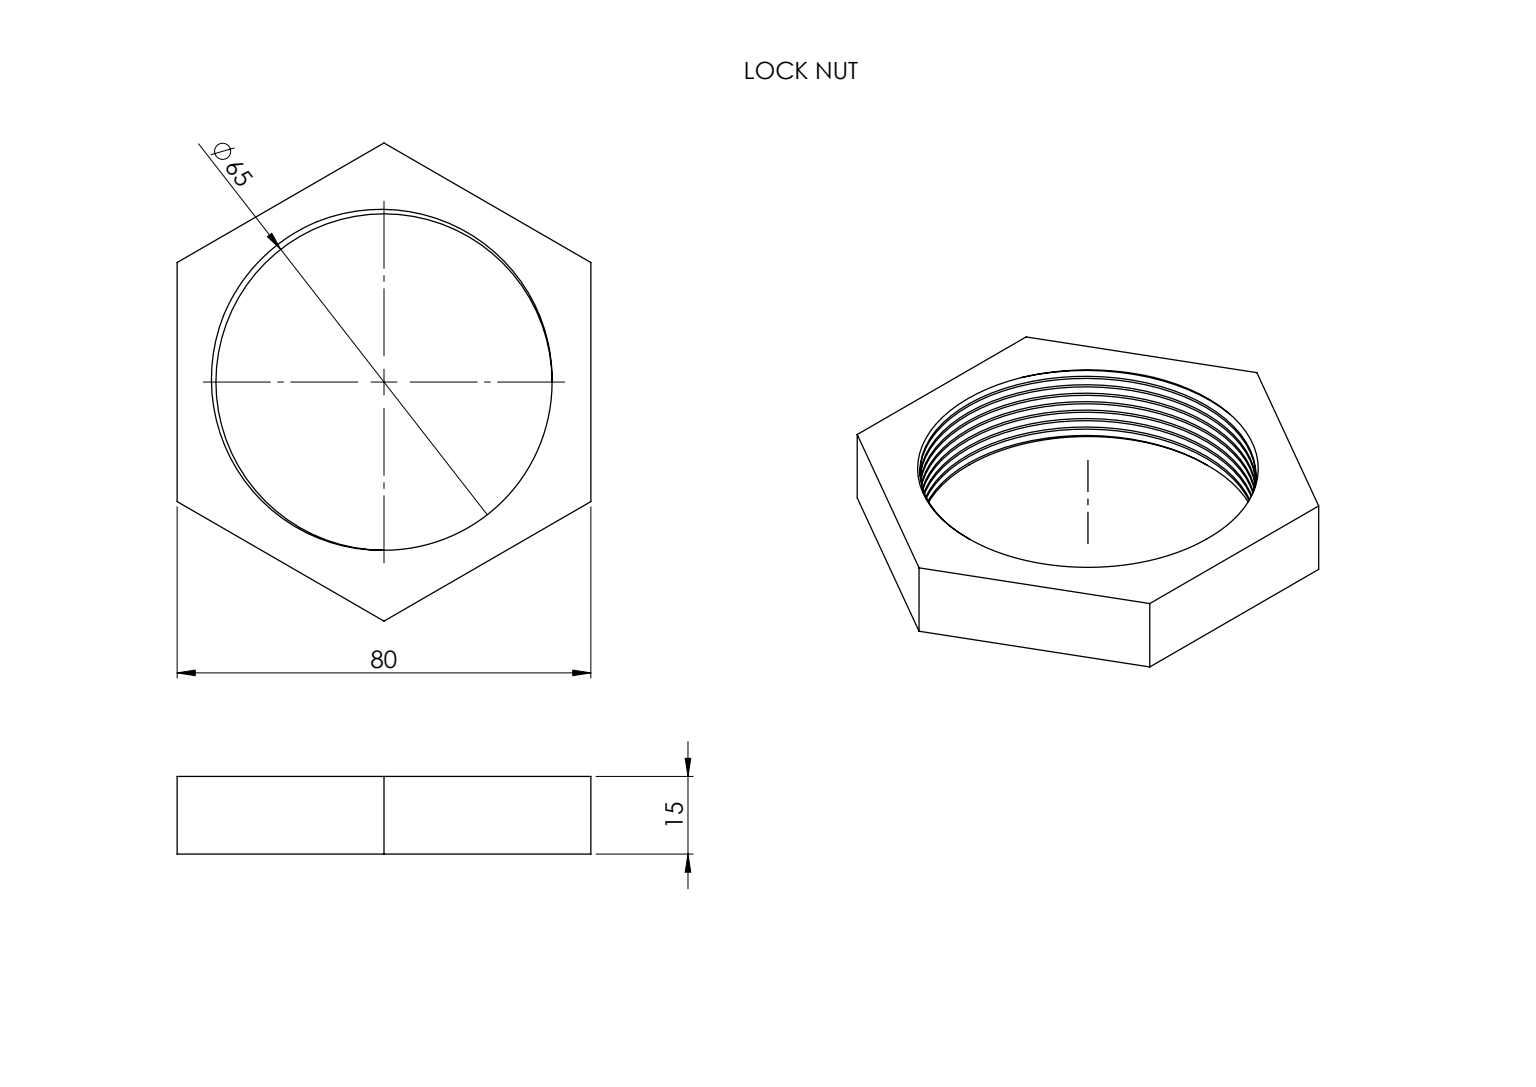
ISO-10303-21;
HEADER;
FILE_DESCRIPTION (('STEP AP214'),
    '1' );
FILE_NAME ('lock nut.step',
    '2026-10-02T18:08:48',
    ( '' ),
    ( '' ),
    'SwSTEP 2.0',
    'SolidWorks 2026',
    '' );
FILE_SCHEMA (( 'AUTOMOTIVE_DESIGN' ));
ENDSEC;

DATA;
#2=CARTESIAN_POINT ( 'NONE',  ( 20.75514604977249178, 32.07500000273117990, 28.56700777964553950 ) ) ;
#7=CARTESIAN_POINT ( 'NONE',  ( -32.50000000000000000, 22.50000000546238610, 0.000000000000000000 ) ) ;
#19=CARTESIAN_POINT ( 'NONE',  ( 10.37757302488624767, 61.72500000273119269, 31.93888565452638417 ) ) ;
#24=CARTESIAN_POINT ( 'NONE',  ( -10.04305231718579172, 66.10000000546239107, -30.90933677959248982 ) ) ;
#26=LINE ( 'NONE', #5703, #33612 ) ;
#29=CARTESIAN_POINT ( 'NONE',  ( 20.75514604977249178, 76.07500000273118701, 28.56700777964553950 ) ) ;
#34=CARTESIAN_POINT ( 'NONE',  ( 20.75514604977248467, 54.42500000273117422, -28.56700777964554305 ) ) ;
#35=CARTESIAN_POINT ( 'NONE',  ( 33.58253175000000113, 14.37500000273118950, -4.112674001490185761E-15 ) ) ;
#36=CARTESIAN_POINT ( 'NONE',  ( 10.37757302488624056, 4.775000002731191628, -31.93888565452638417 ) ) ;
#40=CARTESIAN_POINT ( 'NONE',  ( -26.29305231718578995, 76.70000000546238539, 19.10302069950538595 ) ) ;
#42=CARTESIAN_POINT ( 'NONE',  ( 1.353501352685244852, 52.00000000000004263, -32.52334280248234677 ) ) ;
#47=ORIENTED_EDGE ( 'NONE', *, *, #4310, .T. ) ;
#48=CARTESIAN_POINT ( 'NONE',  ( -33.58253175000000113, 53.27500000273117564, -10.91162601494193218 ) ) ;
#52=VERTEX_POINT ( 'NONE', #19751 ) ;
#53=CARTESIAN_POINT ( 'NONE',  ( -10.37757302488624411, 22.72500000273118559, -31.93888565452638417 ) ) ;
#64=B_SPLINE_CURVE_WITH_KNOTS ( 'NONE', 3,
 ( #12577, #7079, #6739, #22702, #12751, #9302, #25452, #17563, #30235, #33154 ),
 .UNSPECIFIED., .F., .F.,
 ( 4, 2, 2, 2, 4 ),
 ( 0.000000000000000000, 0.006590582801587737370, 0.01318116560317547474, 0.01977174840476321124, 0.02636233120635094948 ),
 .UNSPECIFIED. ) ;
#66=CARTESIAN_POINT ( 'NONE',  ( 1.093617666956751375E-13, 66.00000000546238255, -32.50000000000000711 ) ) ;
#68=CARTESIAN_POINT ( 'NONE',  ( -10.04305231718579172, 13.59999999999998721, -30.90933677959248982 ) ) ;
#74=CARTESIAN_POINT ( 'NONE',  ( -27.16883889988624290, 70.92500000273120975, -19.73931689729374028 ) ) ;
#76=CARTESIAN_POINT ( 'NONE',  ( -33.58253175000000113, 33.37500000273117706, 0.000000000000000000 ) ) ;
#83=CARTESIAN_POINT ( 'NONE',  ( -20.08610463437157989, 55.69999999999998863, -27.64615127144129758 ) ) ;
#88=CARTESIAN_POINT ( 'NONE',  ( 10.37757302488624767, 71.97500000273120691, 31.93888565452638417 ) ) ;
#93=CARTESIAN_POINT ( 'NONE',  ( 6.486482029760649416E-15, 43.62500000273116285, 35.31076352940723240 ) ) ;
#97=CARTESIAN_POINT ( 'NONE',  ( -20.08610463437157989, 4.200000005462371178, -27.64615127144129758 ) ) ;
#113=CARTESIAN_POINT ( 'NONE',  ( 27.16883889988623935, 52.57500000273117280, -19.73931689729374384 ) ) ;
#120=CARTESIAN_POINT ( 'NONE',  ( 6.486482029760649416E-15, 15.62500000273117884, 35.31076352940723240 ) ) ;
#126=CARTESIAN_POINT ( 'NONE',  ( 20.08610463437157279, 33.80000000546235839, -27.64615127144129758 ) ) ;
#131=CARTESIAN_POINT ( 'NONE',  ( -33.58253175000000113, 63.02500000273118985, -10.91162601494193218 ) ) ;
#133=ORIENTED_EDGE ( 'NONE', *, *, #14029, .F. ) ;
#137=CARTESIAN_POINT ( 'NONE',  ( -20.75514604977248112, 3.425000002731186655, 28.56700777964554661 ) ) ;
#147=CARTESIAN_POINT ( 'NONE',  ( 6.277390505771533514E-15, 20.49999999999999289, 34.17252228774368916 ) ) ;
#157=CARTESIAN_POINT ( 'NONE',  ( -6.410174973103736740, 66.99999999999995737, -32.88179426022560392 ) ) ;
#160=CARTESIAN_POINT ( 'NONE',  ( -33.58253175000000113, 33.02500000273118275, -10.91162601494193218 ) ) ;
#162=CARTESIAN_POINT ( 'NONE',  ( 12.90513655866702081, 52.00000000000000711, 31.00393344628893288 ) ) ;
#165=CARTESIAN_POINT ( 'NONE',  ( 20.08610463437158344, 53.20000000546237118, 27.64615127144129403 ) ) ;
#172=CARTESIAN_POINT ( 'NONE',  ( 10.37757302488624767, 25.97500000273118914, 31.93888565452638417 ) ) ;
#176=CARTESIAN_POINT ( 'NONE',  ( -20.08610463437156923, 14.80000000546238503, 27.64615127144130113 ) ) ;
#188=CARTESIAN_POINT ( 'NONE',  ( 10.37757302488624056, 60.52500000273118275, -31.93888565452638417 ) ) ;
#198=CARTESIAN_POINT ( 'NONE',  ( -33.58253175000000113, 73.27500000273118985, -10.91162601494193218 ) ) ;
#202=CARTESIAN_POINT ( 'NONE',  ( 27.16883889988623935, 52.32500000273120122, -19.73931689729374384 ) ) ;
#203=CARTESIAN_POINT ( 'NONE',  ( 33.58253175000000113, 16.37500000273119127, -4.112674001490185761E-15 ) ) ;
#204=CARTESIAN_POINT ( 'NONE',  ( 33.58253175000000113, 6.475000002731178483, -10.91162601494193751 ) ) ;
#208=CARTESIAN_POINT ( 'NONE',  ( -26.29305231718579350, 76.30000000546237970, -19.10302069950537884 ) ) ;
#209=CARTESIAN_POINT ( 'NONE',  ( 33.29860495311163504, 51.99999999999997868, -1.751800823569056309 ) ) ;
#217=CARTESIAN_POINT ( 'NONE',  ( 27.16883889988623935, 46.57500000273119412, -19.73931689729374384 ) ) ;
#221=CARTESIAN_POINT ( 'NONE',  ( -33.58253175000000113, 25.22500000273119625, 10.91162601494193929 ) ) ;
#225=FACE_OUTER_BOUND ( 'NONE', #13152, .T. ) ;
#240=CARTESIAN_POINT ( 'NONE',  ( 32.50000000000000000, 19.00000000000000355, -3.980102097228898626E-15 ) ) ;
#247=CARTESIAN_POINT ( 'NONE',  ( 33.58253175000000113, 76.12500000273118417, -4.112674001490185761E-15 ) ) ;
#248=CARTESIAN_POINT ( 'NONE',  ( 27.16883889988623935, 38.57500000273118701, -19.73931689729374384 ) ) ;
#254=CARTESIAN_POINT ( 'NONE',  ( -10.04305231718578462, 56.39999999999999147, 30.90933677959249337 ) ) ;
#258=ORIENTED_EDGE ( 'NONE', *, *, #24258, .F. ) ;
#259=CARTESIAN_POINT ( 'NONE',  ( 10.37757302488624056, 70.77500000273118985, -31.93888565452638417 ) ) ;
#264=CARTESIAN_POINT ( 'NONE',  ( 10.37757302488624767, 45.72500000273120691, 31.93888565452638417 ) ) ;
#269=CARTESIAN_POINT ( 'NONE',  ( 10.04305231718578817, 5.900000005462382902, -30.90933677959249337 ) ) ;
#288=CARTESIAN_POINT ( 'NONE',  ( 27.16883889988623935, 56.57500000273117990, -19.73931689729374384 ) ) ;
#295=CARTESIAN_POINT ( 'NONE',  ( -26.29305231718578995, 76.20000000000000284, 19.10302069950538595 ) ) ;
#296=CARTESIAN_POINT ( 'NONE',  ( -33.58253175000000113, 15.22500000273119447, 10.91162601494193929 ) ) ;
#300=CARTESIAN_POINT ( 'NONE',  ( -2.092463501923844636E-15, 36.00000000546238255, -34.17252228774368916 ) ) ;
#305=CARTESIAN_POINT ( 'NONE',  ( 27.16883889988623935, 62.32500000273120833, -19.73931689729374384 ) ) ;
#309=CARTESIAN_POINT ( 'NONE',  ( 10.37757302488624767, 3.725000002731182480, 31.93888565452638417 ) ) ;
#320=CARTESIAN_POINT ( 'NONE',  ( -32.50000000000000000, 19.90000000000001279, -10.55989012756945478 ) ) ;
#324=CARTESIAN_POINT ( 'NONE',  ( -20.18813247507404185, 67.00000000000005684, 25.94218825114890237 ) ) ;
#332=CARTESIAN_POINT ( 'NONE',  ( 2.357955684373970406, 67.00000000000001421, -33.24972188832315823 ) ) ;
#334=CARTESIAN_POINT ( 'NONE',  ( -33.58253175000000113, 37.12500000273118417, 0.000000000000000000 ) ) ;
#340=CARTESIAN_POINT ( 'NONE',  ( 32.50000000000000000, 51.60000000546239107, -10.55989012756945833 ) ) ;
#342=SURFACE_STYLE_FILL_AREA ( #7570 ) ;
#347=CARTESIAN_POINT ( 'NONE',  ( -20.75514604977248112, 27.67500000273118133, 28.56700777964554661 ) ) ;
#352=CARTESIAN_POINT ( 'NONE',  ( -20.08610463437157989, 16.20000000546237118, -27.64615127144129758 ) ) ;
#362=CARTESIAN_POINT ( 'NONE',  ( -2.162160676586882350E-15, 52.62500000273117706, -35.31076352940722529 ) ) ;
#372=CARTESIAN_POINT ( 'NONE',  ( 27.16883889988623935, 68.57500000273118701, -19.73931689729374384 ) ) ;
#377=CARTESIAN_POINT ( 'NONE',  ( -33.58253175000000113, 55.22500000273117848, 10.91162601494193929 ) ) ;
#378=CARTESIAN_POINT ( 'NONE',  ( -20.75514604977248823, 15.07500000273116747, -28.56700777964554305 ) ) ;
#379=CARTESIAN_POINT ( 'NONE',  ( 33.58253175000000113, 4.475000002731183812, -10.91162601494193751 ) ) ;
#384=CARTESIAN_POINT ( 'NONE',  ( -2.092463501923844636E-15, 74.00000000546236834, -34.17252228774368916 ) ) ;
#391=CARTESIAN_POINT ( 'NONE',  ( 6.486482029760649416E-15, 47.87500000273117706, 35.31076352940723240 ) ) ;
#396=CARTESIAN_POINT ( 'NONE',  ( -33.58253175000000113, 19.22500000273118204, 10.91162601494193929 ) ) ;
#406=CARTESIAN_POINT ( 'NONE',  ( -1.053607264507113999E-13, 64.50000000000000000, 32.50000000000000711 ) ) ;
#408=CARTESIAN_POINT ( 'NONE',  ( -1.137977401836464321E-14, 52.00000000000000711, 46.18802153517007270 ) ) ;
#411=CARTESIAN_POINT ( 'NONE',  ( -10.04305231718578462, 16.40000000000001279, 30.90933677959249337 ) ) ;
#417=CARTESIAN_POINT ( 'NONE',  ( -20.75514604977248112, 71.42500000273119554, 28.56700777964554661 ) ) ;
#418=CARTESIAN_POINT ( 'NONE',  ( 33.58253175000000113, 36.37500000273118417, -4.112674001490185761E-15 ) ) ;
#424=CARTESIAN_POINT ( 'NONE',  ( 20.08610463437157279, 51.29999999999997584, -27.64615127144129758 ) ) ;
#431=CARTESIAN_POINT ( 'NONE',  ( -33.58253175000000113, 67.37500000273121259, 0.000000000000000000 ) ) ;
#436=CARTESIAN_POINT ( 'NONE',  ( -20.75514604977248823, 38.82500000273120122, -28.56700777964554305 ) ) ;
#456=CARTESIAN_POINT ( 'NONE',  ( -5.147494310547430452, 54.05125428700921475, -32.49999999999999289 ) ) ;
#460=CARTESIAN_POINT ( 'NONE',  ( -2.162160676586881955E-15, 56.87500000273117706, -35.31076352940723240 ) ) ;
#466=CARTESIAN_POINT ( 'NONE',  ( 26.29305231718579350, 74.80000000000002558, 19.10302069950537529 ) ) ;
#467=CARTESIAN_POINT ( 'NONE',  ( 20.75514604977248467, 6.425000002731192872, -28.56700777964554305 ) ) ;
#475=CARTESIAN_POINT ( 'NONE',  ( -10.37757302488624411, 60.72500000273119269, -31.93888565452638417 ) ) ;
#479=CARTESIAN_POINT ( 'NONE',  ( 27.16883889988623935, 2.325000002731183901, -19.73931689729374384 ) ) ;
#490=CARTESIAN_POINT ( 'NONE',  ( 32.50000000000000000, 25.09999999999999432, -10.55989012756945833 ) ) ;
#494=CARTESIAN_POINT ( 'NONE',  ( -31.53731130704430541, 66.99999999999997158, -11.55439184653567253 ) ) ;
#501=DIRECTION ( 'NONE',  ( -0.8660254037844385966, 0.000000000000000000, 0.5000000000000000000 ) ) ;
#502=CARTESIAN_POINT ( 'NONE',  ( -4.374313548017133790, 52.00000000000000000, 33.03144926559792083 ) ) ;
#503=CARTESIAN_POINT ( 'NONE',  ( -33.58253175000000113, 27.02500000273119696, -10.91162601494193218 ) ) ;
#504=CARTESIAN_POINT ( 'NONE',  ( 10.04305231718578817, 65.40000000000000568, -30.90933677959249337 ) ) ;
#509=CARTESIAN_POINT ( 'NONE',  ( 32.50000000000000000, 55.60000000546238397, -10.55989012756945833 ) ) ;
#518=CARTESIAN_POINT ( 'NONE',  ( -20.08610463437157989, 18.20000000546239605, -27.64615127144129758 ) ) ;
#528=CARTESIAN_POINT ( 'NONE',  ( -10.37757302488623701, 57.52500000273118275, 31.93888565452638417 ) ) ;
#537=CARTESIAN_POINT ( 'NONE',  ( -33.58253175000000113, 67.47500000273117848, 10.91162601494193929 ) ) ;
#541=CARTESIAN_POINT ( 'NONE',  ( 10.37757302488624056, 52.52500000273117564, -31.93888565452638417 ) ) ;
#542=CARTESIAN_POINT ( 'NONE',  ( -20.75514604977248112, 11.67500000273118843, 28.56700777964554661 ) ) ;
#543=CARTESIAN_POINT ( 'NONE',  ( 6.486482029760649416E-15, 5.875000002731183280, 35.31076352940723240 ) ) ;
#548=CARTESIAN_POINT ( 'NONE',  ( -20.08610463437156923, 72.80000000546239391, 27.64615127144130113 ) ) ;
#551=( BOUNDED_CURVE ( )  B_SPLINE_CURVE ( 2, ( #8336, #3034, #11096, #13507, #32180, #11259, #29937, #3529, #27205, #21735, #3205, #16579, #13673 ),
 .UNSPECIFIED., .F., .T. ) 
 B_SPLINE_CURVE_WITH_KNOTS ( ( 3, 2, 2, 2, 2, 2, 3 ),
 ( 0.2628205128205128305, 0.2641025641025641080, 0.2666666666666666630, 0.2692307692307692180, 0.2717948717948717730, 0.2743589743589743835, 0.2756410256410256610 ),
 .UNSPECIFIED. ) 
 CURVE ( )  GEOMETRIC_REPRESENTATION_ITEM ( )  RATIONAL_B_SPLINE_CURVE ( ( 0.9755282581475768211, 0.9755282581475768211, 1.000000000000000000, 0.9510565162951535312, 1.000000000000000000, 0.9510565162951535312, 1.000000000000000000, 0.9510565162951535312, 1.000000000000000000, 0.9510565162951535312, 1.000000000000000000, 0.9755282581475768211, 0.9755282581475768211 ) ) 
 REPRESENTATION_ITEM ( '' )  );
#557=CARTESIAN_POINT ( 'NONE',  ( 10.37757302488624056, 44.77500000273119696, -31.93888565452638417 ) ) ;
#562=CARTESIAN_POINT ( 'NONE',  ( 27.16883889988623935, 16.32500000273116925, -19.73931689729374384 ) ) ;
#576=CARTESIAN_POINT ( 'NONE',  ( 32.50000000000000000, 7.099999999999993427, -10.55989012756945833 ) ) ;
#582=CARTESIAN_POINT ( 'NONE',  ( 33.58253175000000823, 76.02500000273118985, 10.91162601494192863 ) ) ;
#583=CARTESIAN_POINT ( 'NONE',  ( 10.37757302488624056, 30.77500000273118630, -31.93888565452638417 ) ) ;
#588=CARTESIAN_POINT ( 'NONE',  ( 32.50000000000000711, 52.89999999999999147, 10.55989012756945122 ) ) ;
#593=CARTESIAN_POINT ( 'NONE',  ( 6.486482029760649416E-15, 69.87500000273121259, 35.31076352940723240 ) ) ;
#598=CARTESIAN_POINT ( 'NONE',  ( -10.37757302488623701, 39.52500000273119696, 31.93888565452638417 ) ) ;
#620=CARTESIAN_POINT ( 'NONE',  ( -10.04305231718578462, 54.90000000546239534, 30.90933677959249337 ) ) ;
#624=CARTESIAN_POINT ( 'NONE',  ( -20.75514604977248112, 53.67500000273119554, 28.56700777964554661 ) ) ;
#630=CARTESIAN_POINT ( 'NONE',  ( 20.08610463437157279, 75.30000000000001137, -27.64615127144129758 ) ) ;
#631=CARTESIAN_POINT ( 'NONE',  ( -20.75514604977248112, 9.425000002731184878, 28.56700777964554661 ) ) ;
#633=B_SPLINE_CURVE_WITH_KNOTS ( 'NONE', 3,
 ( #5996, #16472, #16149, #29654, #14063, #13570, #10819, #16643, #26602, #24033, #24364, #502, #10987, #21459, #995, #834, #21793, #24526, #31739, #11480, #2925, #19384, #5497, #26926, #5834, #29160, #15976, #26433, #13395, #5667, #31902, #8397, #29333, #26769, #3260, #4261, #16811, #4092, #27601, #14735, #27267, #32571, #20059, #6666 ),
 .UNSPECIFIED., .F., .F.,
 ( 4, 2, 2, 2, 2, 2, 2, 2, 2, 2, 2, 2, 2, 2, 2, 2, 2, 2, 2, 2, 2, 4 ),
 ( 0.000000000000000000, 0.004064997385822698324, 0.008129994771645396648, 0.01219499215746809584, 0.01422749085037944457, 0.01625998954329079330, 0.02032498692911348381, 0.02235748562202483428, 0.02438998431493618127, 0.02845498170075888567, 0.03251997908658158659, 0.03455247777949293359, 0.03658497647240428752, 0.04064997385822698150, 0.04471497124404968243, 0.04877996862987238336, 0.05081246732278373035, 0.05284496601569507734, 0.05690996340151777827, 0.05894246209442912526, 0.06097496078734047226, 0.06503995817316317318 ),
 .UNSPECIFIED. ) ;
#635=CARTESIAN_POINT ( 'NONE',  ( -32.50000000000000000, 66.10000000000000853, 10.55989012756946366 ) ) ;
#640=CARTESIAN_POINT ( 'NONE',  ( -10.37757302488624411, 56.72500000273118559, -31.93888565452638417 ) ) ;
#656=CARTESIAN_POINT ( 'NONE',  ( 32.50000000000000711, 24.90000000000000213, 10.55989012756945122 ) ) ;
#668=CARTESIAN_POINT ( 'NONE',  ( -10.37757302488623701, 25.52500000273118275, 31.93888565452638417 ) ) ;
#669=CARTESIAN_POINT ( 'NONE',  ( 32.50000000000000711, 56.90000000000000568, 10.55989012756945122 ) ) ;
#670=CARTESIAN_POINT ( 'NONE',  ( 32.50000000000000711, 61.40000000546236691, 10.55989012756945122 ) ) ;
#673=CARTESIAN_POINT ( 'NONE',  ( 6.277390505771533514E-15, 49.00000000546238965, 34.17252228774368916 ) ) ;
#679=VERTEX_POINT ( 'NONE', #27771 ) ;
#681=CARTESIAN_POINT ( 'NONE',  ( 27.16883889988623935, 74.32500000273118701, -19.73931689729374384 ) ) ;
#686=CARTESIAN_POINT ( 'NONE',  ( -26.29305231718579350, 16.30000000546237615, -19.10302069950537884 ) ) ;
#704=CARTESIAN_POINT ( 'NONE',  ( 33.58253175000000113, 70.37500000273121259, -4.112674001490185761E-15 ) ) ;
#709=CARTESIAN_POINT ( 'NONE',  ( 27.16883889988624290, 47.92500000273118843, 19.73931689729373673 ) ) ;
#710=CARTESIAN_POINT ( 'NONE',  ( 33.58253175000000113, 12.37500000273118772, -4.112674001490185761E-15 ) ) ;
#711=CARTESIAN_POINT ( 'NONE',  ( 10.37757302488624767, 59.97500000273119269, 31.93888565452638417 ) ) ;
#715=CARTESIAN_POINT ( 'NONE',  ( -10.04305231718578462, 76.90000000546235981, 30.90933677959249337 ) ) ;
#722=CARTESIAN_POINT ( 'NONE',  ( 27.16883889988624290, 46.17500000273118133, 19.73931689729373673 ) ) ;
#727=CARTESIAN_POINT ( 'NONE',  ( 27.16883889988623935, 18.32500000273119767, -19.73931689729374384 ) ) ;
#742=CARTESIAN_POINT ( 'NONE',  ( 6.277390505771533514E-15, 12.49999999999999645, 34.17252228774368916 ) ) ;
#748=CARTESIAN_POINT ( 'NONE',  ( 20.75514604977248467, 64.42500000273116711, -28.56700777964554305 ) ) ;
#749=CARTESIAN_POINT ( 'NONE',  ( -20.75514604977248823, 27.07500000273119412, -28.56700777964554305 ) ) ;
#751=CARTESIAN_POINT ( 'NONE',  ( 33.58253175000000113, 18.47500000273117848, -10.91162601494193751 ) ) ;
#761=CARTESIAN_POINT ( 'NONE',  ( -26.29305231718579350, 53.79999999999999716, -19.10302069950537884 ) ) ;
#765=EDGE_CURVE ( 'NONE', #2905, #6717, #4427, .T. ) ;
#767=CARTESIAN_POINT ( 'NONE',  ( -27.16883889988623935, 69.57500000273118701, 19.73931689729374739 ) ) ;
#772=CARTESIAN_POINT ( 'NONE',  ( 33.58253175000000113, 38.12500000273118417, -4.112674001490185761E-15 ) ) ;
#776=CARTESIAN_POINT ( 'NONE',  ( 27.16883889988623935, 66.57500000273118701, -19.73931689729374384 ) ) ;
#788=CARTESIAN_POINT ( 'NONE',  ( 26.29305231718578995, 53.70000000546236407, -19.10302069950538240 ) ) ;
#789=CARTESIAN_POINT ( 'NONE',  ( -10.04305231718579172, 54.10000000546237686, -30.90933677959248982 ) ) ;
#793=CARTESIAN_POINT ( 'NONE',  ( 27.16883889988624290, 50.17500000273118843, 19.73931689729373673 ) ) ;
#800=CARTESIAN_POINT ( 'NONE',  ( -20.08610463437156923, 74.30000000000001137, 27.64615127144130113 ) ) ;
#801=CARTESIAN_POINT ( 'NONE',  ( -33.58253175000000113, 11.22500000273118559, 10.91162601494193929 ) ) ;
#810=EDGE_LOOP ( 'NONE', ( #13911, #21012, #6429, #7622 ) ) ;
#811=CARTESIAN_POINT ( 'NONE',  ( -27.16883889988624290, 58.92500000273119554, -19.73931689729374028 ) ) ;
#812=EDGE_LOOP ( 'NONE', ( #32829, #8494, #29549, #33668 ) ) ;
#824=CARTESIAN_POINT ( 'NONE',  ( 10.04305231718578817, 25.39999999999999147, -30.90933677959249337 ) ) ;
#833=DIRECTION ( 'NONE',  ( 0.000000000000000000, 1.000000000000000000, 0.000000000000000000 ) ) ;
#834=CARTESIAN_POINT ( 'NONE',  ( -9.638965394428050004, 52.00000000000000000, 31.78062433674932308 ) ) ;
#835=CARTESIAN_POINT ( 'NONE',  ( -27.16883889988624290, 26.92500000273119554, -19.73931689729374028 ) ) ;
#836=CARTESIAN_POINT ( 'NONE',  ( -20.08610463437156923, 56.80000000546240102, 27.64615127144130113 ) ) ;
#840=CARTESIAN_POINT ( 'NONE',  ( 10.04305231718579705, 49.10000000546236976, 30.90933677959248982 ) ) ;
#843=( BOUNDED_CURVE ( )  B_SPLINE_CURVE ( 2, ( #8736, #29835, #998, #836, #5669, #11157, #16474, #18887, #11482, #8902, #19386, #16151, #24366 ),
 .UNSPECIFIED., .F., .T. ) 
 B_SPLINE_CURVE_WITH_KNOTS ( ( 3, 2, 2, 2, 2, 2, 3 ),
 ( 0.2756410256410256610, 0.2769230769230769384, 0.2794871794871794934, 0.2820512820512820484, 0.2846153846153846034, 0.2871794871794871584, 0.2884615384615384914 ),
 .UNSPECIFIED. ) 
 CURVE ( )  GEOMETRIC_REPRESENTATION_ITEM ( )  RATIONAL_B_SPLINE_CURVE ( ( 0.9755282581475768211, 0.9755282581475768211, 1.000000000000000000, 0.9510565162951535312, 1.000000000000000000, 0.9510565162951535312, 1.000000000000000000, 0.9510565162951535312, 1.000000000000000000, 0.9510565162951535312, 1.000000000000000000, 0.9755282581475762660, 0.9755282581475768211 ) ) 
 REPRESENTATION_ITEM ( '' )  );
#847=CARTESIAN_POINT ( 'NONE',  ( -10.37757302488624411, 74.72500000273117848, -31.93888565452638417 ) ) ;
#853=CARTESIAN_POINT ( 'NONE',  ( -26.29305231718578995, 14.70000000546238539, 19.10302069950538595 ) ) ;
#870=CARTESIAN_POINT ( 'NONE',  ( -33.58253175000000113, 71.47500000273119269, 10.91162601494193929 ) ) ;
#876=CARTESIAN_POINT ( 'NONE',  ( 33.58253175000000113, 50.22500000273118559, -10.91162601494193751 ) ) ;
#877=CARTESIAN_POINT ( 'NONE',  ( 27.16883889988624290, 10.17500000273117955, 19.73931689729373673 ) ) ;
#878=CARTESIAN_POINT ( 'NONE',  ( 33.58253175000000823, 62.27500000273118985, 10.91162601494192685 ) ) ;
#882=CARTESIAN_POINT ( 'NONE',  ( -32.50000000000000000, 66.60000000546236265, 10.55989012756946366 ) ) ;
#889=CARTESIAN_POINT ( 'NONE',  ( -27.16883889988623935, 49.57500000273120122, 19.73931689729374739 ) ) ;
#894=CARTESIAN_POINT ( 'NONE',  ( -10.37757302488623701, 19.52500000273120406, 31.93888565452638417 ) ) ;
#906=CARTESIAN_POINT ( 'NONE',  ( 32.50000000000000000, 65.50000000546239676, -3.980102097228898626E-15 ) ) ;
#909=CARTESIAN_POINT ( 'NONE',  ( 20.08610463437157279, 13.29999999999998650, -27.64615127144129758 ) ) ;
#915=CARTESIAN_POINT ( 'NONE',  ( -33.58253175000000113, 69.22500000273117848, 10.91162601494193929 ) ) ;
#916=CARTESIAN_POINT ( 'NONE',  ( 10.37757302488624767, 31.97500000273119269, 31.93888565452638417 ) ) ;
#917=CARTESIAN_POINT ( 'NONE',  ( -27.16883889988623935, 19.57500000273119767, 19.73931689729374739 ) ) ;
#923=CARTESIAN_POINT ( 'NONE',  ( 26.29305231718579350, 50.79999999999999716, 19.10302069950537529 ) ) ;
#927=VERTEX_POINT ( 'NONE', #25192 ) ;
#928=CARTESIAN_POINT ( 'NONE',  ( 20.75514604977249178, 68.07500000273118701, 28.56700777964553950 ) ) ;
#934=CARTESIAN_POINT ( 'NONE',  ( 20.75514604977248467, 34.42500000273117422, -28.56700777964554305 ) ) ;
#949=EDGE_CURVE ( 'NONE', #9615, #21053, #27598, .T. ) ;
#950=CARTESIAN_POINT ( 'NONE',  ( -26.29305231718579350, 54.30000000546237970, -19.10302069950537884 ) ) ;
#954=CARTESIAN_POINT ( 'NONE',  ( 27.16883889988624290, 46.17500000273118133, 19.73931689729373673 ) ) ;
#960=CARTESIAN_POINT ( 'NONE',  ( 32.50000000000000000, 68.99999999999998579, -3.980102097228898626E-15 ) ) ;
#961=CARTESIAN_POINT ( 'NONE',  ( -33.58253175000000113, 11.12500000273118594, 0.000000000000000000 ) ) ;
#970=CARTESIAN_POINT ( 'NONE',  ( 10.37757302488624056, 58.52500000273118275, -31.93888565452638417 ) ) ;
#971=CARTESIAN_POINT ( 'NONE',  ( -33.58253175000000113, 29.27500000273118630, -10.91162601494193218 ) ) ;
#995=CARTESIAN_POINT ( 'NONE',  ( -8.342407680043393725, 52.00000000000000711, 32.16802901964487660 ) ) ;
#997=CARTESIAN_POINT ( 'NONE',  ( -33.58253175000000113, 29.22500000273118914, 10.91162601494193929 ) ) ;
#998=CARTESIAN_POINT ( 'NONE',  ( -10.04305231718578462, 56.90000000546240244, 30.90933677959249337 ) ) ;
#999=CARTESIAN_POINT ( 'NONE',  ( 5.147494310547426899, 61.94874572391552192, -32.50000000000000000 ) ) ;
#1002=CARTESIAN_POINT ( 'NONE',  ( 32.50000000000000000, 49.50000000546238255, -3.980102097228898626E-15 ) ) ;
#1006=CARTESIAN_POINT ( 'NONE',  ( 27.16883889988623935, 76.32500000273120122, -19.73931689729374384 ) ) ;
#1011=CARTESIAN_POINT ( 'NONE',  ( -32.50000000000000000, 10.40000000546237935, -10.55989012756945478 ) ) ;
#1018=CARTESIAN_POINT ( 'NONE',  ( -10.04305231718579172, 62.10000000546238397, -30.90933677959248982 ) ) ;
#1020=SURFACE_STYLE_USAGE ( .BOTH. , #4120 ) ;
#1021=CARTESIAN_POINT ( 'NONE',  ( 26.29305231718578995, 37.19999999999999574, -19.10302069950538240 ) ) ;
#1031=CARTESIAN_POINT ( 'NONE',  ( 20.75514604977249178, 66.07500000273118701, 28.56700777964553950 ) ) ;
#1036=CARTESIAN_POINT ( 'NONE',  ( 33.58253175000000823, 50.02500000273118985, 10.91162601494192863 ) ) ;
#1037=CARTESIAN_POINT ( 'NONE',  ( 20.75514604977249178, 14.07500000273119944, 28.56700777964553950 ) ) ;
#1038=CARTESIAN_POINT ( 'NONE',  ( 33.58253175000000113, 60.47500000273118559, -10.91162601494193574 ) ) ;
#1042=CARTESIAN_POINT ( 'NONE',  ( 26.29305231718579350, 67.30000000546236549, 19.10302069950537529 ) ) ;
#1048=CARTESIAN_POINT ( 'NONE',  ( 10.37757302488624767, 41.97500000273117138, 31.93888565452638417 ) ) ;
#1050=CARTESIAN_POINT ( 'NONE',  ( 6.277390505771533514E-15, 33.00000000546238255, 34.17252228774368916 ) ) ;
#1051=ORIENTED_EDGE ( 'NONE', *, *, #15985, .F. ) ;
#1052=CARTESIAN_POINT ( 'NONE',  ( 10.37757302488624767, 17.72500000273118204, 31.93888565452638417 ) ) ;
#1070=CARTESIAN_POINT ( 'NONE',  ( -20.08610463437157989, 11.70000000000000995, -27.64615127144129758 ) ) ;
#1076=CARTESIAN_POINT ( 'NONE',  ( -27.16883889988624290, 66.92500000273119554, -19.73931689729374028 ) ) ;
#1077=CARTESIAN_POINT ( 'NONE',  ( 27.16883889988624290, 32.17500000273120264, 19.73931689729373673 ) ) ;
#1078=CARTESIAN_POINT ( 'NONE',  ( -10.37757302488624411, 14.97500000273120691, -31.93888565452638417 ) ) ;
#1084=CARTESIAN_POINT ( 'NONE',  ( 10.04305231718578817, 49.39999999999998437, -30.90933677959249337 ) ) ;
#1089=CARTESIAN_POINT ( 'NONE',  ( -33.58253175000000113, 69.27500000273116143, -10.91162601494193218 ) ) ;
#1094=CARTESIAN_POINT ( 'NONE',  ( -20.75514604977248112, 39.42500000273118843, 28.56700777964554661 ) ) ;
#1114=CARTESIAN_POINT ( 'NONE',  ( -2.162160676586881955E-15, 50.87500000273119838, -35.31076352940723240 ) ) ;
#1118=CARTESIAN_POINT ( 'NONE',  ( 0.000000000000000000, 52.00000000000000711, 0.000000000000000000 ) ) ;
#1120=CARTESIAN_POINT ( 'NONE',  ( 32.50000000000000711, 68.90000000000001990, 10.55989012756945122 ) ) ;
#1121=CARTESIAN_POINT ( 'NONE',  ( -10.37757302488623701, 7.525000002731194293, 31.93888565452638417 ) ) ;
#1131=CARTESIAN_POINT ( 'NONE',  ( 27.16883889988624290, 53.92500000273118843, 19.73931689729373673 ) ) ;
#1132=CARTESIAN_POINT ( 'NONE',  ( -27.16883889988624290, 27.17500000273119554, -19.73931689729374028 ) ) ;
#1148=CARTESIAN_POINT ( 'NONE',  ( -33.58253175000000113, 57.02500000273118275, -10.91162601494193041 ) ) ;
#1162=CARTESIAN_POINT ( 'NONE',  ( 30.93003301939247152, 66.99999999999998579, -10.64619209630829211 ) ) ;
#1164=CARTESIAN_POINT ( 'NONE',  ( 33.58253175000000113, 26.22500000273119625, -10.91162601494193751 ) ) ;
#1172=CARTESIAN_POINT ( 'NONE',  ( 10.04305231718579705, 51.10000000546236976, 30.90933677959248982 ) ) ;
#1173=CARTESIAN_POINT ( 'NONE',  ( -1.778240108872766143E-15, 58.00000000546237544, -32.49999999999999289 ) ) ;
#1175=ORIENTED_EDGE ( 'NONE', *, *, #13369, .F. ) ;
#1176=CARTESIAN_POINT ( 'NONE',  ( 33.58253175000000113, 72.22500000273119269, -10.91162601494193751 ) ) ;
#1181=CARTESIAN_POINT ( 'NONE',  ( -10.04305231718579172, 10.10000000546239285, -30.90933677959248982 ) ) ;
#1191=CARTESIAN_POINT ( 'NONE',  ( -20.08610463437156923, 34.29999999999998295, 27.64615127144130113 ) ) ;
#1203=CARTESIAN_POINT ( 'NONE',  ( 10.37757302488624767, 49.72500000273117848, 31.93888565452638417 ) ) ;
#1204=CARTESIAN_POINT ( 'NONE',  ( -27.16883889988623935, 13.57500000273119412, 19.73931689729374739 ) ) ;
#1205=CARTESIAN_POINT ( 'NONE',  ( -27.16883889988624290, 61.17500000273119554, -19.73931689729374028 ) ) ;
#1209=CARTESIAN_POINT ( 'NONE',  ( -32.50000000000000000, 68.50000000546239676, 0.000000000000000000 ) ) ;
#1214=ORIENTED_EDGE ( 'NONE', *, *, #29173, .F. ) ;
#1216=CARTESIAN_POINT ( 'NONE',  ( 33.58253175000000113, 44.47500000273119269, -10.91162601494193751 ) ) ;
#1218=CARTESIAN_POINT ( 'NONE',  ( -10.04305231718579172, 32.10000000546238397, -30.90933677959248982 ) ) ;
#1221=VERTEX_POINT ( 'NONE', #6926 ) ;
#1222=ORIENTED_EDGE ( 'NONE', *, *, #18466, .F. ) ;
#1234=CARTESIAN_POINT ( 'NONE',  ( 0.000000000000000000, 52.00000000000000711, 32.50000000000000000 ) ) ;
#1237=CARTESIAN_POINT ( 'NONE',  ( -26.29305231718578995, 56.20000000000001705, 19.10302069950538595 ) ) ;
#1239=CARTESIAN_POINT ( 'NONE',  ( 20.08610463437157279, 3.299999999999997602, -27.64615127144129758 ) ) ;
#1244=CARTESIAN_POINT ( 'NONE',  ( -33.58253175000000113, 67.22500000273117848, 10.91162601494193929 ) ) ;
#1245=CARTESIAN_POINT ( 'NONE',  ( 33.58253175000000823, 30.27500000273118630, 10.91162601494192863 ) ) ;
#1246=CARTESIAN_POINT ( 'NONE',  ( -33.58253175000000113, 15.37500000273118950, 0.000000000000000000 ) ) ;
#1252=CARTESIAN_POINT ( 'NONE',  ( 6.277390505771533514E-15, 46.50000000000001421, 34.17252228774368916 ) ) ;
#1258=CARTESIAN_POINT ( 'NONE',  ( 10.37757302488624767, 61.97500000273119269, 31.93888565452638417 ) ) ;
#1264=CARTESIAN_POINT ( 'NONE',  ( 6.486482029760649416E-15, 33.62500000273119127, 35.31076352940723240 ) ) ;
#1286=CARTESIAN_POINT ( 'NONE',  ( -20.75514604977248823, 51.07500000273116569, -28.56700777964554305 ) ) ;
#1291=CARTESIAN_POINT ( 'NONE',  ( -31.04172217648553556, 66.99999999999998579, -12.81397374188210136 ) ) ;
#1292=CARTESIAN_POINT ( 'NONE',  ( -20.08610463437157989, 65.69999999999998863, -27.64615127144129758 ) ) ;
#1297=CARTESIAN_POINT ( 'NONE',  ( -2.162160676586881955E-15, 78.87500000273118417, -35.31076352940723240 ) ) ;
#1303=CARTESIAN_POINT ( 'NONE',  ( -33.58253175000000113, 53.02500000273118985, -10.91162601494193218 ) ) ;
#1304=CARTESIAN_POINT ( 'NONE',  ( -20.75514604977248112, 25.67500000273118488, 28.56700777964554661 ) ) ;
#1318=CARTESIAN_POINT ( 'NONE',  ( -20.75514604977248823, 54.82500000273118701, -28.56700777964554305 ) ) ;
#1331=DIRECTION ( 'NONE',  ( 0.000000000000000000, 0.000000000000000000, 1.000000000000000000 ) ) ;
#1336=CARTESIAN_POINT ( 'NONE',  ( -33.58253175000000113, 21.02500000273117919, -10.91162601494193218 ) ) ;
#1341=CARTESIAN_POINT ( 'NONE',  ( 32.50000000000000000, 45.60000000546236265, -10.55989012756945833 ) ) ;
#1345=VERTEX_POINT ( 'NONE', #20504 ) ;
#1346=CARTESIAN_POINT ( 'NONE',  ( 33.58253175000000113, 76.22500000273119269, -10.91162601494193751 ) ) ;
#1352=CARTESIAN_POINT ( 'NONE',  ( 6.277390505771533514E-15, 13.00000000546238255, 34.17252228774368916 ) ) ;
#1364=CARTESIAN_POINT ( 'NONE',  ( -32.50000000000000000, 34.10000000000000142, 10.55989012756946366 ) ) ;
#1376=AXIS2_PLACEMENT_3D ( 'NONE', #6186, #27460, #21818 ) ;
#1379=CARTESIAN_POINT ( 'NONE',  ( -20.75514604977248112, 49.42500000273118133, 28.56700777964554661 ) ) ;
#1380=CARTESIAN_POINT ( 'NONE',  ( -33.58253175000000113, 1.375000002731191495, 0.000000000000000000 ) ) ;
#1381=CARTESIAN_POINT ( 'NONE',  ( 27.16883889988623935, 56.57500000273117990, -19.73931689729374384 ) ) ;
#1386=CARTESIAN_POINT ( 'NONE',  ( 20.08610463437157279, 69.80000000546240813, -27.64615127144129758 ) ) ;
#1394=CARTESIAN_POINT ( 'NONE',  ( -10.37757302488623701, 43.77500000273119696, 31.93888565452638417 ) ) ;
#1396=CARTESIAN_POINT ( 'NONE',  ( -32.50000000000000000, 32.60000000546237686, 10.55989012756946366 ) ) ;
#1399=ORIENTED_EDGE ( 'NONE', *, *, #21754, .T. ) ;
#1404=CARTESIAN_POINT ( 'NONE',  ( 20.75514604977248467, 66.42500000273119554, -28.56700777964554305 ) ) ;
#1412=CARTESIAN_POINT ( 'NONE',  ( -20.08610463437156923, 56.29999999999999716, 27.64615127144130113 ) ) ;
#1414=CARTESIAN_POINT ( 'NONE',  ( 32.50000000000000000, 5.099999999999998757, -10.55989012756945833 ) ) ;
#1415=ORIENTED_EDGE ( 'NONE', *, *, #27172, .T. ) ;
#1419=CARTESIAN_POINT ( 'NONE',  ( -20.75514604977248112, 69.42500000273116711, 28.56700777964554661 ) ) ;
#1420=CARTESIAN_POINT ( 'NONE',  ( -20.75514604977248823, 23.07500000273117635, -28.56700777964554305 ) ) ;
#1421=CARTESIAN_POINT ( 'NONE',  ( 33.58253175000000113, 16.47500000273118204, -10.91162601494193751 ) ) ;
#1426=CARTESIAN_POINT ( 'NONE',  ( -2.092463501923844636E-15, 45.49999999999998579, -34.17252228774368916 ) ) ;
#1431=CARTESIAN_POINT ( 'NONE',  ( -33.58253175000000113, 61.27500000273118985, -10.91162601494193218 ) ) ;
#1436=CARTESIAN_POINT ( 'NONE',  ( 27.16883889988624290, 29.92500000273119909, 19.73931689729373673 ) ) ;
#1460=CARTESIAN_POINT ( 'NONE',  ( 10.37757302488624767, 49.97500000273117848, 31.93888565452638417 ) ) ;
#1467=CARTESIAN_POINT ( 'NONE',  ( -20.08610463437157989, 69.69999999999997442, -27.64615127144129758 ) ) ;
#1473=CARTESIAN_POINT ( 'NONE',  ( -27.16883889988624290, 77.17500000273118133, -19.73931689729374028 ) ) ;
#1478=CARTESIAN_POINT ( 'NONE',  ( 27.16883889988624290, 47.92500000273118843, 19.73931689729373673 ) ) ;
#1479=CARTESIAN_POINT ( 'NONE',  ( 6.486482029760649416E-15, 21.87500000273118062, 35.31076352940723240 ) ) ;
#1480=ORIENTED_EDGE ( 'NONE', *, *, #24258, .T. ) ;
#1493=CARTESIAN_POINT ( 'NONE',  ( 33.58253175000000823, 54.02500000273118985, 10.91162601494192685 ) ) ;
#1507=CARTESIAN_POINT ( 'NONE',  ( 27.16883889988624290, 21.92500000273119198, 19.73931689729373673 ) ) ;
#1508=CARTESIAN_POINT ( 'NONE',  ( -40.00000000000000711, 52.00000000000000711, 23.09401076758504345 ) ) ;
#1512=CARTESIAN_POINT ( 'NONE',  ( 32.50000000000000000, 39.60000000546234844, -10.55989012756945833 ) ) ;
#1518=CARTESIAN_POINT ( 'NONE',  ( 27.16883889988624290, 65.92500000273119554, 19.73931689729373673 ) ) ;
#1525=CARTESIAN_POINT ( 'NONE',  ( 32.50000000000000000, 9.500000005462375441, -3.980102097228898626E-15 ) ) ;
#1534=CARTESIAN_POINT ( 'NONE',  ( -32.50000000000000000, 34.00000000000001421, 0.000000000000000000 ) ) ;
#1539=CARTESIAN_POINT ( 'NONE',  ( -1.778240108872766143E-15, 63.50000000000000000, -32.49999999999999289 ) ) ;
#1546=CARTESIAN_POINT ( 'NONE',  ( -20.75514604977248112, 43.42500000273117422, 28.56700777964554661 ) ) ;
#1547=CARTESIAN_POINT ( 'NONE',  ( -33.58253175000000113, 5.275000002731187188, -10.91162601494193218 ) ) ;
#1548=CARTESIAN_POINT ( 'NONE',  ( -20.75514604977248112, 57.67500000273118843, 28.56700777964554661 ) ) ;
#1552=CARTESIAN_POINT ( 'NONE',  ( -26.29305231718579350, 58.30000000546238681, -19.10302069950537884 ) ) ;
#1557=CARTESIAN_POINT ( 'NONE',  ( -33.58253175000000113, 41.47500000273117138, 10.91162601494193929 ) ) ;
#1560=CARTESIAN_POINT ( 'NONE',  ( -26.29305231718579350, 28.30000000546238681, -19.10302069950537884 ) ) ;
#1570=CARTESIAN_POINT ( 'NONE',  ( 27.16883889988624290, 65.92500000273119554, 19.73931689729373673 ) ) ;
#1580=CARTESIAN_POINT ( 'NONE',  ( 10.04305231718579705, 6.599999999999994316, 30.90933677959248982 ) ) ;
#1586=CARTESIAN_POINT ( 'NONE',  ( -27.16883889988623935, 63.32500000273120833, 19.73931689729374739 ) ) ;
#1587=CARTESIAN_POINT ( 'NONE',  ( -33.58253175000000113, 25.37500000273119838, 0.000000000000000000 ) ) ;
#1588=CARTESIAN_POINT ( 'NONE',  ( -27.16883889988623935, 11.57500000273119234, 19.73931689729374739 ) ) ;
#1592=CARTESIAN_POINT ( 'NONE',  ( 32.50000000000000711, 46.90000000000000568, 10.55989012756945122 ) ) ;
#1599=CARTESIAN_POINT ( 'NONE',  ( 27.16883889988624290, 58.17500000273119554, 19.73931689729373673 ) ) ;
#1604=CARTESIAN_POINT ( 'NONE',  ( -10.37757302488623701, 27.52500000273118275, 31.93888565452638417 ) ) ;
#1625=CARTESIAN_POINT ( 'NONE',  ( 20.75514604977249178, 40.07500000273118701, 28.56700777964553950 ) ) ;
#1630=CARTESIAN_POINT ( 'NONE',  ( 20.08610463437157279, 69.29999999999996874, -27.64615127144129758 ) ) ;
#1636=LINE ( 'NONE', #9362, #17269 ) ;
#1642=CARTESIAN_POINT ( 'NONE',  ( 20.75514604977248467, 50.42500000273118843, -28.56700777964554305 ) ) ;
#1643=CARTESIAN_POINT ( 'NONE',  ( 33.58253175000000113, 20.47500000273120335, -10.91162601494193751 ) ) ;
#1656=CARTESIAN_POINT ( 'NONE',  ( -31.04172217648553556, 66.99999999999998579, -12.81397374188210136 ) ) ;
#1667=CARTESIAN_POINT ( 'NONE',  ( -20.75514604977248823, 61.07500000273119412, -28.56700777964554305 ) ) ;
#1675=CARTESIAN_POINT ( 'NONE',  ( -33.58253175000000113, 21.12500000273119483, 0.000000000000000000 ) ) ;
#1677=CARTESIAN_POINT ( 'NONE',  ( -2.165007332552593587E-13, 52.50000000000000711, 32.50000000000000000 ) ) ;
#1680=CARTESIAN_POINT ( 'NONE',  ( 26.29305231718578995, 43.70000000546238539, -19.10302069950538240 ) ) ;
#1683=CARTESIAN_POINT ( 'NONE',  ( -10.37757302488623701, 65.77500000273118985, 31.93888565452638417 ) ) ;
#1687=CARTESIAN_POINT ( 'NONE',  ( -10.37757302488624411, 68.72500000273116427, -31.93888565452638417 ) ) ;
#1690=VERTEX_POINT ( 'NONE', #10366 ) ;
#1693=CARTESIAN_POINT ( 'NONE',  ( -2.162160676586881955E-15, 12.62500000273118772, -35.31076352940723240 ) ) ;
#1702=CARTESIAN_POINT ( 'NONE',  ( -10.04305231718578462, 36.39999999999999858, 30.90933677959249337 ) ) ;
#1706=CARTESIAN_POINT ( 'NONE',  ( 5.779280353836490358E-15, 62.50000000000000000, 32.49999999999999289 ) ) ;
#1716=CARTESIAN_POINT ( 'NONE',  ( 20.75514604977248467, 42.42500000273117422, -28.56700777964554305 ) ) ;
#1717=CARTESIAN_POINT ( 'NONE',  ( -10.37757302488624411, 6.975000002731198911, -31.93888565452638417 ) ) ;
#1718=CARTESIAN_POINT ( 'NONE',  ( -2.162160676586882350E-15, 52.87500000273119838, -35.31076352940722529 ) ) ;
#1721=CARTESIAN_POINT ( 'NONE',  ( -32.50000000000000000, 58.50000000546238965, 0.000000000000000000 ) ) ;
#1727=CARTESIAN_POINT ( 'NONE',  ( 6.486482029760649416E-15, 41.87500000273119127, 35.31076352940723240 ) ) ;
#1729=VERTEX_POINT ( 'NONE', #22178 ) ;
#1731=CARTESIAN_POINT ( 'NONE',  ( -20.08610463437156923, 32.80000000546237260, 27.64615127144130113 ) ) ;
#1736=( BOUNDED_CURVE ( )  B_SPLINE_CURVE ( 2, ( #33821, #10315, #4815, #31068, #18047, #4988, #13398, #669, #6161, #27100, #3427, #21959, #16645 ),
 .UNSPECIFIED., .F., .T. ) 
 B_SPLINE_CURVE_WITH_KNOTS ( ( 3, 2, 2, 2, 2, 2, 3 ),
 ( 0.2884615384615384914, 0.2897435897435897689, 0.2923076923076923239, 0.2948717948717948789, 0.2974358974358974339, 0.2999999999999999889, 0.3012820512820512664 ),
 .UNSPECIFIED. ) 
 CURVE ( )  GEOMETRIC_REPRESENTATION_ITEM ( )  RATIONAL_B_SPLINE_CURVE ( ( 0.9755282581475768211, 0.9755282581475772652, 1.000000000000000000, 0.9510565162951535312, 1.000000000000000000, 0.9510565162951535312, 1.000000000000000000, 0.9510565162951535312, 1.000000000000000000, 0.9510565162951535312, 1.000000000000000000, 0.9755282581475768211, 0.9755282581475768211 ) ) 
 REPRESENTATION_ITEM ( '' )  );
#1740=CARTESIAN_POINT ( 'NONE',  ( -10.37757302488624411, 64.72500000273119269, -31.93888565452638417 ) ) ;
#1749=DIRECTION ( 'NONE',  ( 0.8660254037844385966, 0.000000000000000000, 0.5000000000000000000 ) ) ;
#1750=CARTESIAN_POINT ( 'NONE',  ( -20.08610463437157989, 5.699999999999993960, -27.64615127144129758 ) ) ;
#1755=CARTESIAN_POINT ( 'NONE',  ( 33.58253175000000113, 60.12500000273117706, -4.112674001490185761E-15 ) ) ;
#1756=CARTESIAN_POINT ( 'NONE',  ( -33.58253175000000113, 21.37500000273119483, 0.000000000000000000 ) ) ;
#1757=CARTESIAN_POINT ( 'NONE',  ( -27.16883889988624290, 11.17500000273118133, -19.73931689729374028 ) ) ;
#1761=CARTESIAN_POINT ( 'NONE',  ( -27.16883889988624290, 2.925000002731187543, -19.73931689729374028 ) ) ;
#1763=CARTESIAN_POINT ( 'NONE',  ( -10.04305231718579172, 41.60000000000000853, -30.90933677959248982 ) ) ;
#1767=EDGE_LOOP ( 'NONE', ( #11128, #21845, #19685, #258 ) ) ;
#1768=CARTESIAN_POINT ( 'NONE',  ( 27.16883889988624290, 60.17500000273119554, 19.73931689729373673 ) ) ;
#1774=CARTESIAN_POINT ( 'NONE',  ( 10.37757302488624056, 28.52500000273118630, -31.93888565452638417 ) ) ;
#1799=CARTESIAN_POINT ( 'NONE',  ( 20.75514604977248467, 40.67500000273116711, -28.56700777964554305 ) ) ;
#1806=CARTESIAN_POINT ( 'NONE',  ( -10.04305231718578462, 60.39999999999999858, 30.90933677959249337 ) ) ;
#1811=CARTESIAN_POINT ( 'NONE',  ( 27.16883889988624290, 78.17500000273118133, 19.73931689729373673 ) ) ;
#1815=ORIENTED_EDGE ( 'NONE', *, *, #23644, .F. ) ;
#1816=CARTESIAN_POINT ( 'NONE',  ( 33.58253175000000113, 50.12500000273119127, -4.112674001490185761E-15 ) ) ;
#1817=CARTESIAN_POINT ( 'NONE',  ( -27.16883889988624290, 21.17500000273118843, -19.73931689729374028 ) ) ;
#1841=CARTESIAN_POINT ( 'NONE',  ( 20.75514604977248467, 60.67500000273118133, -28.56700777964554305 ) ) ;
#1848=CARTESIAN_POINT ( 'NONE',  ( 32.50000000000000000, 63.50000000546239676, -3.980102097228898626E-15 ) ) ;
#1850=CARTESIAN_POINT ( 'NONE',  ( 33.58253175000000113, 24.22500000273119625, -10.91162601494193751 ) ) ;
#1857=CARTESIAN_POINT ( 'NONE',  ( 10.04305231718579705, 39.10000000546236265, 30.90933677959248982 ) ) ;
#1862=CARTESIAN_POINT ( 'NONE',  ( -33.58253175000000113, 69.22500000273117848, 10.91162601494193929 ) ) ;
#1868=CARTESIAN_POINT ( 'NONE',  ( -33.58253175000000113, 11.12500000273118594, 0.000000000000000000 ) ) ;
#1870=CARTESIAN_POINT ( 'NONE',  ( 5.779280353836490358E-15, 66.50000000000000000, 32.49999999999999289 ) ) ;
#1878=CARTESIAN_POINT ( 'NONE',  ( -26.29305231718578995, 28.19999999999998863, 19.10302069950538595 ) ) ;
#1893=CARTESIAN_POINT ( 'NONE',  ( 20.75514604977248467, 38.42500000273118133, -28.56700777964554305 ) ) ;
#1894=CARTESIAN_POINT ( 'NONE',  ( 6.486482029760649416E-15, 5.875000002731183280, 35.31076352940723240 ) ) ;
#1895=CARTESIAN_POINT ( 'NONE',  ( -27.16883889988624290, 57.17500000273119554, -19.73931689729374028 ) ) ;
#1900=CARTESIAN_POINT ( 'NONE',  ( 6.277390505771533514E-15, 63.00000000546238255, 34.17252228774368916 ) ) ;
#1906=CARTESIAN_POINT ( 'NONE',  ( -27.16883889988623935, 37.57500000273118701, 19.73931689729374739 ) ) ;
#1910=CARTESIAN_POINT ( 'NONE',  ( -32.50000000000000000, 24.40000000546237047, -10.55989012756945478 ) ) ;
#1928=CARTESIAN_POINT ( 'NONE',  ( 0.000000000000000000, 52.00000000000000711, 0.000000000000000000 ) ) ;
#1929=CARTESIAN_POINT ( 'NONE',  ( 26.29305231718579350, 4.799999999999998934, 19.10302069950537529 ) ) ;
#1934=CARTESIAN_POINT ( 'NONE',  ( -10.37757302488624411, 62.72500000273119269, -31.93888565452638417 ) ) ;
#1935=CARTESIAN_POINT ( 'NONE',  ( -27.16883889988623935, 21.57500000273120122, 19.73931689729374739 ) ) ;
#1936=CARTESIAN_POINT ( 'NONE',  ( -33.58253175000000113, 13.47500000273118914, 10.91162601494193929 ) ) ;
#1943=CARTESIAN_POINT ( 'NONE',  ( -33.58253175000000113, 5.225000002731188253, 10.91162601494193929 ) ) ;
#1945=CARTESIAN_POINT ( 'NONE',  ( 10.04305231718579705, 40.60000000000000853, 30.90933677959248982 ) ) ;
#1951=CARTESIAN_POINT ( 'NONE',  ( 27.16883889988623935, 58.57500000273117990, -19.73931689729374384 ) ) ;
#1958=CARTESIAN_POINT ( 'NONE',  ( 6.486482029760649416E-15, 31.62500000273119483, 35.31076352940723240 ) ) ;
#1978=CARTESIAN_POINT ( 'NONE',  ( 20.75514604977248467, 78.42500000273116711, -28.56700777964554305 ) ) ;
#1979=CARTESIAN_POINT ( 'NONE',  ( -33.58253175000000113, 43.47500000273117138, 10.91162601494193929 ) ) ;
#1984=CARTESIAN_POINT ( 'NONE',  ( -26.29305231718578995, 58.20000000000001705, 19.10302069950538595 ) ) ;
#1989=CARTESIAN_POINT ( 'NONE',  ( -2.162160676586881955E-15, 76.87500000273115575, -35.31076352940723240 ) ) ;
#1994=CARTESIAN_POINT ( 'NONE',  ( -10.37757302488623701, 49.52500000273117564, 31.93888565452638417 ) ) ;
#1995=CARTESIAN_POINT ( 'NONE',  ( 33.58253175000000823, 24.27500000273120051, 10.91162601494192863 ) ) ;
#2007=CARTESIAN_POINT ( 'NONE',  ( -22.23068731925732422, 67.00000000000001421, -25.26668985625435226 ) ) ;
#2019=CARTESIAN_POINT ( 'NONE',  ( -20.75514604977248112, 63.67500000273116711, 28.56700777964554661 ) ) ;
#2025=EDGE_CURVE ( 'NONE', #24744, #7658, #28169, .T. ) ;
#2027=CARTESIAN_POINT ( 'NONE',  ( -26.29305231718578995, 78.20000000000000284, 19.10302069950538595 ) ) ;
#2028=CARTESIAN_POINT ( 'NONE',  ( 27.16883889988624290, 23.92500000273119198, 19.73931689729373673 ) ) ;
#2031=DIRECTION ( 'NONE',  ( 0.000000000000000000, 1.000000000000000000, 0.000000000000000000 ) ) ;
#2033=CARTESIAN_POINT ( 'NONE',  ( 32.50000000000000000, 41.60000000546238397, -10.55989012756945833 ) ) ;
#2039=CARTESIAN_POINT ( 'NONE',  ( -33.58253175000000113, 67.12500000273118417, 0.000000000000000000 ) ) ;
#2045=CARTESIAN_POINT ( 'NONE',  ( 10.37757302488624767, 11.72500000273117493, 31.93888565452638417 ) ) ;
#2054=CARTESIAN_POINT ( 'NONE',  ( 32.50000000000000000, 29.10000000000000853, -10.55989012756945833 ) ) ;
#2067=CARTESIAN_POINT ( 'NONE',  ( 6.486482029760649416E-15, 39.62500000273117706, 35.31076352940723240 ) ) ;
#2068=CARTESIAN_POINT ( 'NONE',  ( -10.37757302488624411, 2.975000002731182036, -31.93888565452638417 ) ) ;
#2069=CARTESIAN_POINT ( 'NONE',  ( 27.16883889988624290, 54.17500000273118843, 19.73931689729373673 ) ) ;
#2073=CARTESIAN_POINT ( 'NONE',  ( -32.50000000000000000, 58.40000000546237402, -10.55989012756945478 ) ) ;
#2081=CARTESIAN_POINT ( 'NONE',  ( -33.58253175000000113, 37.47500000273118559, 10.91162601494193929 ) ) ;
#2083=ORIENTED_EDGE ( 'NONE', *, *, #26141, .F. ) ;
#2085=CARTESIAN_POINT ( 'NONE',  ( 20.08610463437158344, 25.20000000546237473, 27.64615127144129403 ) ) ;
#2105=CARTESIAN_POINT ( 'NONE',  ( 10.37757302488624056, 72.77500000273118985, -31.93888565452638417 ) ) ;
#2106=ORIENTED_EDGE ( 'NONE', *, *, #949, .T. ) ;
#2110=CARTESIAN_POINT ( 'NONE',  ( 33.58253175000000113, 58.12500000273116996, -4.112674001490185761E-15 ) ) ;
#2111=CARTESIAN_POINT ( 'NONE',  ( -20.75514604977248823, 25.07500000273120122, -28.56700777964554305 ) ) ;
#2112=CARTESIAN_POINT ( 'NONE',  ( 33.58253175000000113, 12.47500000273119447, -10.91162601494193751 ) ) ;
#2116=CARTESIAN_POINT ( 'NONE',  ( -33.58253175000000113, 5.025000002731194293, -10.91162601494193218 ) ) ;
#2118=CARTESIAN_POINT ( 'NONE',  ( 32.50000000000000711, 40.89999999999998437, 10.55989012756945122 ) ) ;
#2122=CARTESIAN_POINT ( 'NONE',  ( 20.75514604977249178, 52.07500000273119412, 28.56700777964553950 ) ) ;
#2127=CARTESIAN_POINT ( 'NONE',  ( -33.58253175000000113, 21.12500000273119483, 0.000000000000000000 ) ) ;
#2141=CARTESIAN_POINT ( 'NONE',  ( 20.08610463437158344, 54.69999999999998153, 27.64615127144129403 ) ) ;
#2142=CARTESIAN_POINT ( 'NONE',  ( -32.49999999999985789, 52.10000000000001563, 10.55989012756966083 ) ) ;
#2147=CARTESIAN_POINT ( 'NONE',  ( 27.16883889988624290, 77.92500000273118133, 19.73931689729373673 ) ) ;
#2148=CARTESIAN_POINT ( 'NONE',  ( -20.75514604977248112, 41.67500000273117422, 28.56700777964554661 ) ) ;
#2153=( BOUNDED_CURVE ( )  B_SPLINE_CURVE ( 2, ( #19559, #16479, #16321, #24533, #11164, #21800, #3599, #3933, #6512, #29342, #30007, #24696, #1173 ),
 .UNSPECIFIED., .F., .T. ) 
 B_SPLINE_CURVE_WITH_KNOTS ( ( 3, 2, 2, 2, 2, 2, 3 ),
 ( 0.2500000000000000000, 0.2512820512820512775, 0.2538461538461538325, 0.2564102564102563875, 0.2589743589743589980, 0.2615384615384615530, 0.2628205128205128305 ),
 .UNSPECIFIED. ) 
 CURVE ( )  GEOMETRIC_REPRESENTATION_ITEM ( )  RATIONAL_B_SPLINE_CURVE ( ( 0.9755282581475768211, 0.9755282581475768211, 1.000000000000000000, 0.9510565162951535312, 1.000000000000000000, 0.9510565162951535312, 1.000000000000000000, 0.9510565162951535312, 1.000000000000000000, 0.9510565162951535312, 1.000000000000000000, 0.9755282581475768211, 0.9755282581475768211 ) ) 
 REPRESENTATION_ITEM ( '' )  );
#2154=CARTESIAN_POINT ( 'NONE',  ( 26.29305231718579350, 58.80000000000000426, 19.10302069950537529 ) ) ;
#2158=CARTESIAN_POINT ( 'NONE',  ( -33.58253175000000113, 75.37500000273118417, 0.000000000000000000 ) ) ;
#2163=CARTESIAN_POINT ( 'NONE',  ( 20.75514604977249178, 49.82500000273117990, 28.56700777964553950 ) ) ;
#2166=DIRECTION ( 'NONE',  ( 0.000000000000000000, 0.000000000000000000, 1.000000000000000000 ) ) ;
#2167=CARTESIAN_POINT ( 'NONE',  ( 10.04305231718579705, 3.100000005462372421, 30.90933677959248982 ) ) ;
#2168=CARTESIAN_POINT ( 'NONE',  ( 0.000000000000000000, 52.00000000000000711, 32.50000000000000000 ) ) ;
#2187=CARTESIAN_POINT ( 'NONE',  ( 33.58253175000000113, 64.37500000273121259, -4.112674001490185761E-15 ) ) ;
#2193=CARTESIAN_POINT ( 'NONE',  ( 32.50000000000000711, 78.89999999999999147, 10.55989012756945122 ) ) ;
#2194=CARTESIAN_POINT ( 'NONE',  ( -2.162160676586881955E-15, 14.62500000273118239, -35.31076352940723240 ) ) ;
#2199=CARTESIAN_POINT ( 'NONE',  ( -20.08610463437157989, 42.20000000546239249, -27.64615127144129758 ) ) ;
#2204=CARTESIAN_POINT ( 'NONE',  ( -20.75514604977248823, 66.82500000273118701, -28.56700777964554305 ) ) ;
#2210=CARTESIAN_POINT ( 'NONE',  ( 6.486482029760649416E-15, 11.62500000273118950, 35.31076352940723240 ) ) ;
#2218=LINE ( 'NONE', #25223, #6094 ) ;
#2222=CARTESIAN_POINT ( 'NONE',  ( -20.08610463437156923, 26.29999999999998295, 27.64615127144130113 ) ) ;
#2226=CARTESIAN_POINT ( 'NONE',  ( -12.54892211412393266, 66.99999999999995737, 30.22116052075399750 ) ) ;
#2237=CARTESIAN_POINT ( 'NONE',  ( -33.58253175000000113, 39.22500000273119269, 10.91162601494193929 ) ) ;
#2242=LINE ( 'NONE', #25419, #32443 ) ;
#2244=CARTESIAN_POINT ( 'NONE',  ( -20.08610463437156923, 62.80000000546237970, 27.64615127144130113 ) ) ;
#2252=CARTESIAN_POINT ( 'NONE',  ( 10.37757302488624767, 35.97500000273119980, 31.93888565452638417 ) ) ;
#2256=CARTESIAN_POINT ( 'NONE',  ( -26.29305231718579350, 26.30000000546238326, -19.10302069950537884 ) ) ;
#2261=VERTEX_POINT ( 'NONE', #28849 ) ;
#2268=CARTESIAN_POINT ( 'NONE',  ( 10.37757302488624056, 58.52500000273118275, -31.93888565452638417 ) ) ;
#2278=CARTESIAN_POINT ( 'NONE',  ( 27.16883889988624290, 72.17500000273118133, 19.73931689729373673 ) ) ;
#2283=CARTESIAN_POINT ( 'NONE',  ( -27.16883889988623935, 61.32500000273120833, 19.73931689729374739 ) ) ;
#2284=CARTESIAN_POINT ( 'NONE',  ( -33.58253175000000113, 17.37500000273119127, 0.000000000000000000 ) ) ;
#2285=CARTESIAN_POINT ( 'NONE',  ( -33.58253175000000113, 11.47500000273119625, 10.91162601494193929 ) ) ;
#2290=CARTESIAN_POINT ( 'NONE',  ( -10.37757302488624411, 4.725000002731183812, -31.93888565452638417 ) ) ;
#2293=CARTESIAN_POINT ( 'NONE',  ( -20.08610463437157989, 39.70000000000000284, -27.64615127144129758 ) ) ;
#2299=CARTESIAN_POINT ( 'NONE',  ( 10.37757302488624056, 56.77500000273121117, -31.93888565452638417 ) ) ;
#2300=CARTESIAN_POINT ( 'NONE',  ( 1.093617666956751375E-13, 60.00000000546238255, -32.50000000000000711 ) ) ;
#2304=CARTESIAN_POINT ( 'NONE',  ( 27.16883889988624290, 25.92500000273119554, 19.73931689729373673 ) ) ;
#2317=CARTESIAN_POINT ( 'NONE',  ( -1.137977401836464321E-14, 66.99999999999998579, 46.18802153517007270 ) ) ;
#2318=CARTESIAN_POINT ( 'NONE',  ( 26.29305231718579350, 16.79999999999999716, 19.10302069950537529 ) ) ;
#2323=CARTESIAN_POINT ( 'NONE',  ( 10.37757302488624056, 76.52500000273120406, -31.93888565452638417 ) ) ;
#2324=CARTESIAN_POINT ( 'NONE',  ( 33.58253175000000113, 36.47500000273119269, -10.91162601494193751 ) ) ;
#2328=CARTESIAN_POINT ( 'NONE',  ( -32.50000000000000000, 59.99999999999998579, 0.000000000000000000 ) ) ;
#2335=CARTESIAN_POINT ( 'NONE',  ( -33.58253175000000113, 75.47500000273116427, 10.91162601494193929 ) ) ;
#2340=CARTESIAN_POINT ( 'NONE',  ( 27.16883889988624290, 43.92500000273118133, 19.73931689729373673 ) ) ;
#2341=ORIENTED_EDGE ( 'NONE', *, *, #33551, .T. ) ;
#2345=CARTESIAN_POINT ( 'NONE',  ( 26.29305231718578995, 1.700000005462373842, -19.10302069950538240 ) ) ;
#2365=CARTESIAN_POINT ( 'NONE',  ( 20.75514604977249178, 60.07500000273119412, 28.56700777964553950 ) ) ;
#2372=CARTESIAN_POINT ( 'NONE',  ( -27.16883889988624290, 16.92500000273118488, -19.73931689729374028 ) ) ;
#2378=CARTESIAN_POINT ( 'NONE',  ( 10.04305231718578817, 35.90000000546238113, -30.90933677959249337 ) ) ;
#2380=CARTESIAN_POINT ( 'NONE',  ( -26.29305231718578995, 66.19999999999998863, 19.10302069950538595 ) ) ;
#2385=CARTESIAN_POINT ( 'NONE',  ( 27.16883889988624290, 59.92500000273119554, 19.73931689729373673 ) ) ;
#2391=CARTESIAN_POINT ( 'NONE',  ( 33.58253175000000113, 14.22500000273119625, -10.91162601494193751 ) ) ;
#2403=CARTESIAN_POINT ( 'NONE',  ( -32.50000000000000000, 27.89999999999999147, -10.55989012756945478 ) ) ;
#2407=CARTESIAN_POINT ( 'NONE',  ( -32.87414713444680103, 67.00000000000000000, -6.322578566051472393 ) ) ;
#2416=CARTESIAN_POINT ( 'NONE',  ( -10.37757302488624411, 34.72500000273119269, -31.93888565452638417 ) ) ;
#2421=CARTESIAN_POINT ( 'NONE',  ( -20.08610463437157989, 52.20000000546236407, -27.64615127144129758 ) ) ;
#2428=CARTESIAN_POINT ( 'NONE',  ( 33.58253175000000823, 32.27500000273117564, 10.91162601494192863 ) ) ;
#2432=CARTESIAN_POINT ( 'NONE',  ( 32.50000000000000000, 21.60000000546237331, -10.55989012756945833 ) ) ;
#2444=CARTESIAN_POINT ( 'NONE',  ( -20.75514604977248823, 58.82500000273117990, -28.56700777964554305 ) ) ;
#2454=CARTESIAN_POINT ( 'NONE',  ( -2.162160676586881955E-15, 76.87500000273115575, -35.31076352940723240 ) ) ;
#2459=CARTESIAN_POINT ( 'NONE',  ( -33.58253175000000113, 57.02500000273118275, -10.91162601494193218 ) ) ;
#2460=CARTESIAN_POINT ( 'NONE',  ( 33.58253175000000823, 20.27500000273117564, 10.91162601494192863 ) ) ;
#2461=CARTESIAN_POINT ( 'NONE',  ( 33.58253175000000823, 4.275000002731189852, 10.91162601494192863 ) ) ;
#2465=CARTESIAN_POINT ( 'NONE',  ( 20.75514604977248467, 4.425000002731183990, -28.56700777964554305 ) ) ;
#2466=( BOUNDED_CURVE ( )  B_SPLINE_CURVE ( 2, ( #11820, #6338, #3594, #16981, #9235, #14068, #29337, #13733, #5839, #24529, #11484, #14236, #8904 ),
 .UNSPECIFIED., .F., .T. ) 
 B_SPLINE_CURVE_WITH_KNOTS ( ( 3, 2, 2, 2, 2, 2, 3 ),
 ( 0.2371794871794871973, 0.2384615384615384748, 0.2410256410256410298, 0.2435897435897435848, 0.2461538461538461675, 0.2487179487179487225, 0.2500000000000000000 ),
 .UNSPECIFIED. ) 
 CURVE ( )  GEOMETRIC_REPRESENTATION_ITEM ( )  RATIONAL_B_SPLINE_CURVE ( ( 0.9755282581475768211, 0.9755282581475770431, 1.000000000000000000, 0.9510565162951535312, 1.000000000000000000, 0.9510565162951535312, 1.000000000000000000, 0.9510565162951535312, 1.000000000000000000, 0.9510565162951535312, 1.000000000000000000, 0.9755282581475768211, 0.9755282581475768211 ) ) 
 REPRESENTATION_ITEM ( '' )  );
#2473=CARTESIAN_POINT ( 'NONE',  ( -10.37757302488623701, 53.77500000273120406, 31.93888565452638417 ) ) ;
#2474=CARTESIAN_POINT ( 'NONE',  ( 32.50000000000000711, 59.40000000546237402, 10.55989012756945122 ) ) ;
#2478=CARTESIAN_POINT ( 'NONE',  ( 20.75514604977248467, 26.42500000273118843, -28.56700777964554305 ) ) ;
#2482=CARTESIAN_POINT ( 'NONE',  ( -10.04305231718578462, 58.39999999999999147, 30.90933677959249337 ) ) ;
#2492=CARTESIAN_POINT ( 'NONE',  ( 6.277390505771533514E-15, 16.50000000000000000, 34.17252228774368916 ) ) ;
#2499=CARTESIAN_POINT ( 'NONE',  ( 20.75514604977248467, 76.42500000273118133, -28.56700777964554305 ) ) ;
#2500=CARTESIAN_POINT ( 'NONE',  ( -33.58253175000000113, 35.47500000273118559, 10.91162601494193929 ) ) ;
#2507=CARTESIAN_POINT ( 'NONE',  ( -26.29305231718579350, 59.80000000000000426, -19.10302069950537884 ) ) ;
#2511=CARTESIAN_POINT ( 'NONE',  ( -33.58253175000000113, 73.47500000273117848, 10.91162601494193929 ) ) ;
#2517=ORIENTED_EDGE ( 'NONE', *, *, #3604, .F. ) ;
#2518=CARTESIAN_POINT ( 'NONE',  ( -10.37757302488624411, 44.72500000273120691, -31.93888565452638417 ) ) ;
#2522=CARTESIAN_POINT ( 'NONE',  ( -32.50000000000000000, 6.400000005462388231, -10.55989012756945478 ) ) ;
#2536=CARTESIAN_POINT ( 'NONE',  ( -40.00000000000000711, 52.00000000000000711, -23.09401076758504345 ) ) ;
#2543=CARTESIAN_POINT ( 'NONE',  ( -33.58253175000000113, 53.47500000273117848, 10.91162601494193929 ) ) ;
#2549=CARTESIAN_POINT ( 'NONE',  ( -10.04305231718578462, 78.40000000000000568, 30.90933677959249337 ) ) ;
#2550=CARTESIAN_POINT ( 'NONE',  ( 27.16883889988623935, 12.32500000273119234, -19.73931689729374384 ) ) ;
#2555=CARTESIAN_POINT ( 'NONE',  ( -32.50000000000000000, 38.40000000546235981, -10.55989012756945478 ) ) ;
#2560=CARTESIAN_POINT ( 'NONE',  ( 33.58253175000000113, 62.12500000273117706, -4.112674001490185761E-15 ) ) ;
#2566=CARTESIAN_POINT ( 'NONE',  ( -27.16883889988624290, 6.925000002731204418, -19.73931689729374028 ) ) ;
#2567=CARTESIAN_POINT ( 'NONE',  ( 1.076200423132605543E-16, 52.00000000000000711, -46.18802153517007980 ) ) ;
#2579=CARTESIAN_POINT ( 'NONE',  ( -10.04305231718578462, 32.39999999999999858, 30.90933677959249337 ) ) ;
#2591=CARTESIAN_POINT ( 'NONE',  ( 33.58253175000000113, 32.22500000273117848, -10.91162601494193751 ) ) ;
#2596=CARTESIAN_POINT ( 'NONE',  ( -20.08610463437157989, 56.20000000546239249, -27.64615127144129758 ) ) ;
#2598=( NAMED_UNIT ( * ) SI_UNIT ( $, .STERADIAN. ) SOLID_ANGLE_UNIT ( ) );
#2604=CARTESIAN_POINT ( 'NONE',  ( 27.16883889988624290, 32.17500000273120264, 19.73931689729373673 ) ) ;
#2608=CARTESIAN_POINT ( 'NONE',  ( 10.04305231718579705, 21.10000000546237331, 30.90933677959248982 ) ) ;
#2618=CARTESIAN_POINT ( 'NONE',  ( -2.162160676586882350E-15, 62.62500000273117706, -35.31076352940722529 ) ) ;
#2623=CARTESIAN_POINT ( 'NONE',  ( -5.147494577961174933, 66.94874572125284828, 32.49999991311200631 ) ) ;
#2628=VECTOR ( 'NONE', #19450, 1000.000000000000114 ) ;
#2629=CARTESIAN_POINT ( 'NONE',  ( -27.16883889988624290, 77.17500000273118133, -19.73931689729374028 ) ) ;
#2633=CARTESIAN_POINT ( 'NONE',  ( -20.75514604977248823, 56.82500000273117990, -28.56700777964554305 ) ) ;
#2634=CARTESIAN_POINT ( 'NONE',  ( 27.16883889988623935, 14.57500000273119412, -19.73931689729374384 ) ) ;
#2635=CARTESIAN_POINT ( 'NONE',  ( 10.37757302488624056, 2.775000002731189852, -31.93888565452638417 ) ) ;
#2639=CARTESIAN_POINT ( 'NONE',  ( 20.08610463437157279, 73.80000000546239391, -27.64615127144129758 ) ) ;
#2640=CARTESIAN_POINT ( 'NONE',  ( 32.46390416700889148, 52.00000000000002842, 8.309214287527991516 ) ) ;
#2646=CARTESIAN_POINT ( 'NONE',  ( 6.486482029760649416E-15, 53.87500000273118417, 35.31076352940723240 ) ) ;
#2650=EDGE_LOOP ( 'NONE', ( #21661, #22225, #26066, #12471 ) ) ;
#2652=CARTESIAN_POINT ( 'NONE',  ( -10.37757302488623701, 23.52500000273117919, 31.93888565452638417 ) ) ;
#2655=EDGE_LOOP ( 'NONE', ( #11680, #2341, #6891 ) ) ;
#2668=CARTESIAN_POINT ( 'NONE',  ( -26.29305231718579350, 13.79999999999999361, -19.10302069950537884 ) ) ;
#2675=CARTESIAN_POINT ( 'NONE',  ( -10.37757302488623701, 71.52500000273118985, 31.93888565452638417 ) ) ;
#2676=CARTESIAN_POINT ( 'NONE',  ( 33.58253175000000113, 34.37500000273117706, -4.112674001490185761E-15 ) ) ;
#2682=CARTESIAN_POINT ( 'NONE',  ( -10.04305231718578462, 54.39999999999999147, 30.90933677959249337 ) ) ;
#2686=CARTESIAN_POINT ( 'NONE',  ( 27.16883889988624290, 72.17500000273118133, 19.73931689729373673 ) ) ;
#2691=CARTESIAN_POINT ( 'NONE',  ( -33.58253175000000113, 41.02500000273118985, -10.91162601494193218 ) ) ;
#2695=CARTESIAN_POINT ( 'NONE',  ( 32.50000000000000000, 5.500000005462371888, -3.980102097228898626E-15 ) ) ;
#2702=DIRECTION ( 'NONE',  ( 0.000000000000000000, 0.000000000000000000, 1.000000000000000000 ) ) ;
#2712=CARTESIAN_POINT ( 'NONE',  ( 33.58253175000000113, 56.47500000273116427, -10.91162601494193751 ) ) ;
#2718=CARTESIAN_POINT ( 'NONE',  ( 27.16883889988623935, 14.32500000273119412, -19.73931689729374384 ) ) ;
#2723=CARTESIAN_POINT ( 'NONE',  ( -32.50000000000000000, 34.40000000546236691, -10.55989012756945478 ) ) ;
#2728=CARTESIAN_POINT ( 'NONE',  ( -10.37757302488623701, 61.52500000273118985, 31.93888565452638417 ) ) ;
#2733=CARTESIAN_POINT ( 'NONE',  ( -33.58253175000000113, 5.225000002731188253, 10.91162601494193929 ) ) ;
#2741=CARTESIAN_POINT ( 'NONE',  ( 26.29305231718578995, 21.19999999999998153, -19.10302069950538240 ) ) ;
#2745=CARTESIAN_POINT ( 'NONE',  ( -32.79451539931719140, 66.99999999999994316, 5.771861194046820742 ) ) ;
#2753=CARTESIAN_POINT ( 'NONE',  ( -33.58253175000000113, 33.12500000273120548, 0.000000000000000000 ) ) ;
#2758=CARTESIAN_POINT ( 'NONE',  ( 10.04305231718578817, 53.90000000546239534, -30.90933677959249337 ) ) ;
#2767=CARTESIAN_POINT ( 'NONE',  ( -33.58253175000000113, 31.47500000273117493, 10.91162601494193929 ) ) ;
#2770=VERTEX_POINT ( 'NONE', #1870 ) ;
#2772=CARTESIAN_POINT ( 'NONE',  ( -26.29305231718579350, 18.30000000546237615, -19.10302069950537884 ) ) ;
#2782=CARTESIAN_POINT ( 'NONE',  ( -33.58253175000000113, 61.02500000273118985, -10.91162601494193041 ) ) ;
#2792=CARTESIAN_POINT ( 'NONE',  ( -33.58253175000000113, 73.37500000273118417, 0.000000000000000000 ) ) ;
#2796=CARTESIAN_POINT ( 'NONE',  ( 33.58253175000000113, 56.22500000273117138, -10.91162601494193751 ) ) ;
#2797=CARTESIAN_POINT ( 'NONE',  ( 27.16883889988623935, 18.57500000273119767, -19.73931689729374384 ) ) ;
#2798=CARTESIAN_POINT ( 'NONE',  ( 27.16883889988623935, 6.575000002731187898, -19.73931689729374384 ) ) ;
#2802=CARTESIAN_POINT ( 'NONE',  ( 10.04305231718578817, 71.90000000546238823, -30.90933677959249337 ) ) ;
#2803=CARTESIAN_POINT ( 'NONE',  ( 20.18813247507400988, 51.99999999999998579, -25.94218825114888105 ) ) ;
#2809=CARTESIAN_POINT ( 'NONE',  ( -33.58253175000000113, 51.27500000273118275, -10.91162601494193218 ) ) ;
#2814=CARTESIAN_POINT ( 'NONE',  ( 6.486482029760649416E-15, 23.62500000273119127, 35.31076352940723240 ) ) ;
#2816=ORIENTED_EDGE ( 'NONE', *, *, #21130, .T. ) ;
#2830=CARTESIAN_POINT ( 'NONE',  ( -32.50000000000000000, 18.09999999999998010, 10.55989012756946366 ) ) ;
#2836=CARTESIAN_POINT ( 'NONE',  ( 27.16883889988624290, 71.92500000273120975, 19.73931689729373673 ) ) ;
#2838=CARTESIAN_POINT ( 'NONE',  ( 10.37757302488624056, 36.77500000273118985, -31.93888565452638417 ) ) ;
#2844=CARTESIAN_POINT ( 'NONE',  ( 20.08610463437158344, 56.69999999999998153, 27.64615127144129403 ) ) ;
#2849=CARTESIAN_POINT ( 'NONE',  ( 10.37757302488624056, 74.77500000273117564, -31.93888565452638417 ) ) ;
#2850=CARTESIAN_POINT ( 'NONE',  ( -32.50000000000000000, 62.09999999999998721, 10.55989012756946366 ) ) ;
#2855=CARTESIAN_POINT ( 'NONE',  ( 27.16883889988624290, 41.92500000273118133, 19.73931689729373673 ) ) ;
#2859=CARTESIAN_POINT ( 'NONE',  ( -32.50000000000000000, 60.50000000546238965, 0.000000000000000000 ) ) ;
#2860=CARTESIAN_POINT ( 'NONE',  ( -26.29305231718579350, 6.300000005462380592, -19.10302069950537884 ) ) ;
#2866=( BOUNDED_CURVE ( )  B_SPLINE_CURVE ( 2, ( #25754, #18386, #15979, #10651, #31408, #15294, #13055, #33988, #28491, #15811, #26435, #12544, #12713 ),
 .UNSPECIFIED., .F., .F. ) 
 B_SPLINE_CURVE_WITH_KNOTS ( ( 3, 2, 2, 2, 2, 2, 3 ),
 ( 0.1730769230769230727, 0.1743589743589743501, 0.1769230769230769329, 0.1794871794871794879, 0.1820512820512820429, 0.1846153846153846256, 0.1858974358974359031 ),
 .UNSPECIFIED. ) 
 CURVE ( )  GEOMETRIC_REPRESENTATION_ITEM ( )  RATIONAL_B_SPLINE_CURVE ( ( 0.9755282581475768211, 0.9755282581475768211, 1.000000000000000000, 0.9510565162951535312, 1.000000000000000000, 0.9510565162951535312, 1.000000000000000000, 0.9510565162951535312, 1.000000000000000000, 0.9510565162951535312, 1.000000000000000000, 0.9755282581475768211, 0.9755282581475768211 ) ) 
 REPRESENTATION_ITEM ( '' )  );
#2883=CARTESIAN_POINT ( 'NONE',  ( 33.58253175000000113, 56.37500000273119838, -4.112674001490185761E-15 ) ) ;
#2889=CARTESIAN_POINT ( 'NONE',  ( -32.50000000000000000, 72.00000000000000000, 0.000000000000000000 ) ) ;
#2890=CARTESIAN_POINT ( 'NONE',  ( -20.75514604977248112, 15.42500000273118843, 28.56700777964554661 ) ) ;
#2894=CARTESIAN_POINT ( 'NONE',  ( -10.04305231718578462, 34.90000000546238113, 30.90933677959249337 ) ) ;
#2899=CARTESIAN_POINT ( 'NONE',  ( -2.162160676586881955E-15, 64.62500000273121259, -35.31076352940723240 ) ) ;
#2904=CARTESIAN_POINT ( 'NONE',  ( -20.75514604977248823, 6.825000002731195892, -28.56700777964554305 ) ) ;
#2905=VERTEX_POINT ( 'NONE', #2567 ) ;
#2915=CARTESIAN_POINT ( 'NONE',  ( 26.29305231718579350, 20.80000000000000071, 19.10302069950537529 ) ) ;
#2925=CARTESIAN_POINT ( 'NONE',  ( -17.00271606754838416, 51.99999999999998579, 28.39578712880047462 ) ) ;
#2926=CARTESIAN_POINT ( 'NONE',  ( 33.58253175000000113, 32.12500000273120548, -4.112674001490185761E-15 ) ) ;
#2928=CARTESIAN_POINT ( 'NONE',  ( 33.58253175000000823, 52.27500000273118275, 10.91162601494192685 ) ) ;
#2932=CARTESIAN_POINT ( 'NONE',  ( -20.08610463437157989, 54.20000000546237118, -27.64615127144129758 ) ) ;
#2934=FILL_AREA_STYLE_COLOUR ( '', #19452 ) ;
#2938=CARTESIAN_POINT ( 'NONE',  ( -27.16883889988623935, 31.57500000273118346, 19.73931689729374739 ) ) ;
#2942=CARTESIAN_POINT ( 'NONE',  ( -32.50000000000000000, 16.40000000546239178, -10.55989012756945478 ) ) ;
#2953=CARTESIAN_POINT ( 'NONE',  ( 6.486482029760648627E-15, 59.62500000273118417, 35.31076352940722529 ) ) ;
#2961=CARTESIAN_POINT ( 'NONE',  ( 5.779280353836490358E-15, 53.00000000546238255, 32.49999999999999289 ) ) ;
#2965=CARTESIAN_POINT ( 'NONE',  ( -27.16883889988623935, 67.57500000273118701, 19.73931689729374739 ) ) ;
#2969=CARTESIAN_POINT ( 'NONE',  ( 10.37757302488624767, 51.72500000273121401, 31.93888565452638417 ) ) ;
#2970=CARTESIAN_POINT ( 'NONE',  ( 20.75514604977248467, 18.67500000273120264, -28.56700777964554305 ) ) ;
#2971=CARTESIAN_POINT ( 'NONE',  ( -33.58253175000000113, 3.275000002731191628, -10.91162601494193218 ) ) ;
#2976=CARTESIAN_POINT ( 'NONE',  ( 32.50000000000000000, 75.50000000546238255, -3.980102097228898626E-15 ) ) ;
#2977=CARTESIAN_POINT ( 'NONE',  ( 31.78338918835718729, 52.00000000000002132, -9.699108655006703827 ) ) ;
#2984=CARTESIAN_POINT ( 'NONE',  ( -10.37757302488623701, 49.77500000273120406, 31.93888565452638417 ) ) ;
#2989=CARTESIAN_POINT ( 'NONE',  ( -33.58253175000000113, 15.12500000273118950, 0.000000000000000000 ) ) ;
#3003=CARTESIAN_POINT ( 'NONE',  ( 5.779280353836490358E-15, 60.49999999999998579, 32.49999999999999289 ) ) ;
#3004=CARTESIAN_POINT ( 'NONE',  ( -10.04305231718579172, 15.59999999999998899, -30.90933677959248982 ) ) ;
#3011=CARTESIAN_POINT ( 'NONE',  ( -33.58253175000000113, 73.12500000273118417, 0.000000000000000000 ) ) ;
#3012=CARTESIAN_POINT ( 'NONE',  ( -10.37757302488623701, 35.77500000273118985, 31.93888565452638417 ) ) ;
#3017=CARTESIAN_POINT ( 'NONE',  ( -2.092463501923844636E-15, 51.50000000000000711, -34.17252228774368916 ) ) ;
#3024=CARTESIAN_POINT ( 'NONE',  ( 10.37757302488624767, 65.97500000273119269, 31.93888565452638417 ) ) ;
#3025=CARTESIAN_POINT ( 'NONE',  ( -20.08610463437157989, 61.69999999999999574, -27.64615127144129758 ) ) ;
#3029=CARTESIAN_POINT ( 'NONE',  ( -10.37757302488624411, 40.72500000273119980, -31.93888565452638417 ) ) ;
#3034=CARTESIAN_POINT ( 'NONE',  ( 5.147494310547426899, 59.44874571845315359, -32.50000000000000000 ) ) ;
#3042=DIRECTION ( 'NONE',  ( 0.000000000000000000, 1.000000000000000000, 0.000000000000000000 ) ) ;
#3054=CARTESIAN_POINT ( 'NONE',  ( -33.58253175000000113, 57.47500000273119269, 10.91162601494193929 ) ) ;
#3060=CARTESIAN_POINT ( 'NONE',  ( -10.04305231718579172, 75.59999999999998010, -30.90933677959248982 ) ) ;
#3062=CARTESIAN_POINT ( 'NONE',  ( -33.58253175000000113, 11.02500000273117919, -10.91162601494193218 ) ) ;
#3071=CARTESIAN_POINT ( 'NONE',  ( -20.75514604977248112, 61.42500000273118133, 28.56700777964554661 ) ) ;
#3072=( BOUNDED_CURVE ( )  B_SPLINE_CURVE ( 2, ( #29163, #24036, #504, #10990, #21462, #26929, #31905, #21628, #8399, #5837, #3262, #24200, #32073 ),
 .UNSPECIFIED., .F., .T. ) 
 B_SPLINE_CURVE_WITH_KNOTS ( ( 3, 2, 2, 2, 2, 2, 3 ),
 ( 0.1858974358974359031, 0.1871794871794871806, 0.1897435897435897356, 0.1923076923076923184, 0.1948717948717948734, 0.1974358974358974284, 0.1987179487179487336 ),
 .UNSPECIFIED. ) 
 CURVE ( )  GEOMETRIC_REPRESENTATION_ITEM ( )  RATIONAL_B_SPLINE_CURVE ( ( 0.9755282581475768211, 0.9755282581475768211, 1.000000000000000000, 0.9510565162951535312, 1.000000000000000000, 0.9510565162951535312, 1.000000000000000000, 0.9510565162951535312, 1.000000000000000000, 0.9510565162951535312, 1.000000000000000000, 0.9755282581475764880, 0.9755282581475768211 ) ) 
 REPRESENTATION_ITEM ( '' )  );
#3076=CARTESIAN_POINT ( 'NONE',  ( -33.58253175000000113, 7.025000002731188964, -10.91162601494193218 ) ) ;
#3086=CARTESIAN_POINT ( 'NONE',  ( -32.50000000000000000, 23.90000000000000213, -10.55989012756945478 ) ) ;
#3098=CARTESIAN_POINT ( 'NONE',  ( 22.34582402162608616, 66.99999999999998579, -24.25905220314542277 ) ) ;
#3101=CARTESIAN_POINT ( 'NONE',  ( -27.16883889988624290, 32.92500000273117422, -19.73931689729374028 ) ) ;
#3103=CARTESIAN_POINT ( 'NONE',  ( 32.50000000000000000, 61.50000000546239676, -3.980102097228898626E-15 ) ) ;
#3106=CARTESIAN_POINT ( 'NONE',  ( 20.08610463437158344, 57.20000000546237828, 27.64615127144129403 ) ) ;
#3115=CARTESIAN_POINT ( 'NONE',  ( -2.092463501923844636E-15, 20.00000000546236834, -34.17252228774368916 ) ) ;
#3133=CARTESIAN_POINT ( 'NONE',  ( -20.75514604977248112, 71.67500000273116711, 28.56700777964554661 ) ) ;
#3138=CARTESIAN_POINT ( 'NONE',  ( -33.58253175000000113, 51.02500000273119696, -10.91162601494193218 ) ) ;
#3139=CARTESIAN_POINT ( 'NONE',  ( -27.16883889988623935, 9.575000002731190563, 19.73931689729374739 ) ) ;
#3140=CARTESIAN_POINT ( 'NONE',  ( -2.162160676586881955E-15, 4.875000002731200155, -35.31076352940723240 ) ) ;
#3145=CARTESIAN_POINT ( 'NONE',  ( 26.29305231718578995, 75.70000000546238539, -19.10302069950538240 ) ) ;
#3153=CARTESIAN_POINT ( 'NONE',  ( -10.37757302488624411, 44.97500000273117848, -31.93888565452638417 ) ) ;
#3159=CARTESIAN_POINT ( 'NONE',  ( 33.58253175000000113, 16.22500000273118914, -10.91162601494193751 ) ) ;
#3175=CARTESIAN_POINT ( 'NONE',  ( 32.50000000000000711, 12.90000000000000036, 10.55989012756945122 ) ) ;
#3181=CARTESIAN_POINT ( 'NONE',  ( -33.58253175000000113, 71.12500000273118417, 0.000000000000000000 ) ) ;
#3182=CARTESIAN_POINT ( 'NONE',  ( -10.37757302488624411, 30.97500000273119269, -31.93888565452638417 ) ) ;
#3187=CARTESIAN_POINT ( 'NONE',  ( 32.50000000000000711, 50.89999999999999858, 10.55989012756945122 ) ) ;
#3194=CARTESIAN_POINT ( 'NONE',  ( -20.75514604977248823, 69.07500000273115859, -28.56700777964554305 ) ) ;
#3200=CARTESIAN_POINT ( 'NONE',  ( -27.16883889988623935, 37.32500000273118701, 19.73931689729374739 ) ) ;
#3202=ORIENTED_EDGE ( 'NONE', *, *, #9641, .T. ) ;
#3205=CARTESIAN_POINT ( 'NONE',  ( 10.04305231718579705, 58.60000000000000142, 30.90933677959248982 ) ) ;
#3217=CARTESIAN_POINT ( 'NONE',  ( -32.50000000000000000, 54.60000000546237686, 10.55989012756946366 ) ) ;
#3221=CARTESIAN_POINT ( 'NONE',  ( 20.75514604977249178, 54.07500000273118701, 28.56700777964553950 ) ) ;
#3227=CARTESIAN_POINT ( 'NONE',  ( 20.08610463437158344, 72.70000000000001705, 27.64615127144129403 ) ) ;
#3228=CARTESIAN_POINT ( 'NONE',  ( -20.75514604977248823, 10.82500000273118701, -28.56700777964554305 ) ) ;
#3236=CARTESIAN_POINT ( 'NONE',  ( -33.58253175000000113, 55.12500000273119838, 0.000000000000000000 ) ) ;
#3240=CARTESIAN_POINT ( 'NONE',  ( -10.37757302488624411, 6.725000002731185589, -31.93888565452638417 ) ) ;
#3249=CARTESIAN_POINT ( 'NONE',  ( 6.277390505771533514E-15, 24.50000000000001421, 34.17252228774368916 ) ) ;
#3260=CARTESIAN_POINT ( 'NONE',  ( -30.22248186753587973, 52.00000000000002842, 12.55019540181404736 ) ) ;
#3261=CARTESIAN_POINT ( 'NONE',  ( -27.16883889988623935, 27.32500000273117990, 19.73931689729374739 ) ) ;
#3262=CARTESIAN_POINT ( 'NONE',  ( 10.04305231718579705, 64.60000000000000853, 30.90933677959248982 ) ) ;
#3266=CARTESIAN_POINT ( 'NONE',  ( -26.29305231718578995, 50.70000000546236407, 19.10302069950538595 ) ) ;
#3276=CARTESIAN_POINT ( 'NONE',  ( -20.08610463437157989, 20.20000000546239249, -27.64615127144129758 ) ) ;
#3288=CARTESIAN_POINT ( 'NONE',  ( -33.58253175000000113, 53.02500000273118985, -10.91162601494193041 ) ) ;
#3297=EDGE_CURVE ( 'NONE', #33362, #1345, #15710, .T. ) ;
#3298=CARTESIAN_POINT ( 'NONE',  ( 20.75514604977249178, 70.07500000273120122, 28.56700777964553950 ) ) ;
#3303=CARTESIAN_POINT ( 'NONE',  ( -10.37757302488624411, 44.72500000273120691, -31.93888565452638417 ) ) ;
#3304=CARTESIAN_POINT ( 'NONE',  ( -33.58253175000000113, 13.47500000273118914, 10.91162601494193929 ) ) ;
#3305=CARTESIAN_POINT ( 'NONE',  ( -27.16883889988623935, 61.57500000273117990, 19.73931689729374739 ) ) ;
#3310=CARTESIAN_POINT ( 'NONE',  ( 32.50000000000000000, 71.60000000546240528, -10.55989012756945833 ) ) ;
#3317=CARTESIAN_POINT ( 'NONE',  ( -27.16883889988624290, 47.17500000273118843, -19.73931689729374028 ) ) ;
#3322=CARTESIAN_POINT ( 'NONE',  ( -10.37757302488624411, 16.72500000273117848, -31.93888565452638417 ) ) ;
#3335=CARTESIAN_POINT ( 'NONE',  ( 32.50000000000000000, 8.999999999999994671, -3.980102097228898626E-15 ) ) ;
#3343=CARTESIAN_POINT ( 'NONE',  ( -10.37757302488624411, 70.72500000273117848, -31.93888565452638417 ) ) ;
#3344=CARTESIAN_POINT ( 'NONE',  ( -2.162160676586881955E-15, 28.87500000273119838, -35.31076352940723240 ) ) ;
#3345=CARTESIAN_POINT ( 'NONE',  ( -33.58253175000000113, 19.47500000273117493, 10.91162601494193929 ) ) ;
#3351=CARTESIAN_POINT ( 'NONE',  ( 26.29305231718578995, 53.20000000000000995, -19.10302069950538240 ) ) ;
#3356=CARTESIAN_POINT ( 'NONE',  ( 10.37757302488624767, 69.97500000273119269, 31.93888565452638417 ) ) ;
#3361=CARTESIAN_POINT ( 'NONE',  ( 33.58253175000000113, 36.12500000273118417, -4.112674001490185761E-15 ) ) ;
#3384=CARTESIAN_POINT ( 'NONE',  ( -20.75514604977248823, 47.07500000273117990, -28.56700777964554305 ) ) ;
#3391=CARTESIAN_POINT ( 'NONE',  ( -20.08610463437156923, 76.30000000000001137, 27.64615127144130113 ) ) ;
#3392=CARTESIAN_POINT ( 'NONE',  ( 33.58253175000000113, 10.22500000273118914, -10.91162601494193751 ) ) ;
#3401=CARTESIAN_POINT ( 'NONE',  ( 33.58253175000000823, 56.02500000273117564, 10.91162601494192863 ) ) ;
#3405=CARTESIAN_POINT ( 'NONE',  ( 0.000000000000000000, 52.00000000000000711, 0.000000000000000000 ) ) ;
#3413=CARTESIAN_POINT ( 'NONE',  ( -2.092463501923844636E-15, 21.49999999999998934, -34.17252228774368916 ) ) ;
#3421=ADVANCED_FACE ( 'NONE', ( #16873 ), #22191, .F. ) ;
#3424=CARTESIAN_POINT ( 'NONE',  ( 31.32135535759086054, 66.99999999999997158, -9.352374566761925578 ) ) ;
#3426=CARTESIAN_POINT ( 'NONE',  ( 27.16883889988623935, 30.32500000273117990, -19.73931689729374384 ) ) ;
#3427=CARTESIAN_POINT ( 'NONE',  ( 10.04305231718579705, 56.59999999999999432, 30.90933677959248982 ) ) ;
#3428=CARTESIAN_POINT ( 'NONE',  ( 26.29305231718579350, 61.30000000546238681, 19.10302069950537529 ) ) ;
#3431=CARTESIAN_POINT ( 'NONE',  ( -32.50000000000000000, 50.50000000546238255, 0.000000000000000000 ) ) ;
#3438=CARTESIAN_POINT ( 'NONE',  ( 10.37757302488624056, 74.52500000273120406, -31.93888565452638417 ) ) ;
#3443=CARTESIAN_POINT ( 'NONE',  ( -32.50000000000000000, 14.50000000546237899, 0.000000000000000000 ) ) ;
#3461=CARTESIAN_POINT ( 'NONE',  ( -10.37757302488623701, 67.77500000273118985, 31.93888565452638417 ) ) ;
#3466=CARTESIAN_POINT ( 'NONE',  ( 20.75514604977249178, 49.82500000273117990, 28.56700777964553950 ) ) ;
#3467=CARTESIAN_POINT ( 'NONE',  ( -10.37757302488623701, 11.77500000273117031, 31.93888565452638417 ) ) ;
#3468=CARTESIAN_POINT ( 'NONE',  ( 27.16883889988623935, 62.57500000273117990, -19.73931689729374384 ) ) ;
#3472=CARTESIAN_POINT ( 'NONE',  ( 20.08610463437157279, 67.80000000546236549, -27.64615127144129758 ) ) ;
#3478=CARTESIAN_POINT ( 'NONE',  ( 20.75514604977248467, 50.67500000273117422, -28.56700777964554305 ) ) ;
#3483=CARTESIAN_POINT ( 'NONE',  ( 20.75514604977249178, 17.82500000273120122, 28.56700777964553950 ) ) ;
#3492=CARTESIAN_POINT ( 'NONE',  ( 0.000000000000000000, 52.00000000000000711, 0.000000000000000000 ) ) ;
#3497=CARTESIAN_POINT ( 'NONE',  ( 26.29305231718579350, 65.30000000546236549, 19.10302069950537529 ) ) ;
#3499=CARTESIAN_POINT ( 'NONE',  ( 20.08610463437158344, 12.70000000000000639, 27.64615127144129403 ) ) ;
#3505=CARTESIAN_POINT ( 'NONE',  ( -10.37757302488623701, 67.52500000273118985, 31.93888565452638417 ) ) ;
#3506=CARTESIAN_POINT ( 'NONE',  ( 33.58253175000000113, 30.37500000273117706, -4.112674001490185761E-15 ) ) ;
#3507=CARTESIAN_POINT ( 'NONE',  ( -2.162160676586881955E-15, 18.87500000273119483, -35.31076352940723240 ) ) ;
#3514=CARTESIAN_POINT ( 'NONE',  ( -32.50000000000000000, 50.00000000000000000, 0.000000000000000000 ) ) ;
#3519=CARTESIAN_POINT ( 'NONE',  ( 20.75514604977249178, 70.07500000273120122, 28.56700777964553950 ) ) ;
#3524=CARTESIAN_POINT ( 'NONE',  ( 10.37757302488624767, 35.72500000273119980, 31.93888565452638417 ) ) ;
#3525=CARTESIAN_POINT ( 'NONE',  ( 0.000000000000000000, 52.00000000000000711, 0.000000000000000000 ) ) ;
#3529=CARTESIAN_POINT ( 'NONE',  ( 32.50000000000000711, 58.90000000000000568, 10.55989012756945122 ) ) ;
#3540=CARTESIAN_POINT ( 'NONE',  ( 26.29305231718579350, 53.30000000546237970, 19.10302069950537529 ) ) ;
#3545=CARTESIAN_POINT ( 'NONE',  ( -33.58253175000000113, 49.37500000273119127, 0.000000000000000000 ) ) ;
#3551=CARTESIAN_POINT ( 'NONE',  ( 6.277390505771533514E-15, 70.50000000000001421, 34.17252228774368916 ) ) ;
#3552=CARTESIAN_POINT ( 'NONE',  ( -27.16883889988623935, 7.325000002731188786, 19.73931689729374739 ) ) ;
#3562=CARTESIAN_POINT ( 'NONE',  ( -27.16883889988623935, 57.32500000273120833, 19.73931689729374739 ) ) ;
#3563=CARTESIAN_POINT ( 'NONE',  ( -27.16883889988623935, 29.57500000273117990, 19.73931689729374739 ) ) ;
#3575=LINE ( 'NONE', #24508, #31320 ) ;
#3591=CARTESIAN_POINT ( 'NONE',  ( 20.75514604977249178, 29.82500000273119767, 28.56700777964553950 ) ) ;
#3593=CARTESIAN_POINT ( 'NONE',  ( 20.08610463437158344, 61.20000000546237118, 27.64615127144129403 ) ) ;
#3594=CARTESIAN_POINT ( 'NONE',  ( 10.04305231718578817, 61.39999999999999858, -30.90933677959249337 ) ) ;
#3596=CARTESIAN_POINT ( 'NONE',  ( -10.04305231718579172, 50.10000000546236976, -30.90933677959248982 ) ) ;
#3599=CARTESIAN_POINT ( 'NONE',  ( -32.50000000000000000, 58.50000000546238965, 0.000000000000000000 ) ) ;
#3601=ORIENTED_EDGE ( 'NONE', *, *, #9641, .F. ) ;
#3602=CARTESIAN_POINT ( 'NONE',  ( 10.37757302488624767, 75.72500000273117848, 31.93888565452638417 ) ) ;
#3604=EDGE_CURVE ( 'NONE', #22688, #2905, #9132, .T. ) ;
#3605=CYLINDRICAL_SURFACE ( 'NONE', #16298, 32.50000000000000000 ) ;
#3609=CARTESIAN_POINT ( 'NONE',  ( 10.04305231718579705, 11.10000000546239285, 30.90933677959248982 ) ) ;
#3616=CARTESIAN_POINT ( 'NONE',  ( -32.50000000000000000, 62.60000000546238397, 10.55989012756946366 ) ) ;
#3619=CARTESIAN_POINT ( 'NONE',  ( 32.50000000000000711, 32.89999999999997726, 10.55989012756945122 ) ) ;
#3627=CARTESIAN_POINT ( 'NONE',  ( -2.162160676586881955E-15, 66.87500000273119838, -35.31076352940723240 ) ) ;
#3632=CARTESIAN_POINT ( 'NONE',  ( -33.58253175000000113, 49.22500000273119269, 10.91162601494193929 ) ) ;
#3633=CARTESIAN_POINT ( 'NONE',  ( 20.75514604977249178, 8.075000002731185234, 28.56700777964553950 ) ) ;
#3634=CARTESIAN_POINT ( 'NONE',  ( -10.37757302488623701, 63.77500000273118985, 31.93888565452638417 ) ) ;
#3638=CARTESIAN_POINT ( 'NONE',  ( -20.08610463437156923, 66.80000000546236549, 27.64615127144130113 ) ) ;
#3644=CARTESIAN_POINT ( 'NONE',  ( 33.58253175000000113, 44.37500000273119127, -4.112674001490185761E-15 ) ) ;
#3646=CARTESIAN_POINT ( 'NONE',  ( 32.50000000000000000, 27.50000000546236478, -3.980102097228898626E-15 ) ) ;
#3648=CARTESIAN_POINT ( 'NONE',  ( 33.58253175000000823, 18.02500000273118630, 10.91162601494192863 ) ) ;
#3666=CARTESIAN_POINT ( 'NONE',  ( -2.092463501923844636E-15, 9.499999999999991118, -34.17252228774368916 ) ) ;
#3672=CARTESIAN_POINT ( 'NONE',  ( 20.75514604977249178, 65.82500000273115859, 28.56700777964553950 ) ) ;
#3673=CARTESIAN_POINT ( 'NONE',  ( 33.58253175000000113, 28.47500000273118204, -10.91162601494193751 ) ) ;
#3674=CARTESIAN_POINT ( 'NONE',  ( 27.16883889988624290, 18.17500000273118843, 19.73931689729373673 ) ) ;
#3680=CARTESIAN_POINT ( 'NONE',  ( -10.04305231718578462, 46.39999999999998437, 30.90933677959249337 ) ) ;
#3681=CARTESIAN_POINT ( 'NONE',  ( 5.147494310547434893, 57.05125428700922185, 32.49999999999999289 ) ) ;
#3685=CARTESIAN_POINT ( 'NONE',  ( -10.37757302488623701, 65.77500000273118985, 31.93888565452638417 ) ) ;
#3691=CARTESIAN_POINT ( 'NONE',  ( 20.75514604977249178, 33.82500000273117990, 28.56700777964553950 ) ) ;
#3714=CARTESIAN_POINT ( 'NONE',  ( -27.16883889988623935, 51.57500000273117280, 19.73931689729374739 ) ) ;
#3721=CARTESIAN_POINT ( 'NONE',  ( -20.08610463437156923, 64.29999999999996874, 27.64615127144130113 ) ) ;
#3722=CARTESIAN_POINT ( 'NONE',  ( -2.162160676586881955E-15, 6.625000002731173510, -35.31076352940723240 ) ) ;
#3732=CARTESIAN_POINT ( 'NONE',  ( -20.75514604977248823, 58.82500000273117990, -28.56700777964554305 ) ) ;
#3733=CARTESIAN_POINT ( 'NONE',  ( 20.75514604977249178, 28.07500000273119412, 28.56700777964553950 ) ) ;
#3761=UNCERTAINTY_MEASURE_WITH_UNIT (LENGTH_MEASURE( 1.000000000000000082E-05 ), #29170, 'distance_accuracy_value', 'NONE');
#3762=CARTESIAN_POINT ( 'NONE',  ( -33.58253175000000113, 27.12500000273120193, 0.000000000000000000 ) ) ;
#3767=CARTESIAN_POINT ( 'NONE',  ( 32.50000000000000000, 47.50000000546238255, -3.980102097228898626E-15 ) ) ;
#3771=CARTESIAN_POINT ( 'NONE',  ( -10.37757302488623701, 77.52500000273120406, 31.93888565452638417 ) ) ;
#3776=CARTESIAN_POINT ( 'NONE',  ( 26.29305231718579350, 9.300000005462369046, 19.10302069950537529 ) ) ;
#3785=( NAMED_UNIT ( * ) PLANE_ANGLE_UNIT ( ) SI_UNIT ( $, .RADIAN. ) );
#3786=CARTESIAN_POINT ( 'NONE',  ( -26.29305231718578995, 36.19999999999999574, 19.10302069950538595 ) ) ;
#3793=CARTESIAN_POINT ( 'NONE',  ( 33.58253175000000823, 60.27500000273116143, 10.91162601494192863 ) ) ;
#3799=CARTESIAN_POINT ( 'NONE',  ( 27.16883889988623935, 50.32500000273120122, -19.73931689729374384 ) ) ;
#3800=CARTESIAN_POINT ( 'NONE',  ( -20.75514604977248823, 13.07500000273118879, -28.56700777964554305 ) ) ;
#3801=CARTESIAN_POINT ( 'NONE',  ( 27.16883889988623935, 60.57500000273117990, -19.73931689729374384 ) ) ;
#3806=CARTESIAN_POINT ( 'NONE',  ( 26.29305231718578995, 65.70000000546237118, -19.10302069950538240 ) ) ;
#3812=CARTESIAN_POINT ( 'NONE',  ( 10.37757302488624767, 39.97500000273117138, 31.93888565452638417 ) ) ;
#3814=CARTESIAN_POINT ( 'NONE',  ( -2.092463501923844636E-15, 32.00000000546236834, -34.17252228774368916 ) ) ;
#3817=EDGE_LOOP ( 'NONE', ( #32106, #15090, #16719, #14877 ) ) ;
#3831=CARTESIAN_POINT ( 'NONE',  ( -32.50000000000000000, 8.099999999999990763, 10.55989012756946366 ) ) ;
#3836=CARTESIAN_POINT ( 'NONE',  ( -27.16883889988623935, 65.32500000273118701, 19.73931689729374739 ) ) ;
#3837=CARTESIAN_POINT ( 'NONE',  ( 33.58253175000000113, 28.37500000273117351, -4.112674001490185761E-15 ) ) ;
#3838=CARTESIAN_POINT ( 'NONE',  ( 6.486482029760649416E-15, 15.87500000273120015, 35.31076352940723240 ) ) ;
#3844=CARTESIAN_POINT ( 'NONE',  ( 26.29305231718578995, 49.20000000000000995, -19.10302069950538240 ) ) ;
#3849=CARTESIAN_POINT ( 'NONE',  ( 6.486482029760649416E-15, 59.87500000273117706, 35.31076352940723240 ) ) ;
#3854=ORIENTED_EDGE ( 'NONE', *, *, #15671, .T. ) ;
#3855=CARTESIAN_POINT ( 'NONE',  ( -33.58253175000000113, 35.22500000273119980, 10.91162601494193929 ) ) ;
#3872=CARTESIAN_POINT ( 'NONE',  ( 5.779280353836490358E-15, 53.00000000546238255, 32.49999999999999289 ) ) ;
#3874=CARTESIAN_POINT ( 'NONE',  ( -20.08610463437156923, 54.80000000546236549, 27.64615127144130113 ) ) ;
#3878=CARTESIAN_POINT ( 'NONE',  ( -10.37757302488624411, 50.97500000273118559, -31.93888565452638417 ) ) ;
#3884=CARTESIAN_POINT ( 'NONE',  ( -32.50000000000000000, 65.89999999999997726, -10.55989012756945478 ) ) ;
#3896=CARTESIAN_POINT ( 'NONE',  ( -2.162160676586881955E-15, 56.62500000273116996, -35.31076352940723240 ) ) ;
#3897=CARTESIAN_POINT ( 'NONE',  ( 33.58253175000000113, 30.37500000273117706, -4.112674001490185761E-15 ) ) ;
#3903=EDGE_CURVE ( 'NONE', #17565, #30177, #21758, .T. ) ;
#3908=CARTESIAN_POINT ( 'NONE',  ( -1.778240108872766143E-15, 58.00000000546237544, -32.49999999999999289 ) ) ;
#3909=CARTESIAN_POINT ( 'NONE',  ( -29.16592172374821601, 67.00000000000004263, -16.79171150063893236 ) ) ;
#3912=CARTESIAN_POINT ( 'NONE',  ( 27.16883889988624290, 57.92500000273119554, 19.73931689729373673 ) ) ;
#3922=FACE_OUTER_BOUND ( 'NONE', #810, .T. ) ;
#3926=CARTESIAN_POINT ( 'NONE',  ( 33.58253175000000113, 30.12500000273120193, -4.112674001490185761E-15 ) ) ;
#3929=CARTESIAN_POINT ( 'NONE',  ( 20.08610463437158344, 52.69999999999998863, 27.64615127144129403 ) ) ;
#3932=CARTESIAN_POINT ( 'NONE',  ( -26.29305231718578995, 48.70000000546238539, 19.10302069950538595 ) ) ;
#3933=CARTESIAN_POINT ( 'NONE',  ( -32.50000000000000000, 58.40000000546237402, -10.55989012756945300 ) ) ;
#3937=CARTESIAN_POINT ( 'NONE',  ( -10.37757302488623701, 73.52500000273120406, 31.93888565452638417 ) ) ;
#3942=CARTESIAN_POINT ( 'NONE',  ( 20.08610463437157279, 9.800000005462381480, -27.64615127144129758 ) ) ;
#3949=CARTESIAN_POINT ( 'NONE',  ( -26.29305231718578995, 62.70000000546237118, 19.10302069950538595 ) ) ;
#3951=CARTESIAN_POINT ( 'NONE',  ( -10.04305231718578462, 38.40000000000000568, 30.90933677959249337 ) ) ;
#3965=CARTESIAN_POINT ( 'NONE',  ( -2.162160676586881955E-15, 50.62500000273118417, -35.31076352940723240 ) ) ;
#3966=CARTESIAN_POINT ( 'NONE',  ( -10.37757302488623701, 1.775000002731188964, 31.93888565452638417 ) ) ;
#3967=CARTESIAN_POINT ( 'NONE',  ( -27.16883889988624290, 59.17500000273119554, -19.73931689729374028 ) ) ;
#3972=CARTESIAN_POINT ( 'NONE',  ( -26.29305231718578995, 64.70000000546237118, 19.10302069950538595 ) ) ;
#3975=CARTESIAN_POINT ( 'NONE',  ( -26.29305231718578995, 54.20000000000000995, 19.10302069950538595 ) ) ;
#3978=CARTESIAN_POINT ( 'NONE',  ( 27.16883889988624290, 44.17500000273118133, 19.73931689729373673 ) ) ;
#3980=CARTESIAN_POINT ( 'NONE',  ( 20.08610463437157279, 31.80000000546237260, -27.64615127144129758 ) ) ;
#3990=CARTESIAN_POINT ( 'NONE',  ( 10.37757302488624767, 65.72500000273119269, 31.93888565452638417 ) ) ;
#3999=CARTESIAN_POINT ( 'NONE',  ( 32.50000000000000711, 4.900000000000005684, 10.55989012756945122 ) ) ;
#4002=CARTESIAN_POINT ( 'NONE',  ( 5.779280353836490358E-15, 58.49999999999999289, 32.49999999999999289 ) ) ;
#4004=CARTESIAN_POINT ( 'NONE',  ( -20.75514604977248823, 68.82500000273118701, -28.56700777964554305 ) ) ;
#4005=CARTESIAN_POINT ( 'NONE',  ( 10.37757302488624056, 26.77500000273118275, -31.93888565452638417 ) ) ;
#4006=CARTESIAN_POINT ( 'NONE',  ( 33.58253175000000823, 16.27500000273118630, 10.91162601494192863 ) ) ;
#4011=CARTESIAN_POINT ( 'NONE',  ( -26.29305231718578995, 48.20000000000000995, 19.10302069950538595 ) ) ;
#4017=CARTESIAN_POINT ( 'NONE',  ( -33.58253175000000113, 63.47500000273117138, 10.91162601494193929 ) ) ;
#4022=CARTESIAN_POINT ( 'NONE',  ( 20.75514604977249178, 31.82500000273119056, 28.56700777964553950 ) ) ;
#4044=CARTESIAN_POINT ( 'NONE',  ( -33.58253175000000113, 51.27500000273118275, -10.91162601494193218 ) ) ;
#4049=CARTESIAN_POINT ( 'NONE',  ( -32.50000000000000000, 66.10000000000000853, 10.55989012756946366 ) ) ;
#4056=( BOUNDED_CURVE ( )  B_SPLINE_CURVE ( 2, ( #17762, #28392, #2482, #18283, #15363, #13117, #18451, #31473, #13285, #33716, #15536, #20693, #21192 ),
 .UNSPECIFIED., .F., .T. ) 
 B_SPLINE_CURVE_WITH_KNOTS ( ( 3, 2, 2, 2, 2, 2, 3 ),
 ( 0.2756410256410256610, 0.2769230769230769384, 0.2794871794871794934, 0.2820512820512820484, 0.2846153846153846034, 0.2871794871794871584, 0.2884615384615384914 ),
 .UNSPECIFIED. ) 
 CURVE ( )  GEOMETRIC_REPRESENTATION_ITEM ( )  RATIONAL_B_SPLINE_CURVE ( ( 0.9755282581475768211, 0.9755282581475768211, 1.000000000000000000, 0.9510565162951535312, 1.000000000000000000, 0.9510565162951535312, 1.000000000000000000, 0.9510565162951535312, 1.000000000000000000, 0.9510565162951535312, 1.000000000000000000, 0.9755282581475762660, 0.9755282581475768211 ) ) 
 REPRESENTATION_ITEM ( '' )  );
#4062=CARTESIAN_POINT ( 'NONE',  ( -33.58253175000000113, 51.02500000273119696, -10.91162601494193218 ) ) ;
#4063=CARTESIAN_POINT ( 'NONE',  ( -33.58253175000000113, 21.27500000273117209, -10.91162601494193218 ) ) ;
#4077=CARTESIAN_POINT ( 'NONE',  ( -20.75514604977248823, 56.82500000273118701, -28.56700777964554305 ) ) ;
#4092=CARTESIAN_POINT ( 'NONE',  ( -31.78768264672014610, 52.00000000000002842, 7.374898305514709484 ) ) ;
#4093=CARTESIAN_POINT ( 'NONE',  ( 6.486482029760649416E-15, 21.62500000273119483, 35.31076352940723240 ) ) ;
#4098=CARTESIAN_POINT ( 'NONE',  ( 32.50000000000000000, 43.60000000546237686, -10.55989012756945833 ) ) ;
#4104=CARTESIAN_POINT ( 'NONE',  ( 33.58253175000000113, 66.22500000273120691, -10.91162601494193751 ) ) ;
#4110=CARTESIAN_POINT ( 'NONE',  ( -32.50000000000000000, 10.50000000546237544, 0.000000000000000000 ) ) ;
#4120=SURFACE_SIDE_STYLE ('',( #14092 ) ) ;
#4121=CARTESIAN_POINT ( 'NONE',  ( 20.08610463437157279, 33.29999999999999716, -27.64615127144129758 ) ) ;
#4125=CARTESIAN_POINT ( 'NONE',  ( -14.41072458151355917, 67.00000000000004263, 29.41684567868815492 ) ) ;
#4134=CARTESIAN_POINT ( 'NONE',  ( -27.16883889988623935, 39.32500000273118701, 19.73931689729374739 ) ) ;
#4135=CARTESIAN_POINT ( 'NONE',  ( -2.162160676586881955E-15, 6.875000002731180615, -35.31076352940723240 ) ) ;
#4136=CARTESIAN_POINT ( 'NONE',  ( -20.75514604977248112, 55.67500000273119554, 28.56700777964554661 ) ) ;
#4140=CARTESIAN_POINT ( 'NONE',  ( -20.08610463437157989, 64.20000000546238539, -27.64615127144129758 ) ) ;
#4147=CARTESIAN_POINT ( 'NONE',  ( -27.16883889988624290, 43.17500000273118133, -19.73931689729374028 ) ) ;
#4150=CARTESIAN_POINT ( 'NONE',  ( -20.08610463437156923, 30.80000000546237615, 27.64615127144130113 ) ) ;
#4170=DIRECTION ( 'NONE',  ( 0.000000000000000000, 1.000000000000000000, 0.000000000000000000 ) ) ;
#4171=CARTESIAN_POINT ( 'NONE',  ( -20.08610463437157989, 3.699999999999999289, -27.64615127144129758 ) ) ;
#4174=LINE ( 'NONE', #24764, #12905 ) ;
#4176=CARTESIAN_POINT ( 'NONE',  ( 10.37757302488624767, 65.72500000273119269, 31.93888565452638417 ) ) ;
#4177=CARTESIAN_POINT ( 'NONE',  ( 33.58253175000000113, 24.37500000273119838, -4.112674001490185761E-15 ) ) ;
#4178=CARTESIAN_POINT ( 'NONE',  ( -27.16883889988624290, 7.175000002731176885, -19.73931689729374028 ) ) ;
#4184=CARTESIAN_POINT ( 'NONE',  ( -20.08610463437157989, 47.70000000000000995, -27.64615127144129758 ) ) ;
#4189=CARTESIAN_POINT ( 'NONE',  ( 10.37757302488624056, 60.77500000273118275, -31.93888565452638417 ) ) ;
#4194=CARTESIAN_POINT ( 'NONE',  ( -33.58253175000000113, 29.02500000273119340, -10.91162601494193218 ) ) ;
#4216=CARTESIAN_POINT ( 'NONE',  ( 10.37757302488624056, 40.77500000273119696, -31.93888565452638417 ) ) ;
#4222=CARTESIAN_POINT ( 'NONE',  ( -32.50000000000000000, 67.89999999999996305, -10.55989012756945478 ) ) ;
#4232=CARTESIAN_POINT ( 'NONE',  ( 6.486482029760649416E-15, 49.62500000273117706, 35.31076352940723240 ) ) ;
#4233=CARTESIAN_POINT ( 'NONE',  ( 33.58253175000000113, 24.37500000273119838, -4.112674001490185761E-15 ) ) ;
#4237=CARTESIAN_POINT ( 'NONE',  ( 5.779280353836490358E-15, 60.49999999999998579, 32.49999999999999289 ) ) ;
#4247=CARTESIAN_POINT ( 'NONE',  ( 10.37757302488624767, 53.72500000273118559, 31.93888565452638417 ) ) ;
#4261=CARTESIAN_POINT ( 'NONE',  ( -30.93003301939250704, 52.00000000000002842, 10.64619209630807006 ) ) ;
#4262=CARTESIAN_POINT ( 'NONE',  ( -20.75514604977248112, 23.42500000273119909, 28.56700777964554661 ) ) ;
#4264=CARTESIAN_POINT ( 'NONE',  ( 10.04305231718578817, 53.39999999999999147, -30.90933677959249337 ) ) ;
#4267=CARTESIAN_POINT ( 'NONE',  ( 10.04305231718579705, 43.10000000546236265, 30.90933677959248982 ) ) ;
#4273=CARTESIAN_POINT ( 'NONE',  ( -20.75514604977248112, 67.42500000273118133, 28.56700777964554661 ) ) ;
#4279=CARTESIAN_POINT ( 'NONE',  ( 10.37757302488624056, 14.52500000273120051, -31.93888565452638417 ) ) ;
#4288=CARTESIAN_POINT ( 'NONE',  ( -20.08610463437156923, 38.29999999999997584, 27.64615127144130113 ) ) ;
#4292=CARTESIAN_POINT ( 'NONE',  ( 32.50000000000000711, 62.89999999999998437, 10.55989012756945122 ) ) ;
#4301=CARTESIAN_POINT ( 'NONE',  ( 33.58253175000000113, 42.12500000273118417, -4.112674001490185761E-15 ) ) ;
#4302=CARTESIAN_POINT ( 'NONE',  ( -2.162160676586881955E-15, 2.875000002731189941, -35.31076352940723240 ) ) ;
#4303=CARTESIAN_POINT ( 'NONE',  ( 20.75514604977248467, 56.67500000273119554, -28.56700777964554305 ) ) ;
#4306=CARTESIAN_POINT ( 'NONE',  ( -32.50000000000000000, 60.40000000546236691, -10.55989012756945478 ) ) ;
#4309=CARTESIAN_POINT ( 'NONE',  ( -32.50000000000000000, 54.00000000000000711, 0.000000000000000000 ) ) ;
#4310=EDGE_CURVE ( 'NONE', #24744, #25078, #23939, .T. ) ;
#4313=CARTESIAN_POINT ( 'NONE',  ( 33.58253175000000113, 38.47500000273118559, -10.91162601494193751 ) ) ;
#4317=CARTESIAN_POINT ( 'NONE',  ( 20.08610463437158344, 29.20000000546237118, 27.64615127144129403 ) ) ;
#4329=CARTESIAN_POINT ( 'NONE',  ( -27.16883889988624290, 64.92500000273119554, -19.73931689729374028 ) ) ;
#4338=CARTESIAN_POINT ( 'NONE',  ( -32.50000000000000000, 3.899999999999992806, -10.55989012756945478 ) ) ;
#4343=CARTESIAN_POINT ( 'NONE',  ( -33.58253175000000113, 59.22500000273119269, 10.91162601494193929 ) ) ;
#4344=CARTESIAN_POINT ( 'NONE',  ( 27.16883889988624290, 24.17500000273119198, 19.73931689729373673 ) ) ;
#4345=CARTESIAN_POINT ( 'NONE',  ( 33.58253175000000823, 10.27500000273117564, 10.91162601494192863 ) ) ;
#4349=CARTESIAN_POINT ( 'NONE',  ( 20.08610463437157279, 77.80000000546237970, -27.64615127144129758 ) ) ;
#4351=CARTESIAN_POINT ( 'NONE',  ( 20.08610463437158344, 42.69999999999998863, 27.64615127144129403 ) ) ;
#4357=CARTESIAN_POINT ( 'NONE',  ( 6.486482029760649416E-15, 57.87500000273117706, 35.31076352940723240 ) ) ;
#4363=CARTESIAN_POINT ( 'NONE',  ( -20.75514604977248112, 29.42500000273118133, 28.56700777964554661 ) ) ;
#4382=CARTESIAN_POINT ( 'NONE',  ( 33.58253175000000113, 78.22500000273119269, -10.91162601494193751 ) ) ;
#4383=CARTESIAN_POINT ( 'NONE',  ( -10.37757302488623701, 39.77500000273119696, 31.93888565452638417 ) ) ;
#4389=CARTESIAN_POINT ( 'NONE',  ( 6.277390505771533514E-15, 64.50000000000000000, 34.17252228774368916 ) ) ;
#4395=CARTESIAN_POINT ( 'NONE',  ( -33.58253175000000113, 77.37500000273118417, 0.000000000000000000 ) ) ;
#4400=CARTESIAN_POINT ( 'NONE',  ( -27.16883889988623935, 51.32500000273120122, 19.73931689729374739 ) ) ;
#4401=CARTESIAN_POINT ( 'NONE',  ( -10.37757302488623701, 21.77500000273117919, 31.93888565452638417 ) ) ;
#4410=EDGE_CURVE ( 'NONE', #13108, #17050, #12146, .T. ) ;
#4413=CARTESIAN_POINT ( 'NONE',  ( 26.29305231718579350, 66.80000000000001137, 19.10302069950537529 ) ) ;
#4424=CARTESIAN_POINT ( 'NONE',  ( 20.75514604977249178, 64.07500000273120122, 28.56700777964553950 ) ) ;
#4427=LINE ( 'NONE', #12145, #21596 ) ;
#4431=CARTESIAN_POINT ( 'NONE',  ( -20.75514604977248112, 19.42500000273117777, 28.56700777964554661 ) ) ;
#4433=CARTESIAN_POINT ( 'NONE',  ( 32.50000000000000711, 55.40000000546238113, 10.55989012756945122 ) ) ;
#4436=CARTESIAN_POINT ( 'NONE',  ( -10.04305231718578462, 42.90000000546238823, 30.90933677959249337 ) ) ;
#4441=CARTESIAN_POINT ( 'NONE',  ( -10.37757302488624411, 66.72500000273116427, -31.93888565452638417 ) ) ;
#4447=CARTESIAN_POINT ( 'NONE',  ( 10.37757302488624056, 12.52500000273119873, -31.93888565452638417 ) ) ;
#4458=CARTESIAN_POINT ( 'NONE',  ( 32.50000000000000000, 27.00000000000001066, -3.980102097228898626E-15 ) ) ;
#4459=ADVANCED_FACE ( 'NONE', ( #3922 ), #12325, .T. ) ;
#4463=CARTESIAN_POINT ( 'NONE',  ( -19.64450058003837185, 66.99999999999998579, 26.34187928026369718 ) ) ;
#4464=AXIS2_PLACEMENT_3D ( 'NONE', #29115, #5619, #16103 ) ;
#4474=CARTESIAN_POINT ( 'NONE',  ( 27.16883889988623935, 38.32500000273118701, -19.73931689729374384 ) ) ;
#4475=CARTESIAN_POINT ( 'NONE',  ( -10.37757302488624411, 4.975000002731183812, -31.93888565452638417 ) ) ;
#4476=CARTESIAN_POINT ( 'NONE',  ( 33.58253175000000823, 56.27500000273117564, 10.91162601494192685 ) ) ;
#4480=CARTESIAN_POINT ( 'NONE',  ( 32.50000000000000000, 59.60000000546236976, -10.55989012756945833 ) ) ;
#4486=CARTESIAN_POINT ( 'NONE',  ( -10.37757302488623701, 35.77500000273118985, 31.93888565452638417 ) ) ;
#4490=CARTESIAN_POINT ( 'NONE',  ( -32.50000000000000000, 24.60000000546236620, 10.55989012756946366 ) ) ;
#4498=CARTESIAN_POINT ( 'NONE',  ( -27.16883889988624290, 66.92500000273119554, -19.73931689729374028 ) ) ;
#4503=VECTOR ( 'NONE', #4606, 1000.000000000000000 ) ;
#4509=CARTESIAN_POINT ( 'NONE',  ( -10.04305231718578462, 4.400000000000001243, 30.90933677959249337 ) ) ;
#4514=CARTESIAN_POINT ( 'NONE',  ( 27.16883889988624290, 61.92500000273119554, 19.73931689729373673 ) ) ;
#4515=CARTESIAN_POINT ( 'NONE',  ( 6.486482029760649416E-15, 21.87500000273118062, 35.31076352940723240 ) ) ;
#4516=CARTESIAN_POINT ( 'NONE',  ( -2.162160676586881955E-15, 12.87500000273117884, -35.31076352940723240 ) ) ;
#4521=CARTESIAN_POINT ( 'NONE',  ( -20.75514604977248823, 4.825000002731186122, -28.56700777964554305 ) ) ;
#4523=CARTESIAN_POINT ( 'NONE',  ( 26.29305231718578995, 43.20000000000000284, -19.10302069950538240 ) ) ;
#4529=CARTESIAN_POINT ( 'NONE',  ( 20.75514604977248467, 60.67500000273118133, -28.56700777964554305 ) ) ;
#4535=CARTESIAN_POINT ( 'NONE',  ( -10.37757302488624411, 32.72500000273119269, -31.93888565452638417 ) ) ;
#4555=CARTESIAN_POINT ( 'NONE',  ( 27.16883889988624290, 44.17500000273118133, 19.73931689729373673 ) ) ;
#4562=CARTESIAN_POINT ( 'NONE',  ( 10.04305231718579705, 60.60000000000000142, 30.90933677959248982 ) ) ;
#4567=CARTESIAN_POINT ( 'NONE',  ( -33.58253175000000113, 77.27500000273117564, -10.91162601494193218 ) ) ;
#4572=CARTESIAN_POINT ( 'NONE',  ( -2.162160676586881955E-15, 50.62500000273118417, -35.31076352940723240 ) ) ;
#4573=CARTESIAN_POINT ( 'NONE',  ( 10.37757302488624767, 23.97500000273118559, 31.93888565452638417 ) ) ;
#4574=ORIENTED_EDGE ( 'NONE', *, *, #21402, .F. ) ;
#4586=CARTESIAN_POINT ( 'NONE',  ( 20.08610463437158344, 66.69999999999998863, 27.64615127144129403 ) ) ;
#4596=CARTESIAN_POINT ( 'NONE',  ( 20.75514604977248467, 64.67500000273118133, -28.56700777964554305 ) ) ;
#4603=CARTESIAN_POINT ( 'NONE',  ( -2.162160676586881955E-15, 20.62500000273119483, -35.31076352940723240 ) ) ;
#4606=DIRECTION ( 'NONE',  ( 0.000000000000000000, 1.000000000000000000, 0.000000000000000000 ) ) ;
#4608=CARTESIAN_POINT ( 'NONE',  ( 6.277390505771533514E-15, 39.00000000546236834, 34.17252228774368916 ) ) ;
#4615=CARTESIAN_POINT ( 'NONE',  ( 33.58253175000000113, 68.22500000273116427, -10.91162601494193751 ) ) ;
#4618=VERTEX_POINT ( 'NONE', #21257 ) ;
#4621=CARTESIAN_POINT ( 'NONE',  ( -27.16883889988624290, 10.92500000273120797, -19.73931689729374028 ) ) ;
#4631=CARTESIAN_POINT ( 'NONE',  ( 26.29305231718578995, 29.19999999999998863, -19.10302069950538240 ) ) ;
#4644=CARTESIAN_POINT ( 'NONE',  ( 33.58253175000000823, 38.02500000273117564, 10.91162601494192863 ) ) ;
#4645=CARTESIAN_POINT ( 'NONE',  ( -27.16883889988623935, 3.575000002731185234, 19.73931689729374739 ) ) ;
#4646=CARTESIAN_POINT ( 'NONE',  ( 6.486482029760648627E-15, 55.87500000273118417, 35.31076352940722529 ) ) ;
#4650=CARTESIAN_POINT ( 'NONE',  ( -10.04305231718579172, 60.10000000546238397, -30.90933677959248982 ) ) ;
#4658=CARTESIAN_POINT ( 'NONE',  ( -10.37757302488623701, 37.77500000273118985, 31.93888565452638417 ) ) ;
#4662=CARTESIAN_POINT ( 'NONE',  ( 6.277390505771533514E-15, 25.00000000546238255, 34.17252228774368916 ) ) ;
#4681=CARTESIAN_POINT ( 'NONE',  ( -32.50000000000000000, 4.099999999999986322, 10.55989012756946366 ) ) ;
#4686=CARTESIAN_POINT ( 'NONE',  ( -10.37757302488624411, 58.72500000273119269, -31.93888565452638417 ) ) ;
#4687=CARTESIAN_POINT ( 'NONE',  ( -27.16883889988624290, 21.17500000273118843, -19.73931689729374028 ) ) ;
#4688=CARTESIAN_POINT ( 'NONE',  ( 33.58253175000000113, 10.47500000273118204, -10.91162601494193751 ) ) ;
#4692=CARTESIAN_POINT ( 'NONE',  ( 33.58253175000000113, 4.225000002731190030, -10.91162601494193751 ) ) ;
#4694=CARTESIAN_POINT ( 'NONE',  ( 20.08610463437157279, 39.30000000000001137, -27.64615127144129758 ) ) ;
#4699=CARTESIAN_POINT ( 'NONE',  ( 10.37757302488624767, 51.97500000273118559, 31.93888565452638417 ) ) ;
#4704=CARTESIAN_POINT ( 'NONE',  ( 27.16883889988623935, 22.32500000273117280, -19.73931689729374384 ) ) ;
#4724=CARTESIAN_POINT ( 'NONE',  ( 33.58253175000000113, 42.37500000273118417, -4.112674001490185761E-15 ) ) ;
#4729=CARTESIAN_POINT ( 'NONE',  ( 32.50000000000000000, 60.99999999999998579, -3.980102097228898626E-15 ) ) ;
#4734=CARTESIAN_POINT ( 'NONE',  ( -33.58253175000000113, 71.47500000273119269, 10.91162601494193929 ) ) ;
#4740=CARTESIAN_POINT ( 'NONE',  ( 33.58253175000000823, 50.02500000273118985, 10.91162601494192863 ) ) ;
#4745=CARTESIAN_POINT ( 'NONE',  ( 20.08610463437157279, 7.800000005462373487, -27.64615127144129758 ) ) ;
#4766=CARTESIAN_POINT ( 'NONE',  ( 33.58253175000000113, 62.37500000273120548, -4.112674001490185761E-15 ) ) ;
#4773=CARTESIAN_POINT ( 'NONE',  ( -2.092463501923844636E-15, 79.49999999999998579, -34.17252228774368916 ) ) ;
#4774=CARTESIAN_POINT ( 'NONE',  ( -27.16883889988623935, 23.32500000273117635, 19.73931689729374739 ) ) ;
#4779=CARTESIAN_POINT ( 'NONE',  ( 6.277390505771533514E-15, 41.00000000546236123, 34.17252228774368916 ) ) ;
#4784=CARTESIAN_POINT ( 'NONE',  ( -33.58253175000000113, 71.12500000273118417, 0.000000000000000000 ) ) ;
#4790=CARTESIAN_POINT ( 'NONE',  ( -20.75514604977248112, 9.425000002731184878, 28.56700777964554661 ) ) ;
#4800=CARTESIAN_POINT ( 'NONE',  ( 6.277390505771533514E-15, 26.50000000000000711, 34.17252228774368916 ) ) ;
#4805=CARTESIAN_POINT ( 'NONE',  ( 20.08610463437157279, 63.30000000000001137, -27.64615127144129758 ) ) ;
#4814=CARTESIAN_POINT ( 'NONE',  ( 6.486482029760649416E-15, 41.62500000273116996, 35.31076352940723240 ) ) ;
#4815=CARTESIAN_POINT ( 'NONE',  ( 10.04305231718578817, 57.39999999999999147, -30.90933677959249337 ) ) ;
#4816=CARTESIAN_POINT ( 'NONE',  ( -10.37757302488623701, 57.77500000273121117, 31.93888565452638417 ) ) ;
#4820=CARTESIAN_POINT ( 'NONE',  ( 32.50000000000000000, 63.50000000546239676, -3.980102097228898626E-15 ) ) ;
#4827=CARTESIAN_POINT ( 'NONE',  ( 27.16883889988624290, 34.17500000273120264, 19.73931689729373673 ) ) ;
#4831=CARTESIAN_POINT ( 'NONE',  ( -20.08610463437157989, 26.20000000546237828, -27.64615127144129758 ) ) ;
#4836=ORIENTED_EDGE ( 'NONE', *, *, #12067, .F. ) ;
#4842=CARTESIAN_POINT ( 'NONE',  ( 33.58253175000000823, 60.02500000273116854, 10.91162601494192685 ) ) ;
#4853=ADVANCED_FACE ( 'NONE', ( #7856 ), #18005, .F. ) ;
#4854=CARTESIAN_POINT ( 'NONE',  ( -33.58253175000000113, 77.27500000273117564, -10.91162601494193218 ) ) ;
#4859=CARTESIAN_POINT ( 'NONE',  ( 33.58253175000000113, 62.22500000273119269, -10.91162601494193751 ) ) ;
#4860=CARTESIAN_POINT ( 'NONE',  ( 20.75514604977249178, 18.07500000273119056, 28.56700777964553950 ) ) ;
#4861=CARTESIAN_POINT ( 'NONE',  ( 27.16883889988623935, 10.57500000273119056, -19.73931689729374384 ) ) ;
#4865=CARTESIAN_POINT ( 'NONE',  ( -27.16883889988623935, 5.325000002731187010, 19.73931689729374739 ) ) ;
#4868=CARTESIAN_POINT ( 'NONE',  ( 26.29305231718579350, 42.79999999999999005, 19.10302069950537529 ) ) ;
#4873=CARTESIAN_POINT ( 'NONE',  ( -33.58253175000000113, 53.47500000273117848, 10.91162601494193929 ) ) ;
#4878=CARTESIAN_POINT ( 'NONE',  ( -20.75514604977248823, 24.82500000273117635, -28.56700777964554305 ) ) ;
#4892=CARTESIAN_POINT ( 'NONE',  ( -32.50000000000000000, 17.89999999999998437, -10.55989012756945478 ) ) ;
#4899=CARTESIAN_POINT ( 'NONE',  ( 10.37757302488624767, 43.97500000273117848, 31.93888565452638417 ) ) ;
#4904=CARTESIAN_POINT ( 'NONE',  ( -20.08610463437157989, 59.70000000000000284, -27.64615127144129758 ) ) ;
#4909=CARTESIAN_POINT ( 'NONE',  ( 33.58253175000000113, 76.37500000273118417, -4.112674001490185761E-15 ) ) ;
#4914=CARTESIAN_POINT ( 'NONE',  ( 33.58253175000000823, 46.02500000273118275, 10.91162601494192863 ) ) ;
#4919=CARTESIAN_POINT ( 'NONE',  ( -10.04305231718579172, 2.100000005462371533, -30.90933677959248982 ) ) ;
#4937=CARTESIAN_POINT ( 'NONE',  ( 33.58253175000000113, 60.37500000273120548, -4.112674001490185761E-15 ) ) ;
#4944=CARTESIAN_POINT ( 'NONE',  ( -10.37757302488624411, 12.72500000273117671, -31.93888565452638417 ) ) ;
#4950=CARTESIAN_POINT ( 'NONE',  ( 10.04305231718579705, 35.10000000546238397, 30.90933677959248982 ) ) ;
#4951=CARTESIAN_POINT ( 'NONE',  ( -20.08610463437156923, 66.29999999999999716, 27.64615127144130113 ) ) ;
#4957=CARTESIAN_POINT ( 'NONE',  ( 10.37757302488624056, 60.52500000273118275, -31.93888565452638417 ) ) ;
#4963=CARTESIAN_POINT ( 'NONE',  ( -27.16883889988623935, 9.325000002731190563, 19.73931689729374739 ) ) ;
#4974=CARTESIAN_POINT ( 'NONE',  ( -26.29305231718578995, 52.70000000546236407, 19.10302069950538595 ) ) ;
#4976=CARTESIAN_POINT ( 'NONE',  ( 32.50000000000000000, 31.00000000000001421, -3.980102097228898626E-15 ) ) ;
#4980=CARTESIAN_POINT ( 'NONE',  ( -30.28308157046056337, 66.99999999999997158, 13.46430247876124753 ) ) ;
#4987=CARTESIAN_POINT ( 'NONE',  ( -27.16883889988623935, 35.32500000273118701, 19.73931689729374739 ) ) ;
#4988=CARTESIAN_POINT ( 'NONE',  ( 32.50000000000000000, 57.10000000000000142, -10.55989012756945833 ) ) ;
#4992=CARTESIAN_POINT ( 'NONE',  ( -26.29305231718578995, 60.70000000546237118, 19.10302069950538595 ) ) ;
#4998=CARTESIAN_POINT ( 'NONE',  ( -33.58253175000000113, 35.27500000273120406, -10.91162601494193218 ) ) ;
#5002=CARTESIAN_POINT ( 'NONE',  ( -20.08610463437157989, 22.20000000546238184, -27.64615127144129758 ) ) ;
#5013=CARTESIAN_POINT ( 'NONE',  ( -10.37757302488623701, 61.52500000273118985, 31.93888565452638417 ) ) ;
#5023=CARTESIAN_POINT ( 'NONE',  ( 20.75514604977249178, 74.07500000273120122, 28.56700777964553950 ) ) ;
#5028=CARTESIAN_POINT ( 'NONE',  ( -10.37757302488624411, 52.72500000273121401, -31.93888565452638417 ) ) ;
#5029=CARTESIAN_POINT ( 'NONE',  ( -27.16883889988623935, 19.57500000273119767, 19.73931689729374739 ) ) ;
#5030=CARTESIAN_POINT ( 'NONE',  ( -33.58253175000000113, 1.375000002731191495, 0.000000000000000000 ) ) ;
#5035=CARTESIAN_POINT ( 'NONE',  ( 6.486482029760649416E-15, 5.625000002731175286, 35.31076352940723240 ) ) ;
#5036=CARTESIAN_POINT ( 'NONE',  ( 33.36402495954516212, 51.99999999999999289, -0.4025740098922445664 ) ) ;
#5043=CARTESIAN_POINT ( 'NONE',  ( -27.16883889988624290, 55.17500000273119554, -19.73931689729374028 ) ) ;
#5049=CARTESIAN_POINT ( 'NONE',  ( 20.75514604977249178, 23.82500000273118701, 28.56700777964553950 ) ) ;
#5062=CARTESIAN_POINT ( 'NONE',  ( 10.04305231718579705, 18.59999999999999076, 30.90933677959248982 ) ) ;
#5069=CARTESIAN_POINT ( 'NONE',  ( -33.58253175000000113, 77.12500000273118417, 0.000000000000000000 ) ) ;
#5070=CARTESIAN_POINT ( 'NONE',  ( 27.16883889988624290, 36.17500000273120264, 19.73931689729373673 ) ) ;
#5076=CARTESIAN_POINT ( 'NONE',  ( 10.04305231718578817, 61.39999999999999858, -30.90933677959249337 ) ) ;
#5081=CARTESIAN_POINT ( 'NONE',  ( 33.58253175000000113, 70.37500000273121259, -4.112674001490185761E-15 ) ) ;
#5083=CARTESIAN_POINT ( 'NONE',  ( -27.16883889988623935, 65.57500000273118701, 19.73931689729374739 ) ) ;
#5087=CARTESIAN_POINT ( 'NONE',  ( -20.75514604977248112, 45.42500000273119554, 28.56700777964554661 ) ) ;
#5090=CARTESIAN_POINT ( 'NONE',  ( 0.000000000000000000, 52.00000000000000711, 0.000000000000000000 ) ) ;
#5091=CARTESIAN_POINT ( 'NONE',  ( -20.08610463437156923, 6.800000005462376151, 27.64615127144130113 ) ) ;
#5111=CARTESIAN_POINT ( 'NONE',  ( -33.58253175000000113, 55.47500000273119980, 10.91162601494193929 ) ) ;
#5117=CARTESIAN_POINT ( 'NONE',  ( 6.277390505771533514E-15, 76.50000000000001421, 34.17252228774368916 ) ) ;
#5118=CARTESIAN_POINT ( 'NONE',  ( -10.37757302488623701, 15.52500000273120051, 31.93888565452638417 ) ) ;
#5123=CARTESIAN_POINT ( 'NONE',  ( 10.04305231718579705, 37.10000000546239107, 30.90933677959248982 ) ) ;
#5129=CARTESIAN_POINT ( 'NONE',  ( 6.486482029760649416E-15, 61.62500000273118417, 35.31076352940723240 ) ) ;
#5134=CARTESIAN_POINT ( 'NONE',  ( -10.37757302488623701, 5.525000002731192517, 31.93888565452638417 ) ) ;
#5144=CARTESIAN_POINT ( 'NONE',  ( -32.50000000000000000, 30.10000000000000853, 10.55989012756946366 ) ) ;
#5152=AXIS2_PLACEMENT_3D ( 'NONE', #1928, #4170, #32809 ) ;
#5156=CARTESIAN_POINT ( 'NONE',  ( 10.28315354913682356, 66.99999999999998579, -31.56665548893539963 ) ) ;
#5158=CARTESIAN_POINT ( 'NONE',  ( -27.16883889988623935, 33.32500000273118701, 19.73931689729374739 ) ) ;
#5163=CARTESIAN_POINT ( 'NONE',  ( -32.50000000000000000, 54.50000000546238965, 0.000000000000000000 ) ) ;
#5172=CARTESIAN_POINT ( 'NONE',  ( -33.58253175000000113, 33.37500000273117706, 0.000000000000000000 ) ) ;
#5177=CARTESIAN_POINT ( 'NONE',  ( -26.29305231718579350, 22.30000000546237970, -19.10302069950537884 ) ) ;
#5188=CARTESIAN_POINT ( 'NONE',  ( -33.58253175000000113, 63.02500000273118985, -10.91162601494193041 ) ) ;
#5189=ADVANCED_FACE ( 'NONE', ( #16766 ), #14188, .F. ) ;
#5198=CARTESIAN_POINT ( 'NONE',  ( -10.37757302488623701, 77.77500000273117564, 31.93888565452638417 ) ) ;
#5203=CARTESIAN_POINT ( 'NONE',  ( -33.58253175000000113, 51.22500000273119269, 10.91162601494193929 ) ) ;
#5204=CARTESIAN_POINT ( 'NONE',  ( -10.37757302488624411, 14.97500000273120691, -31.93888565452638417 ) ) ;
#5205=CARTESIAN_POINT ( 'NONE',  ( -2.162160676586881955E-15, 78.62500000273115575, -35.31076352940723240 ) ) ;
#5209=CARTESIAN_POINT ( 'NONE',  ( -26.29305231718579350, 72.30000000546236549, -19.10302069950537884 ) ) ;
#5215=CARTESIAN_POINT ( 'NONE',  ( -10.37757302488624411, 54.97500000273118559, -31.93888565452638417 ) ) ;
#5220=CARTESIAN_POINT ( 'NONE',  ( -20.75514604977248112, 25.42500000273119198, 28.56700777964554661 ) ) ;
#5235=CARTESIAN_POINT ( 'NONE',  ( -32.50000000000000000, 14.09999999999999254, 10.55989012756946366 ) ) ;
#5243=CARTESIAN_POINT ( 'NONE',  ( 33.58253175000000113, 74.12500000273118417, -4.112674001490185761E-15 ) ) ;
#5244=CARTESIAN_POINT ( 'NONE',  ( -20.75514604977248823, 37.07500000273120122, -28.56700777964554305 ) ) ;
#5249=STYLED_ITEM ( 'NONE', ( #14594 ), #10725 ) ;
#5250=CARTESIAN_POINT ( 'NONE',  ( -10.04305231718579172, 57.60000000000000142, -30.90933677959248982 ) ) ;
#5251=PLANE ( 'NONE',  #30889 ) ;
#5254=CARTESIAN_POINT ( 'NONE',  ( -20.75514604977248112, 75.67500000273118133, 28.56700777964554661 ) ) ;
#5260=CARTESIAN_POINT ( 'NONE',  ( -10.37757302488624411, 42.72500000273119980, -31.93888565452638417 ) ) ;
#5264=CARTESIAN_POINT ( 'NONE',  ( 32.50000000000000000, 7.500000005462373664, -3.980102097228898626E-15 ) ) ;
#5283=CARTESIAN_POINT ( 'NONE',  ( -10.37757302488624411, 52.97500000273118559, -31.93888565452638417 ) ) ;
#5291=CARTESIAN_POINT ( 'NONE',  ( -33.58253175000000113, 15.02500000273120051, -10.91162601494193218 ) ) ;
#5296=CARTESIAN_POINT ( 'NONE',  ( -32.50000000000000000, 36.40000000546236691, -10.55989012756945478 ) ) ;
#5301=CARTESIAN_POINT ( 'NONE',  ( 33.58253175000000113, 60.12500000273117706, -4.112674001490185761E-15 ) ) ;
#5305=CARTESIAN_POINT ( 'NONE',  ( -2.162160676586881955E-15, 4.625000002731192161, -35.31076352940723240 ) ) ;
#5317=CARTESIAN_POINT ( 'NONE',  ( 10.04305231718578817, 21.39999999999998792, -30.90933677959249337 ) ) ;
#5321=CARTESIAN_POINT ( 'NONE',  ( -32.98389303421630103, 66.99999999999998579, -5.656568564006192013 ) ) ;
#5327=CARTESIAN_POINT ( 'NONE',  ( -11.64495469945077311, 66.99999999999998579, -31.50463004621152763 ) ) ;
#5329=CARTESIAN_POINT ( 'NONE',  ( 33.58253175000000113, 34.12500000273117706, -4.112674001490185761E-15 ) ) ;
#5334=CARTESIAN_POINT ( 'NONE',  ( 32.50000000000000000, 57.60000000546237686, -10.55989012756945833 ) ) ;
#5342=CARTESIAN_POINT ( 'NONE',  ( -27.16883889988623935, 27.57500000273117990, 19.73931689729374739 ) ) ;
#5344=ORIENTED_EDGE ( 'NONE', *, *, #32784, .T. ) ;
#5346=CARTESIAN_POINT ( 'NONE',  ( 10.04305231718578817, 15.90000000546236336, -30.90933677959249337 ) ) ;
#5356=CARTESIAN_POINT ( 'NONE',  ( 33.58253175000000113, 64.12500000273118417, -4.112674001490185761E-15 ) ) ;
#5366=CARTESIAN_POINT ( 'NONE',  ( -2.162160676586881955E-15, 74.87500000273116996, -35.31076352940723240 ) ) ;
#5370=CARTESIAN_POINT ( 'NONE',  ( -2.162160676586881955E-15, 52.62500000273117706, -35.31076352940723240 ) ) ;
#5371=CARTESIAN_POINT ( 'NONE',  ( -20.75514604977248823, 19.07500000273118701, -28.56700777964554305 ) ) ;
#5372=CARTESIAN_POINT ( 'NONE',  ( 33.58253175000000113, 2.375000002731192161, -4.112674001490185761E-15 ) ) ;
#5378=CARTESIAN_POINT ( 'NONE',  ( 32.50000000000000711, 73.40000000546234560, 10.55989012756945122 ) ) ;
#5379=CARTESIAN_POINT ( 'NONE',  ( 33.37605761044780905, 52.00000000000002132, 0.2721180500512087597 ) ) ;
#5386=CARTESIAN_POINT ( 'NONE',  ( -33.58253175000000113, 51.47500000273118559, 10.91162601494193929 ) ) ;
#5391=CARTESIAN_POINT ( 'NONE',  ( 33.58253175000000113, 26.12500000273119838, -4.112674001490185761E-15 ) ) ;
#5405=CARTESIAN_POINT ( 'NONE',  ( -32.50000000000000000, 60.09999999999999432, 10.55989012756946366 ) ) ;
#5406=CARTESIAN_POINT ( 'NONE',  ( 32.50000000000000000, 15.09999999999998899, -10.55989012756945833 ) ) ;
#5412=CARTESIAN_POINT ( 'NONE',  ( 20.75514604977248467, 72.42500000273119554, -28.56700777964554305 ) ) ;
#5413=CARTESIAN_POINT ( 'NONE',  ( 10.37757302488624767, 37.97500000273119980, 31.93888565452638417 ) ) ;
#5419=CARTESIAN_POINT ( 'NONE',  ( 20.08610463437158344, 52.69999999999998863, 27.64615127144129403 ) ) ;
#5424=CARTESIAN_POINT ( 'NONE',  ( -27.16883889988623935, 75.57500000273118701, 19.73931689729374739 ) ) ;
#5425=CARTESIAN_POINT ( 'NONE',  ( -20.08610463437156923, 62.29999999999998295, 27.64615127144130113 ) ) ;
#5429=CARTESIAN_POINT ( 'NONE',  ( 10.37757302488624056, 40.52500000273119696, -31.93888565452638417 ) ) ;
#5431=EDGE_LOOP ( 'NONE', ( #9267, #30782, #18319, #8412 ) ) ;
#5434=CARTESIAN_POINT ( 'NONE',  ( 32.50000000000000000, 3.500000005462383434, -3.980102097228898626E-15 ) ) ;
#5453=CARTESIAN_POINT ( 'NONE',  ( -10.37757302488623701, 55.77500000273121117, 31.93888565452638417 ) ) ;
#5459=CARTESIAN_POINT ( 'NONE',  ( 6.277390505771533514E-15, 74.50000000000000000, 34.17252228774368916 ) ) ;
#5460=CARTESIAN_POINT ( 'NONE',  ( 27.16883889988623935, 16.32500000273116925, -19.73931689729374384 ) ) ;
#5464=CARTESIAN_POINT ( 'NONE',  ( 20.08610463437158344, 37.20000000546237118, 27.64615127144129403 ) ) ;
#5469=CARTESIAN_POINT ( 'NONE',  ( -10.37757302488623701, 63.52500000273118985, 31.93888565452638417 ) ) ;
#5475=CARTESIAN_POINT ( 'NONE',  ( -33.58253175000000113, 5.125000002731180615, 0.000000000000000000 ) ) ;
#5486=CARTESIAN_POINT ( 'NONE',  ( -26.29305231718578995, 24.19999999999998508, 19.10302069950538595 ) ) ;
#5497=CARTESIAN_POINT ( 'NONE',  ( -19.22940031075258105, 52.00000000000002132, 26.85591229561304161 ) ) ;
#5498=CARTESIAN_POINT ( 'NONE',  ( -27.16883889988623935, 37.32500000273118701, 19.73931689729374739 ) ) ;
#5500=CARTESIAN_POINT ( 'NONE',  ( 31.04172217648528687, 52.00000000000000711, 12.81397374188273908 ) ) ;
#5504=CARTESIAN_POINT ( 'NONE',  ( 6.277390505771533514E-15, 55.00000000546239676, 34.17252228774368916 ) ) ;
#5510=CARTESIAN_POINT ( 'NONE',  ( 10.37757302488624767, 29.97500000273119269, 31.93888565452638417 ) ) ;
#5514=CARTESIAN_POINT ( 'NONE',  ( 10.04305231718578817, 17.90000000546236691, -30.90933677959249337 ) ) ;
#5526=CARTESIAN_POINT ( 'NONE',  ( -33.58253175000000113, 59.12500000273116996, 0.000000000000000000 ) ) ;
#5536=CARTESIAN_POINT ( 'NONE',  ( 20.75514604977248467, 74.67500000273118133, -28.56700777964554305 ) ) ;
#5540=CARTESIAN_POINT ( 'NONE',  ( -27.16883889988624290, 54.92500000273118843, -19.73931689729374028 ) ) ;
#5541=CARTESIAN_POINT ( 'NONE',  ( -27.16883889988623935, 15.57500000273119589, 19.73931689729374739 ) ) ;
#5542=CARTESIAN_POINT ( 'NONE',  ( -27.16883889988623935, 5.575000002731187010, 19.73931689729374739 ) ) ;
#5546=CARTESIAN_POINT ( 'NONE',  ( -10.04305231718578462, 74.90000000546235981, 30.90933677959249337 ) ) ;
#5547=CARTESIAN_POINT ( 'NONE',  ( 32.98389303421620866, 52.00000000000003553, 5.656568564006877686 ) ) ;
#5553=CARTESIAN_POINT ( 'NONE',  ( -33.58253175000000113, 47.47500000273119269, 10.91162601494193929 ) ) ;
#5560=CARTESIAN_POINT ( 'NONE',  ( -27.16883889988623935, 15.32500000273116747, 19.73931689729374739 ) ) ;
#5570=CARTESIAN_POINT ( 'NONE',  ( -5.147494310547478413, 64.44874571845313938, 32.49999999999998579 ) ) ;
#5575=CARTESIAN_POINT ( 'NONE',  ( -32.50000000000000000, 16.00000000000000000, 0.000000000000000000 ) ) ;
#5581=CARTESIAN_POINT ( 'NONE',  ( 27.16883889988624290, 73.92500000273120975, 19.73931689729373673 ) ) ;
#5583=CARTESIAN_POINT ( 'NONE',  ( -27.16883889988624290, 39.17500000273120264, -19.73931689729374028 ) ) ;
#5588=CARTESIAN_POINT ( 'NONE',  ( -20.08610463437157989, 51.70000000000000284, -27.64615127144129758 ) ) ;
#5593=CARTESIAN_POINT ( 'NONE',  ( 27.16883889988624290, 68.17500000273118133, 19.73931689729373673 ) ) ;
#5598=CARTESIAN_POINT ( 'NONE',  ( -2.162160676586881955E-15, 42.62500000273119838, -35.31076352940723240 ) ) ;
#5599=FACE_OUTER_BOUND ( 'NONE', #812, .T. ) ;
#5604=CARTESIAN_POINT ( 'NONE',  ( 20.08610463437158344, 3.200000005462373398, 27.64615127144129403 ) ) ;
#5619=DIRECTION ( 'NONE',  ( 0.000000000000000000, 1.000000000000000000, 0.000000000000000000 ) ) ;
#5623=CARTESIAN_POINT ( 'NONE',  ( 20.75514604977249178, 58.07500000273117990, 28.56700777964553950 ) ) ;
#5629=CARTESIAN_POINT ( 'NONE',  ( 32.50000000000000000, 73.09999999999996589, -10.55989012756945833 ) ) ;
#5630=CARTESIAN_POINT ( 'NONE',  ( 27.16883889988624290, 11.92500000273118133, 19.73931689729373673 ) ) ;
#5638=CARTESIAN_POINT ( 'NONE',  ( 33.58253175000000823, 60.02500000273116854, 10.91162601494192863 ) ) ;
#5643=CARTESIAN_POINT ( 'NONE',  ( 20.75514604977249178, 3.825000002731188786, 28.56700777964553950 ) ) ;
#5651=CARTESIAN_POINT ( 'NONE',  ( -32.50000000000000000, 52.50000000546238255, 0.000000000000000000 ) ) ;
#5654=CARTESIAN_POINT ( 'NONE',  ( 26.29305231718579350, 24.80000000000000426, 19.10302069950537529 ) ) ;
#5658=CARTESIAN_POINT ( 'NONE',  ( -33.25271216035369548, 66.99999999999997158, -3.649504031948202165 ) ) ;
#5666=CARTESIAN_POINT ( 'NONE',  ( 20.82183453687062169, 66.99999999999997158, -25.59657189324412485 ) ) ;
#5667=CARTESIAN_POINT ( 'NONE',  ( -27.48632242023157701, 51.99999999999999289, 17.98641839608171011 ) ) ;
#5668=CARTESIAN_POINT ( 'NONE',  ( 10.37757302488624767, 31.72500000273119269, 31.93888565452638417 ) ) ;
#5669=CARTESIAN_POINT ( 'NONE',  ( -26.29305231718578995, 56.70000000546236407, 19.10302069950538595 ) ) ;
#5675=CARTESIAN_POINT ( 'NONE',  ( 20.08610463437157279, 55.80000000546236549, -27.64615127144129758 ) ) ;
#5682=CARTESIAN_POINT ( 'NONE',  ( -33.58253175000000113, 25.47500000273118914, 10.91162601494193929 ) ) ;
#5686=CARTESIAN_POINT ( 'NONE',  ( -26.29305231718578995, 18.70000000546238894, 19.10302069950538595 ) ) ;
#5697=CARTESIAN_POINT ( 'NONE',  ( 33.58253175000000113, 54.12500000273119838, -4.112674001490185761E-15 ) ) ;
#5702=CARTESIAN_POINT ( 'NONE',  ( -5.147494310547377161, 66.05125428700924317, -32.50000000000002132 ) ) ;
#5703=CARTESIAN_POINT ( 'NONE',  ( 0.000000000000000000, 52.00000000000000711, 32.50000000000000000 ) ) ;
#5707=CARTESIAN_POINT ( 'NONE',  ( 33.58253175000000113, 68.47500000273119269, -10.91162601494193751 ) ) ;
#5708=ORIENTED_EDGE ( 'NONE', *, *, #30107, .T. ) ;
#5711=EDGE_CURVE ( 'NONE', #31633, #32671, #22703, .T. ) ;
#5712=CARTESIAN_POINT ( 'NONE',  ( 27.16883889988624290, 51.92500000273118843, 19.73931689729373673 ) ) ;
#5713=CARTESIAN_POINT ( 'NONE',  ( -10.37757302488623701, 13.77500000273117209, 31.93888565452638417 ) ) ;
#5714=CARTESIAN_POINT ( 'NONE',  ( -20.75514604977248112, 5.675000002731189319, 28.56700777964554661 ) ) ;
#5718=CARTESIAN_POINT ( 'NONE',  ( -2.092463501923844636E-15, 76.00000000546235412, -34.17252228774368916 ) ) ;
#5719=CARTESIAN_POINT ( 'NONE',  ( 6.725304478054956903, 51.99999999999999289, -31.94333337441925025 ) ) ;
#5725=CARTESIAN_POINT ( 'NONE',  ( 10.37757302488624767, 49.97500000273117848, 31.93888565452638417 ) ) ;
#5730=CARTESIAN_POINT ( 'NONE',  ( -2.162160676586881955E-15, 16.62500000273120548, -35.31076352940723240 ) ) ;
#5737=DIRECTION ( 'NONE',  ( 0.000000000000000000, 1.000000000000000000, 0.000000000000000000 ) ) ;
#5744=CARTESIAN_POINT ( 'NONE',  ( 20.08610463437157279, 7.300000000000001599, -27.64615127144129758 ) ) ;
#5750=CARTESIAN_POINT ( 'NONE',  ( 10.37757302488624767, 71.72500000273117848, 31.93888565452638417 ) ) ;
#5751=CARTESIAN_POINT ( 'NONE',  ( -10.37757302488623701, 37.77500000273118985, 31.93888565452638417 ) ) ;
#5756=CARTESIAN_POINT ( 'NONE',  ( 20.08610463437158344, 54.69999999999998863, 27.64615127144129403 ) ) ;
#5762=CARTESIAN_POINT ( 'NONE',  ( 27.16883889988623935, 64.57500000273118701, -19.73931689729374384 ) ) ;
#5766=VERTEX_POINT ( 'NONE', #29754 ) ;
#5767=CARTESIAN_POINT ( 'NONE',  ( -33.58253175000000113, 35.02500000273118275, -10.91162601494193218 ) ) ;
#5769=ORIENTED_EDGE ( 'NONE', *, *, #33051, .T. ) ;
#5784=CARTESIAN_POINT ( 'NONE',  ( 5.779280353836490358E-15, 55.00000000546238965, 32.49999999999999289 ) ) ;
#5788=CARTESIAN_POINT ( 'NONE',  ( 33.58253175000000113, 54.37500000273119838, -4.112674001490185761E-15 ) ) ;
#5794=CARTESIAN_POINT ( 'NONE',  ( 32.50000000000000000, 71.00000000000000000, -3.980102097228898626E-15 ) ) ;
#5795=CARTESIAN_POINT ( 'NONE',  ( 27.16883889988624290, 5.925000002731190207, 19.73931689729373673 ) ) ;
#5799=DIRECTION ( 'NONE',  ( 0.000000000000000000, 1.000000000000000000, 0.000000000000000000 ) ) ;
#5806=CARTESIAN_POINT ( 'NONE',  ( 10.37757302488624767, 57.72500000273118559, 31.93888565452638417 ) ) ;
#5811=CARTESIAN_POINT ( 'NONE',  ( -27.16883889988623935, 5.325000002731187010, 19.73931689729374739 ) ) ;
#5822=CARTESIAN_POINT ( 'NONE',  ( 20.08610463437158344, 22.70000000000000995, 27.64615127144129403 ) ) ;
#5834=CARTESIAN_POINT ( 'NONE',  ( -20.82183453687059682, 52.00000000000002842, 25.59657189324412130 ) ) ;
#5836=CARTESIAN_POINT ( 'NONE',  ( 27.16883889988624290, 27.92500000273119554, 19.73931689729373673 ) ) ;
#5837=CARTESIAN_POINT ( 'NONE',  ( 20.08610463437158344, 64.70000000000001705, 27.64615127144129403 ) ) ;
#5839=CARTESIAN_POINT ( 'NONE',  ( 26.29305231718579350, 60.80000000000000426, 19.10302069950537529 ) ) ;
#5841=CARTESIAN_POINT ( 'NONE',  ( -10.04305231718578462, 56.90000000546240244, 30.90933677959249337 ) ) ;
#5850=CARTESIAN_POINT ( 'NONE',  ( 20.08610463437158344, 17.20000000546236762, 27.64615127144129403 ) ) ;
#5858=CYLINDRICAL_SURFACE ( 'NONE', #22003, 32.50000000000000000 ) ;
#5861=CARTESIAN_POINT ( 'NONE',  ( -27.16883889988623935, 53.32500000273120122, 19.73931689729374739 ) ) ;
#5865=CARTESIAN_POINT ( 'NONE',  ( -32.50000000000000000, 66.60000000546237686, 10.55989012756946366 ) ) ;
#5869=CARTESIAN_POINT ( 'NONE',  ( -20.75514604977248112, 69.67500000273119554, 28.56700777964554661 ) ) ;
#5875=CARTESIAN_POINT ( 'NONE',  ( -33.58253175000000113, 45.02500000273117564, -10.91162601494193218 ) ) ;
#5876=CARTESIAN_POINT ( 'NONE',  ( 33.58253175000000113, 8.475000002731185589, -10.91162601494193751 ) ) ;
#5877=CARTESIAN_POINT ( 'NONE',  ( 20.75514604977248467, 64.67500000273116711, -28.56700777964554305 ) ) ;
#5882=CARTESIAN_POINT ( 'NONE',  ( -20.08610463437157989, 72.20000000546237118, -27.64615127144129758 ) ) ;
#5889=CARTESIAN_POINT ( 'NONE',  ( -20.75514604977248112, 49.67500000273118133, 28.56700777964554661 ) ) ;
#5894=CARTESIAN_POINT ( 'NONE',  ( -10.37757302488624411, 20.72500000273118204, -31.93888565452638417 ) ) ;
#5906=CARTESIAN_POINT ( 'NONE',  ( -26.29305231718579350, 63.80000000000001137, -19.10302069950537884 ) ) ;
#5910=CARTESIAN_POINT ( 'NONE',  ( 20.08610463437157279, 9.299999999999998934, -27.64615127144129758 ) ) ;
#5916=CARTESIAN_POINT ( 'NONE',  ( -33.58253175000000113, 73.22500000273117848, 10.91162601494193929 ) ) ;
#5917=CARTESIAN_POINT ( 'NONE',  ( -33.58253175000000113, 27.27500000273119340, -10.91162601494193218 ) ) ;
#5918=CARTESIAN_POINT ( 'NONE',  ( 10.37757302488624056, 18.77500000273117564, -31.93888565452638417 ) ) ;
#5924=CARTESIAN_POINT ( 'NONE',  ( -26.29305231718579350, 55.80000000000000426, -19.10302069950537884 ) ) ;
#5930=CARTESIAN_POINT ( 'NONE',  ( 6.486482029760649416E-15, 63.87500000273119127, 35.31076352940723240 ) ) ;
#5931=CARTESIAN_POINT ( 'NONE',  ( -10.04305231718579172, 61.60000000000000142, -30.90933677959248982 ) ) ;
#5935=CARTESIAN_POINT ( 'NONE',  ( 6.486482029760649416E-15, 39.62500000273117706, 35.31076352940723240 ) ) ;
#5951=CARTESIAN_POINT ( 'NONE',  ( 10.04305231718579705, 53.10000000546237686, 30.90933677959248982 ) ) ;
#5955=CARTESIAN_POINT ( 'NONE',  ( 10.37757302488624056, 50.77500000273120406, -31.93888565452638417 ) ) ;
#5962=CARTESIAN_POINT ( 'NONE',  ( -32.50000000000000000, 76.10000000000002274, 10.55989012756946366 ) ) ;
#5963=CARTESIAN_POINT ( 'NONE',  ( -27.16883889988624290, 8.925000002731206195, -19.73931689729374028 ) ) ;
#5972=ORIENTED_EDGE ( 'NONE', *, *, #30747, .F. ) ;
#5973=CARTESIAN_POINT ( 'NONE',  ( 20.75514604977249178, 55.82500000273119412, 28.56700777964553950 ) ) ;
#5974=ORIENTED_EDGE ( 'NONE', *, *, #8471, .T. ) ;
#5977=CARTESIAN_POINT ( 'NONE',  ( -27.16883889988623935, 1.325000002731183013, 19.73931689729374739 ) ) ;
#5985=CARTESIAN_POINT ( 'NONE',  ( -32.50000000000000000, 21.90000000000000924, -10.55989012756945478 ) ) ;
#5996=CARTESIAN_POINT ( 'NONE',  ( 12.90513655866702081, 52.00000000000000711, 31.00393344628893288 ) ) ;
#5997=CARTESIAN_POINT ( 'NONE',  ( 33.58253175000000823, 30.02500000273118985, 10.91162601494192863 ) ) ;
#6003=CARTESIAN_POINT ( 'NONE',  ( -10.04305231718579172, 46.10000000546236976, -30.90933677959248982 ) ) ;
#6008=CARTESIAN_POINT ( 'NONE',  ( -20.75514604977248823, 74.82500000273115859, -28.56700777964554305 ) ) ;
#6013=CARTESIAN_POINT ( 'NONE',  ( 32.50000000000000000, 15.60000000546238930, -10.55989012756945833 ) ) ;
#6028=PLANE ( 'NONE',  #24267 ) ;
#6029=CARTESIAN_POINT ( 'NONE',  ( 20.75514604977248467, 68.67500000273119554, -28.56700777964554305 ) ) ;
#6034=CARTESIAN_POINT ( 'NONE',  ( -27.16883889988624290, 44.92500000273118133, -19.73931689729374028 ) ) ;
#6035=CARTESIAN_POINT ( 'NONE',  ( 10.37757302488624767, 9.975000002731201576, 31.93888565452638417 ) ) ;
#6036=CARTESIAN_POINT ( 'NONE',  ( -33.58253175000000113, 65.27500000273117564, -10.91162601494193041 ) ) ;
#6040=CARTESIAN_POINT ( 'NONE',  ( 32.50000000000000000, 65.50000000546239676, -3.980102097228898626E-15 ) ) ;
#6045=CARTESIAN_POINT ( 'NONE',  ( 27.16883889988624290, 48.17500000273118843, 19.73931689729373673 ) ) ;
#6050=CARTESIAN_POINT ( 'NONE',  ( -33.58253175000000113, 15.02500000273120051, -10.91162601494193218 ) ) ;
#6065=CARTESIAN_POINT ( 'NONE',  ( 32.50000000000000000, 11.09999999999999964, -10.55989012756945833 ) ) ;
#6071=CARTESIAN_POINT ( 'NONE',  ( 10.37757302488624767, 69.72500000273117848, 31.93888565452638417 ) ) ;
#6072=CARTESIAN_POINT ( 'NONE',  ( 33.58253175000000823, 32.27500000273117564, 10.91162601494192863 ) ) ;
#6073=CARTESIAN_POINT ( 'NONE',  ( 33.58253175000000113, 14.37500000273118950, -4.112674001490185761E-15 ) ) ;
#6081=CARTESIAN_POINT ( 'NONE',  ( 20.08610463437157279, 45.29999999999999005, -27.64615127144129758 ) ) ;
#6082=CARTESIAN_POINT ( 'NONE',  ( 5.779280353836490358E-15, 62.50000000000000000, 32.49999999999999289 ) ) ;
#6087=CARTESIAN_POINT ( 'NONE',  ( 20.75514604977248467, 66.67500000273119554, -28.56700777964554305 ) ) ;
#6092=CARTESIAN_POINT ( 'NONE',  ( -27.16883889988623935, 35.32500000273118701, 19.73931689729374739 ) ) ;
#6094=VECTOR ( 'NONE', #20087, 1000.000000000000000 ) ;
#6097=CARTESIAN_POINT ( 'NONE',  ( -20.08610463437156923, 60.80000000546238681, 27.64615127144130113 ) ) ;
#6114=CARTESIAN_POINT ( 'NONE',  ( 33.58253175000000113, 46.47500000273118559, -10.91162601494193751 ) ) ;
#6121=CARTESIAN_POINT ( 'NONE',  ( 26.29305231718579350, 70.80000000000001137, 19.10302069950537529 ) ) ;
#6122=CARTESIAN_POINT ( 'NONE',  ( -33.58253175000000113, 9.125000002731184168, 0.000000000000000000 ) ) ;
#6131=CARTESIAN_POINT ( 'NONE',  ( 10.37757302488624056, 54.52500000273118275, -31.93888565452638417 ) ) ;
#6160=CARTESIAN_POINT ( 'NONE',  ( 27.16883889988623935, 26.32500000273117635, -19.73931689729374384 ) ) ;
#6161=CARTESIAN_POINT ( 'NONE',  ( 26.29305231718579350, 56.80000000000000426, 19.10302069950537529 ) ) ;
#6162=CARTESIAN_POINT ( 'NONE',  ( 10.04305231718578817, 61.90000000546237402, -30.90933677959249337 ) ) ;
#6166=CARTESIAN_POINT ( 'NONE',  ( 26.29305231718579350, 49.30000000546237970, 19.10302069950537529 ) ) ;
#6172=CARTESIAN_POINT ( 'NONE',  ( 20.75514604977248467, 74.42500000273119554, -28.56700777964554305 ) ) ;
#6177=CARTESIAN_POINT ( 'NONE',  ( 32.50000000000000000, 7.600000005462379526, -10.55989012756945833 ) ) ;
#6186=CARTESIAN_POINT ( 'NONE',  ( 0.000000000000000000, 0.000000000000000000, 0.000000000000000000 ) ) ;
#6196=CARTESIAN_POINT ( 'NONE',  ( 20.75514604977248467, 66.67500000273119554, -28.56700777964554305 ) ) ;
#6200=DIRECTION ( 'NONE',  ( 0.000000000000000000, 1.000000000000000000, 0.000000000000000000 ) ) ;
#6201=CARTESIAN_POINT ( 'NONE',  ( 33.58253175000000113, 46.22500000273119269, -10.91162601494193751 ) ) ;
#6202=CARTESIAN_POINT ( 'NONE',  ( 27.16883889988623935, 10.57500000273119056, -19.73931689729374384 ) ) ;
#6203=CARTESIAN_POINT ( 'NONE',  ( -33.58253175000000113, 63.47500000273117848, 10.91162601494193929 ) ) ;
#6207=CARTESIAN_POINT ( 'NONE',  ( 26.29305231718578995, 67.70000000546237118, -19.10302069950538240 ) ) ;
#6211=EDGE_CURVE ( 'NONE', #19609, #9681, #19401, .T. ) ;
#6214=CARTESIAN_POINT ( 'NONE',  ( -33.58253175000000113, 49.37500000273119127, 0.000000000000000000 ) ) ;
#6217=CARTESIAN_POINT ( 'NONE',  ( 32.50000000000000711, 31.40000000546238823, 10.55989012756945122 ) ) ;
#6219=CARTESIAN_POINT ( 'NONE',  ( 33.58253175000000113, 18.12500000273119127, -4.112674001490185761E-15 ) ) ;
#6237=CARTESIAN_POINT ( 'NONE',  ( -10.04305231718579172, 9.599999999999983658, -30.90933677959248982 ) ) ;
#6243=CARTESIAN_POINT ( 'NONE',  ( -10.37757302488624411, 68.72500000273116427, -31.93888565452638417 ) ) ;
#6244=CARTESIAN_POINT ( 'NONE',  ( 20.75514604977248467, 30.67500000273119909, -28.56700777964554305 ) ) ;
#6246=CARTESIAN_POINT ( 'NONE',  ( 27.16883889988623935, 18.57500000273119767, -19.73931689729374384 ) ) ;
#6253=CARTESIAN_POINT ( 'NONE',  ( -32.50000000000000000, 50.09999999999998721, 10.55989012756946366 ) ) ;
#6258=CARTESIAN_POINT ( 'NONE',  ( -10.37757302488623701, 69.77500000273118985, 31.93888565452638417 ) ) ;
#6264=CARTESIAN_POINT ( 'NONE',  ( 27.16883889988624290, 33.92500000273117422, 19.73931689729373673 ) ) ;
#6286=CARTESIAN_POINT ( 'NONE',  ( 33.58253175000000113, 52.37500000273119838, -4.112674001490185761E-15 ) ) ;
#6292=CARTESIAN_POINT ( 'NONE',  ( -10.04305231718579172, 67.59999999999998010, -30.90933677959248982 ) ) ;
#6293=CARTESIAN_POINT ( 'NONE',  ( -27.16883889988624290, 6.925000002731204418, -19.73931689729374028 ) ) ;
#6303=CARTESIAN_POINT ( 'NONE',  ( -33.58253175000000113, 57.12500000273116996, 0.000000000000000000 ) ) ;
#6304=CARTESIAN_POINT ( 'NONE',  ( 10.37757302488624767, 27.97500000273118914, 31.93888565452638417 ) ) ;
#6305=ORIENTED_EDGE ( 'NONE', *, *, #26712, .F. ) ;
#6335=CARTESIAN_POINT ( 'NONE',  ( -27.16883889988624290, 28.92500000273119554, -19.73931689729374028 ) ) ;
#6338=CARTESIAN_POINT ( 'NONE',  ( 5.147494310547481966, 61.44874571845315359, -32.49999999999998579 ) ) ;
#6340=CARTESIAN_POINT ( 'NONE',  ( -32.50000000000000000, 46.50000000546238255, 0.000000000000000000 ) ) ;
#6344=CARTESIAN_POINT ( 'NONE',  ( -27.16883889988623935, 75.32500000273118701, 19.73931689729374739 ) ) ;
#6350=CARTESIAN_POINT ( 'NONE',  ( -10.04305231718579172, 12.10000000546239463, -30.90933677959248982 ) ) ;
#6359=CARTESIAN_POINT ( 'NONE',  ( 32.50000000000000000, 35.10000000000000142, -10.55989012756945833 ) ) ;
#6368=CARTESIAN_POINT ( 'NONE',  ( -27.16883889988623935, 61.57500000273117990, 19.73931689729374739 ) ) ;
#6373=CARTESIAN_POINT ( 'NONE',  ( 27.16883889988624290, 49.92500000273118843, 19.73931689729373673 ) ) ;
#6374=CARTESIAN_POINT ( 'NONE',  ( -10.37757302488624411, 12.97500000273120513, -31.93888565452638417 ) ) ;
#6375=CARTESIAN_POINT ( 'NONE',  ( -27.16883889988623935, 63.57500000273117990, 19.73931689729374739 ) ) ;
#6379=CARTESIAN_POINT ( 'NONE',  ( -10.04305231718579172, 66.10000000546239107, -30.90933677959248982 ) ) ;
#6383=DIRECTION ( 'NONE',  ( -0.8660254037844385966, 0.000000000000000000, 0.5000000000000000000 ) ) ;
#6386=CARTESIAN_POINT ( 'NONE',  ( -33.58253175000000113, 43.47500000273117138, 10.91162601494193929 ) ) ;
#6388=CARTESIAN_POINT ( 'NONE',  ( 6.277390505771533514E-15, 27.00000000546237899, 34.17252228774368916 ) ) ;
#6410=CARTESIAN_POINT ( 'NONE',  ( 26.29305231718579350, 8.800000000000016698, 19.10302069950537529 ) ) ;
#6413=DIRECTION ( 'NONE',  ( 0.000000000000000000, 1.000000000000000000, 0.000000000000000000 ) ) ;
#6416=CARTESIAN_POINT ( 'NONE',  ( 33.58253175000000113, 64.22500000273117848, -10.91162601494193751 ) ) ;
#6417=CARTESIAN_POINT ( 'NONE',  ( 27.16883889988624290, 28.17500000273119554, 19.73931689729373673 ) ) ;
#6418=CARTESIAN_POINT ( 'NONE',  ( -27.16883889988623935, 17.57500000273119767, 19.73931689729374739 ) ) ;
#6425=CARTESIAN_POINT ( 'NONE',  ( -32.50000000000000000, 45.89999999999999858, -10.55989012756945478 ) ) ;
#6429=ORIENTED_EDGE ( 'NONE', *, *, #3604, .T. ) ;
#6430=CARTESIAN_POINT ( 'NONE',  ( 33.58253175000000113, 60.47500000273118559, -10.91162601494193751 ) ) ;
#6436=CARTESIAN_POINT ( 'NONE',  ( 27.16883889988623935, 34.32500000273118701, -19.73931689729374384 ) ) ;
#6438=ORIENTED_EDGE ( 'NONE', *, *, #16640, .F. ) ;
#6457=CARTESIAN_POINT ( 'NONE',  ( 20.75514604977248467, 48.67500000273117422, -28.56700777964554305 ) ) ;
#6464=CARTESIAN_POINT ( 'NONE',  ( -2.092463501923844636E-15, 69.49999999999997158, -34.17252228774368916 ) ) ;
#6476=CARTESIAN_POINT ( 'NONE',  ( -33.58253175000000113, 59.12500000273116996, 0.000000000000000000 ) ) ;
#6477=CARTESIAN_POINT ( 'NONE',  ( -20.75514604977248112, 31.67500000273119909, 28.56700777964554661 ) ) ;
#6490=CARTESIAN_POINT ( 'NONE',  ( -20.75514604977248823, 52.82500000273116569, -28.56700777964554305 ) ) ;
#6502=CARTESIAN_POINT ( 'NONE',  ( 0.000000000000000000, 66.99999999999998579, 0.000000000000000000 ) ) ;
#6505=CARTESIAN_POINT ( 'NONE',  ( -33.58253175000000113, 25.22500000273119625, 10.91162601494193929 ) ) ;
#6510=CARTESIAN_POINT ( 'NONE',  ( 32.50000000000000000, 49.60000000546239818, -10.55989012756945833 ) ) ;
#6512=CARTESIAN_POINT ( 'NONE',  ( -26.29305231718579350, 58.30000000546238681, -19.10302069950537884 ) ) ;
#6516=CARTESIAN_POINT ( 'NONE',  ( -27.16883889988624290, 74.92500000273120975, -19.73931689729374028 ) ) ;
#6518=LINE ( 'NONE', #16989, #8055 ) ;
#6519=EDGE_LOOP ( 'NONE', ( #27199, #16947, #2106, #17327 ) ) ;
#6521=CARTESIAN_POINT ( 'NONE',  ( 20.08610463437157279, 11.80000000546236194, -27.64615127144129758 ) ) ;
#6530=( LENGTH_UNIT ( ) NAMED_UNIT ( * ) SI_UNIT ( .MILLI., .METRE. ) );
#6531=CARTESIAN_POINT ( 'NONE',  ( -20.08610463437157989, 37.70000000000000995, -27.64615127144129758 ) ) ;
#6543=CARTESIAN_POINT ( 'NONE',  ( 6.486482029760649416E-15, 49.62500000273117706, 35.31076352940723240 ) ) ;
#6544=CARTESIAN_POINT ( 'NONE',  ( 10.37757302488624056, 4.775000002731191628, -31.93888565452638417 ) ) ;
#6545=CARTESIAN_POINT ( 'NONE',  ( -33.58253175000000113, 59.47500000273119269, 10.91162601494193929 ) ) ;
#6549=CARTESIAN_POINT ( 'NONE',  ( 32.50000000000000000, 69.60000000546236265, -10.55989012756945833 ) ) ;
#6554=CARTESIAN_POINT ( 'NONE',  ( 10.37757302488624056, 38.77500000273119696, -31.93888565452638417 ) ) ;
#6556=CARTESIAN_POINT ( 'NONE',  ( 32.50000000000000000, 27.60000000546238752, -10.55989012756945833 ) ) ;
#6575=CARTESIAN_POINT ( 'NONE',  ( 26.29305231718578995, 5.199999999999996625, -19.10302069950538240 ) ) ;
#6580=CARTESIAN_POINT ( 'NONE',  ( 27.16883889988624290, 65.92500000273119554, 19.73931689729373673 ) ) ;
#6581=CARTESIAN_POINT ( 'NONE',  ( -2.162160676586881955E-15, 32.87500000273118417, -35.31076352940723240 ) ) ;
#6582=CARTESIAN_POINT ( 'NONE',  ( -20.75514604977248112, 19.67500000273119909, 28.56700777964554661 ) ) ;
#6587=CARTESIAN_POINT ( 'NONE',  ( -26.29305231718579350, 47.79999999999999716, -19.10302069950537884 ) ) ;
#6592=CARTESIAN_POINT ( 'NONE',  ( 33.58253175000000113, 62.37500000273120548, -4.112674001490185761E-15 ) ) ;
#6598=CARTESIAN_POINT ( 'NONE',  ( -10.37757302488623701, 29.52500000273118630, 31.93888565452638417 ) ) ;
#6619=CARTESIAN_POINT ( 'NONE',  ( -20.75514604977248112, 51.67500000273117422, 28.56700777964554661 ) ) ;
#6625=CARTESIAN_POINT ( 'NONE',  ( -10.04305231718578462, 68.40000000000000568, 30.90933677959249337 ) ) ;
#6635=CARTESIAN_POINT ( 'NONE',  ( -10.37757302488624411, 48.72500000273120691, -31.93888565452638417 ) ) ;
#6636=CARTESIAN_POINT ( 'NONE',  ( -27.16883889988624290, 23.17500000273119198, -19.73931689729374028 ) ) ;
#6648=CARTESIAN_POINT ( 'NONE',  ( -25.33181144634176363, 67.00000000000000000, -22.15645287101984096 ) ) ;
#6651=CARTESIAN_POINT ( 'NONE',  ( -20.75514604977248112, 57.42500000273119554, 28.56700777964554661 ) ) ;
#6665=CARTESIAN_POINT ( 'NONE',  ( -1.053607264507113999E-13, 63.00000000546238255, 32.50000000000000711 ) ) ;
#6666=CARTESIAN_POINT ( 'NONE',  ( -32.50000000000000000, 52.00000000000000711, 0.000000000000000000 ) ) ;
#6667=CARTESIAN_POINT ( 'NONE',  ( 33.58253175000000113, 22.12500000273119483, -4.112674001490185761E-15 ) ) ;
#6672=CARTESIAN_POINT ( 'NONE',  ( 20.08610463437157279, 39.80000000546238681, -27.64615127144129758 ) ) ;
#6677=CARTESIAN_POINT ( 'NONE',  ( 33.58253175000000113, 76.12500000273118417, -4.112674001490185761E-15 ) ) ;
#6679=DIRECTION ( 'NONE',  ( 0.000000000000000000, 0.000000000000000000, -1.000000000000000000 ) ) ;
#6682=CARTESIAN_POINT ( 'NONE',  ( -26.29305231718578995, 12.70000000546238361, 19.10302069950538595 ) ) ;
#6691=CARTESIAN_POINT ( 'NONE',  ( -10.04305231718579172, 33.60000000000000142, -30.90933677959248982 ) ) ;
#6706=CARTESIAN_POINT ( 'NONE',  ( -27.16883889988623935, 43.32500000273119412, 19.73931689729374739 ) ) ;
#6707=CARTESIAN_POINT ( 'NONE',  ( -33.58253175000000113, 5.475000002731181148, 10.91162601494193929 ) ) ;
#6708=CARTESIAN_POINT ( 'NONE',  ( -33.58253175000000113, 53.37500000273119838, 0.000000000000000000 ) ) ;
#6713=CARTESIAN_POINT ( 'NONE',  ( -10.04305231718578462, 66.90000000546238823, 30.90933677959249337 ) ) ;
#6717=VERTEX_POINT ( 'NONE', #32626 ) ;
#6718=CARTESIAN_POINT ( 'NONE',  ( -20.75514604977248823, 39.07500000273119412, -28.56700777964554305 ) ) ;
#6720=CARTESIAN_POINT ( 'NONE',  ( -32.50000000000000000, 28.40000000546235981, -10.55989012756945478 ) ) ;
#6739=CARTESIAN_POINT ( 'NONE',  ( 29.16592172374795311, 52.00000000000002842, 16.79171150063938356 ) ) ;
#6741=CARTESIAN_POINT ( 'NONE',  ( 26.29305231718578995, 3.199999999999994404, -19.10302069950538240 ) ) ;
#6746=CARTESIAN_POINT ( 'NONE',  ( -10.37757302488623701, 65.52500000273118985, 31.93888565452638417 ) ) ;
#6747=CARTESIAN_POINT ( 'NONE',  ( 33.58253175000000823, 26.27500000273119340, 10.91162601494192863 ) ) ;
#6748=CARTESIAN_POINT ( 'NONE',  ( -33.58253175000000113, 7.475000002731190030, 10.91162601494193929 ) ) ;
#6753=CARTESIAN_POINT ( 'NONE',  ( 32.50000000000000000, 47.10000000000000142, -10.55989012756945833 ) ) ;
#6754=CARTESIAN_POINT ( 'NONE',  ( 10.04305231718579705, 57.10000000546237686, 30.90933677959248982 ) ) ;
#6759=CARTESIAN_POINT ( 'NONE',  ( -20.75514604977248823, 59.07500000273119412, -28.56700777964554305 ) ) ;
#6765=CARTESIAN_POINT ( 'NONE',  ( 33.58253175000000823, 32.02500000273118275, 10.91162601494192863 ) ) ;
#6787=CARTESIAN_POINT ( 'NONE',  ( 27.16883889988623935, 44.57500000273119412, -19.73931689729374384 ) ) ;
#6792=CARTESIAN_POINT ( 'NONE',  ( 26.29305231718579350, 68.80000000000001137, 19.10302069950537529 ) ) ;
#6802=CARTESIAN_POINT ( 'NONE',  ( 33.58253175000000113, 52.22500000273117848, -10.91162601494193751 ) ) ;
#6803=CARTESIAN_POINT ( 'NONE',  ( -27.16883889988623935, 23.57500000273120122, 19.73931689729374739 ) ) ;
#6817=CARTESIAN_POINT ( 'NONE',  ( 10.37757302488624767, 55.72500000273118559, 31.93888565452638417 ) ) ;
#6832=CARTESIAN_POINT ( 'NONE',  ( -20.75514604977248823, 20.82500000273119412, -28.56700777964554305 ) ) ;
#6834=CARTESIAN_POINT ( 'NONE',  ( 5.779280353836490358E-15, 55.00000000546238965, 32.49999999999999289 ) ) ;
#6835=ADVANCED_FACE ( 'NONE', ( #22140 ), #3605, .F. ) ;
#6839=CARTESIAN_POINT ( 'NONE',  ( 32.50000000000000711, 39.40000000546236691, 10.55989012756945122 ) ) ;
#6846=CARTESIAN_POINT ( 'NONE',  ( -20.75514604977248823, 70.82500000273117280, -28.56700777964554305 ) ) ;
#6848=MECHANICAL_DESIGN_GEOMETRIC_PRESENTATION_REPRESENTATION('',(#11770),#29846);
#6853=CARTESIAN_POINT ( 'NONE',  ( -33.58253175000000113, 11.02500000273117919, -10.91162601494193218 ) ) ;
#6862=CARTESIAN_POINT ( 'NONE',  ( 20.08610463437157279, 37.30000000000001847, -27.64615127144129758 ) ) ;
#6874=CARTESIAN_POINT ( 'NONE',  ( 27.16883889988624290, 41.92500000273118133, 19.73931689729373673 ) ) ;
#6875=CARTESIAN_POINT ( 'NONE',  ( 33.58253175000000113, 2.375000002731192161, -4.112674001490185761E-15 ) ) ;
#6876=CARTESIAN_POINT ( 'NONE',  ( -20.75514604977248823, 53.07500000273118701, -28.56700777964554305 ) ) ;
#6879=CARTESIAN_POINT ( 'NONE',  ( -32.50000000000000000, 62.60000000546238397, 10.55989012756946366 ) ) ;
#6887=CARTESIAN_POINT ( 'NONE',  ( -20.75514604977248112, 41.67500000273117422, 28.56700777964554661 ) ) ;
#6890=CARTESIAN_POINT ( 'NONE',  ( -20.08610463437157989, 32.20000000546238539, -27.64615127144129758 ) ) ;
#6891=ORIENTED_EDGE ( 'NONE', *, *, #16640, .T. ) ;
#6900=CARTESIAN_POINT ( 'NONE',  ( 20.75514604977249178, 65.82500000273115859, 28.56700777964553950 ) ) ;
#6911=CARTESIAN_POINT ( 'NONE',  ( 32.50000000000000000, 6.999999999999992006, -3.980102097228898626E-15 ) ) ;
#6915=CARTESIAN_POINT ( 'NONE',  ( -33.58253175000000113, 61.22500000273118559, 10.91162601494193929 ) ) ;
#6916=CARTESIAN_POINT ( 'NONE',  ( -27.16883889988623935, 23.57500000273120122, 19.73931689729374739 ) ) ;
#6917=CARTESIAN_POINT ( 'NONE',  ( 10.37757302488624056, 12.77500000273117031, -31.93888565452638417 ) ) ;
#6921=CARTESIAN_POINT ( 'NONE',  ( -20.75514604977248823, 2.825000002731177240, -28.56700777964554305 ) ) ;
#6923=CARTESIAN_POINT ( 'NONE',  ( -32.50000000000000000, 41.89999999999999147, -10.55989012756945478 ) ) ;
#6926=CARTESIAN_POINT ( 'NONE',  ( -12.90513655866680587, 66.99999999999998579, -31.00393344628902881 ) ) ;
#6929=CARTESIAN_POINT ( 'NONE',  ( -27.16883889988624290, 59.17500000273119554, -19.73931689729374028 ) ) ;
#6933=EDGE_CURVE ( 'NONE', #25517, #1690, #6518, .T. ) ;
#6935=CARTESIAN_POINT ( 'NONE',  ( 10.37757302488624767, 31.72500000273119269, 31.93888565452638417 ) ) ;
#6955=CARTESIAN_POINT ( 'NONE',  ( 10.37757302488624767, 39.97500000273117138, 31.93888565452638417 ) ) ;
#6961=CARTESIAN_POINT ( 'NONE',  ( -32.50000000000000000, 65.99999999999998579, 0.000000000000000000 ) ) ;
#6972=CARTESIAN_POINT ( 'NONE',  ( -2.162160676586881955E-15, 46.62500000273119127, -35.31076352940723240 ) ) ;
#6973=CARTESIAN_POINT ( 'NONE',  ( 20.75514604977249178, 24.07500000273120122, 28.56700777964553950 ) ) ;
#6997=CARTESIAN_POINT ( 'NONE',  ( 27.16883889988624290, 64.17500000273116711, 19.73931689729373673 ) ) ;
#7003=CARTESIAN_POINT ( 'NONE',  ( 20.08610463437158344, 63.20000000546237118, 27.64615127144129403 ) ) ;
#7005=CARTESIAN_POINT ( 'NONE',  ( -2.162160676586881955E-15, 22.62500000273119127, -35.31076352940723240 ) ) ;
#7009=CARTESIAN_POINT ( 'NONE',  ( -10.04305231718579172, 44.10000000546236976, -30.90933677959248982 ) ) ;
#7014=CARTESIAN_POINT ( 'NONE',  ( 33.58253175000000113, 68.12500000273118417, -4.112674001490185761E-15 ) ) ;
#7021=CARTESIAN_POINT ( 'NONE',  ( -33.58253175000000113, 13.22500000273119802, 10.91162601494193929 ) ) ;
#7030=CARTESIAN_POINT ( 'NONE',  ( 32.50000000000000000, 36.99999999999999289, -3.980102097228898626E-15 ) ) ;
#7034=CARTESIAN_POINT ( 'NONE',  ( -13.17636326499370014, 67.00000000000004263, 29.96527208688299027 ) ) ;
#7044=CARTESIAN_POINT ( 'NONE',  ( 27.16883889988623935, 40.32500000273118701, -19.73931689729374384 ) ) ;
#7045=CARTESIAN_POINT ( 'NONE',  ( 33.58253175000000823, 2.275000002731194293, 10.91162601494192863 ) ) ;
#7046=CARTESIAN_POINT ( 'NONE',  ( 33.58253175000000113, 56.37500000273119838, -4.112674001490185761E-15 ) ) ;
#7050=CARTESIAN_POINT ( 'NONE',  ( -26.29305231718578995, 62.70000000546237118, 19.10302069950538595 ) ) ;
#7056=CARTESIAN_POINT ( 'NONE',  ( 20.75514604977249178, 40.07500000273118701, 28.56700777964553950 ) ) ;
#7061=CARTESIAN_POINT ( 'NONE',  ( -32.50000000000000000, 26.40000000546236336, -10.55989012756945478 ) ) ;
#7078=CARTESIAN_POINT ( 'NONE',  ( -32.50000000000000000, 55.90000000000000568, -10.55989012756945300 ) ) ;
#7079=CARTESIAN_POINT ( 'NONE',  ( 30.20345010595902480, 52.00000000000000711, 14.84467937978581453 ) ) ;
#7080=CARTESIAN_POINT ( 'NONE',  ( -32.50000000000000000, 6.099999999999996092, 10.55989012756946366 ) ) ;
#7085=CARTESIAN_POINT ( 'NONE',  ( -33.58253175000000113, 59.02500000273120406, -10.91162601494193218 ) ) ;
#7086=CARTESIAN_POINT ( 'NONE',  ( 33.58253175000000823, 24.27500000273120051, 10.91162601494192863 ) ) ;
#7087=CARTESIAN_POINT ( 'NONE',  ( -10.37757302488624411, 8.975000002731201576, -31.93888565452638417 ) ) ;
#7091=CARTESIAN_POINT ( 'NONE',  ( 10.04305231718579705, 77.10000000546239107, 30.90933677959248982 ) ) ;
#7093=CARTESIAN_POINT ( 'NONE',  ( -32.50000000000000000, 44.00000000000000000, 0.000000000000000000 ) ) ;
#7096=PRODUCT ( 'lock nut', 'lock nut', '', ( #31185 ) ) ;
#7099=CARTESIAN_POINT ( 'NONE',  ( -27.16883889988623935, 61.57500000273117990, 19.73931689729374739 ) ) ;
#7104=CARTESIAN_POINT ( 'NONE',  ( -33.58253175000000113, 31.12500000273120548, 0.000000000000000000 ) ) ;
#7117=CARTESIAN_POINT ( 'NONE',  ( 32.50000000000000711, 54.90000000000001279, 10.55989012756945122 ) ) ;
#7122=ADVANCED_FACE ( 'NONE', ( #22306 ), #9245, .T. ) ;
#7125=CARTESIAN_POINT ( 'NONE',  ( 20.75514604977248467, 42.67500000273119554, -28.56700777964554305 ) ) ;
#7127=CARTESIAN_POINT ( 'NONE',  ( -1.137977401836464321E-14, 52.00000000000000711, 46.18802153517007270 ) ) ;
#7131=CARTESIAN_POINT ( 'NONE',  ( -10.04305231718579172, 59.60000000000000142, -30.90933677959248982 ) ) ;
#7141=CARTESIAN_POINT ( 'NONE',  ( 6.486482029760649416E-15, 47.62500000273118417, 35.31076352940723240 ) ) ;
#7142=CARTESIAN_POINT ( 'NONE',  ( 27.16883889988623935, 22.57500000273120122, -19.73931689729374384 ) ) ;
#7166=CARTESIAN_POINT ( 'NONE',  ( -20.75514604977248823, 59.07500000273119412, -28.56700777964554305 ) ) ;
#7174=CARTESIAN_POINT ( 'NONE',  ( -20.75514604977248823, 22.82500000273118701, -28.56700777964554305 ) ) ;
#7176=CARTESIAN_POINT ( 'NONE',  ( 32.50000000000000000, 53.09999999999998010, -10.55989012756945833 ) ) ;
#7177=CARTESIAN_POINT ( 'NONE',  ( 40.00000000000000000, 52.00000000000000711, -23.09401076758505766 ) ) ;
#7179=CARTESIAN_POINT ( 'NONE',  ( -32.50000000000000000, 40.60000000546239107, 10.55989012756946366 ) ) ;
#7185=CARTESIAN_POINT ( 'NONE',  ( 10.37757302488624056, 66.52500000273118985, -31.93888565452638417 ) ) ;
#7191=CARTESIAN_POINT ( 'NONE',  ( -20.75514604977248823, 12.82500000273119589, -28.56700777964554305 ) ) ;
#7201=CARTESIAN_POINT ( 'NONE',  ( 10.04305231718579705, 26.59999999999999787, 30.90933677959248982 ) ) ;
#7215=CARTESIAN_POINT ( 'NONE',  ( -33.58253175000000113, 39.12500000273118417, 0.000000000000000000 ) ) ;
#7216=CARTESIAN_POINT ( 'NONE',  ( -20.75514604977248112, 3.675000002731193316, 28.56700777964554661 ) ) ;
#7217=CARTESIAN_POINT ( 'NONE',  ( -2.162160676586882350E-15, 58.87500000273117706, -35.31076352940722529 ) ) ;
#7220=CARTESIAN_POINT ( 'NONE',  ( 26.29305231718579350, 59.30000000546238681, 19.10302069950537529 ) ) ;
#7226=CARTESIAN_POINT ( 'NONE',  ( 6.486482029760649416E-15, 33.87500000273118417, 35.31076352940723240 ) ) ;
#7230=CARTESIAN_POINT ( 'NONE',  ( 26.29305231718578995, 25.70000000546239605, -19.10302069950538240 ) ) ;
#7242=VECTOR ( 'NONE', #6383, 1000.000000000000227 ) ;
#7248=CARTESIAN_POINT ( 'NONE',  ( 32.50000000000000711, 6.899999999999999467, 10.55989012756945122 ) ) ;
#7253=CARTESIAN_POINT ( 'NONE',  ( -20.75514604977248823, 58.82500000273117990, -28.56700777964554305 ) ) ;
#7254=CARTESIAN_POINT ( 'NONE',  ( 10.37757302488624056, 22.77500000273117919, -31.93888565452638417 ) ) ;
#7255=CARTESIAN_POINT ( 'NONE',  ( -20.75514604977248112, 9.675000002731193760, 28.56700777964554661 ) ) ;
#7260=CARTESIAN_POINT ( 'NONE',  ( 32.50000000000000000, 77.60000000546239107, -10.55989012756945833 ) ) ;
#7263=CARTESIAN_POINT ( 'NONE',  ( -2.092463501923844636E-15, 39.50000000000000000, -34.17252228774368916 ) ) ;
#7270=CARTESIAN_POINT ( 'NONE',  ( 33.58253175000000823, 52.27500000273118985, 10.91162601494192863 ) ) ;
#7276=CARTESIAN_POINT ( 'NONE',  ( -20.75514604977248112, 31.42500000273120619, 28.56700777964554661 ) ) ;
#7295=CARTESIAN_POINT ( 'NONE',  ( -10.37757302488624411, 78.72500000273117848, -31.93888565452638417 ) ) ;
#7296=CARTESIAN_POINT ( 'NONE',  ( -10.37757302488624411, 44.97500000273117848, -31.93888565452638417 ) ) ;
#7299=AXIS2_PLACEMENT_3D ( 'NONE', #5090, #22771, #2166 ) ;
#7302=CARTESIAN_POINT ( 'NONE',  ( -2.092463501923844636E-15, 63.50000000000000000, -34.17252228774368916 ) ) ;
#7307=CARTESIAN_POINT ( 'NONE',  ( 6.486482029760649416E-15, 77.87500000273118417, 35.31076352940723240 ) ) ;
#7312=CARTESIAN_POINT ( 'NONE',  ( 20.75514604977248467, 52.42500000273118133, -28.56700777964554305 ) ) ;
#7318=CARTESIAN_POINT ( 'NONE',  ( -10.04305231718579172, 8.100000005462391073, -30.90933677959248982 ) ) ;
#7338=CARTESIAN_POINT ( 'NONE',  ( 27.16883889988624290, 62.17500000273119554, 19.73931689729373673 ) ) ;
#7344=CARTESIAN_POINT ( 'NONE',  ( 26.29305231718578995, 79.20000000000000284, -19.10302069950538240 ) ) ;
#7345=CARTESIAN_POINT ( 'NONE',  ( 6.486482029760649416E-15, 19.62500000273116996, 35.31076352940723240 ) ) ;
#7351=CARTESIAN_POINT ( 'NONE',  ( 32.50000000000000711, 41.40000000546238823, 10.55989012756945122 ) ) ;
#7356=CARTESIAN_POINT ( 'NONE',  ( 33.58253175000000823, 72.02500000273118985, 10.91162601494192863 ) ) ;
#7364=CARTESIAN_POINT ( 'NONE',  ( -10.37757302488623701, 9.525000002731195181, 31.93888565452638417 ) ) ;
#7377=CARTESIAN_POINT ( 'NONE',  ( -20.08610463437157989, 27.69999999999999929, -27.64615127144129758 ) ) ;
#7389=CARTESIAN_POINT ( 'NONE',  ( -33.58253175000000113, 43.12500000273118417, 0.000000000000000000 ) ) ;
#7391=CARTESIAN_POINT ( 'NONE',  ( 33.58253175000000113, 56.47500000273116427, -10.91162601494193574 ) ) ;
#7395=CARTESIAN_POINT ( 'NONE',  ( -10.04305231718579172, 64.10000000546239107, -30.90933677959248982 ) ) ;
#7398=CARTESIAN_POINT ( 'NONE',  ( 26.29305231718579350, 57.30000000546238681, 19.10302069950537529 ) ) ;
#7403=CARTESIAN_POINT ( 'NONE',  ( -20.75514604977248112, 33.67500000273119554, 28.56700777964554661 ) ) ;
#7407=CARTESIAN_POINT ( 'NONE',  ( 26.29305231718578995, 23.70000000546239249, -19.10302069950538240 ) ) ;
#7412=FACE_OUTER_BOUND ( 'NONE', #13782, .T. ) ;
#7417=CARTESIAN_POINT ( 'NONE',  ( 33.58253175000000113, 60.12500000273117706, -4.112674001490185761E-15 ) ) ;
#7426=CARTESIAN_POINT ( 'NONE',  ( -32.50000000000000000, 52.00000000000000711, 0.000000000000000000 ) ) ;
#7427=CARTESIAN_POINT ( 'NONE',  ( 27.16883889988623935, 72.57500000273118701, -19.73931689729374384 ) ) ;
#7434=CARTESIAN_POINT ( 'NONE',  ( 6.486482029760649416E-15, 57.62500000273119127, 35.31076352940723240 ) ) ;
#7435=CARTESIAN_POINT ( 'NONE',  ( 20.75514604977249178, 16.07500000273119412, 28.56700777964553950 ) ) ;
#7436=CARTESIAN_POINT ( 'NONE',  ( -33.58253175000000113, 9.475000002731185589, 10.91162601494193929 ) ) ;
#7442=CARTESIAN_POINT ( 'NONE',  ( -27.16883889988624290, 4.925000002731189319, -19.73931689729374028 ) ) ;
#7444=CARTESIAN_POINT ( 'NONE',  ( 32.50000000000000711, 42.90000000000001279, 10.55989012756945122 ) ) ;
#7449=CARTESIAN_POINT ( 'NONE',  ( 33.58253175000000113, 54.37500000273119838, -4.112674001490185761E-15 ) ) ;
#7450=CARTESIAN_POINT ( 'NONE',  ( 5.147494310547481966, 59.94874572391553613, -32.49999999999998579 ) ) ;
#7455=CARTESIAN_POINT ( 'NONE',  ( -20.75514604977248112, 23.42500000273119909, 28.56700777964554661 ) ) ;
#7472=CARTESIAN_POINT ( 'NONE',  ( 10.04305231718579705, 16.59999999999999076, 30.90933677959248982 ) ) ;
#7478=FACE_OUTER_BOUND ( 'NONE', #23074, .T. ) ;
#7479=CARTESIAN_POINT ( 'NONE',  ( -33.58253175000000113, 41.27500000273117564, -10.91162601494193218 ) ) ;
#7485=CARTESIAN_POINT ( 'NONE',  ( -32.50000000000000000, 62.09999999999999432, 10.55989012756946366 ) ) ;
#7489=CARTESIAN_POINT ( 'NONE',  ( 33.58253175000000113, 72.47500000273119269, -10.91162601494193751 ) ) ;
#7494=CARTESIAN_POINT ( 'NONE',  ( 20.75514604977248467, 42.42500000273117422, -28.56700777964554305 ) ) ;
#7498=CARTESIAN_POINT ( 'NONE',  ( -32.50000000000000000, 4.400000005462378461, -10.55989012756945478 ) ) ;
#7516=CARTESIAN_POINT ( 'NONE',  ( -20.75514604977248823, 65.07500000273118701, -28.56700777964554305 ) ) ;
#7523=CARTESIAN_POINT ( 'NONE',  ( 20.08610463437158344, 76.70000000000000284, 27.64615127144129403 ) ) ;
#7524=CARTESIAN_POINT ( 'NONE',  ( -33.58253175000000113, 13.22500000273119802, 10.91162601494193929 ) ) ;
#7529=CARTESIAN_POINT ( 'NONE',  ( 32.50000000000000000, 33.60000000546237686, -10.55989012756945833 ) ) ;
#7530=CARTESIAN_POINT ( 'NONE',  ( -10.04305231718578462, 66.40000000000000568, 30.90933677959249337 ) ) ;
#7534=CARTESIAN_POINT ( 'NONE',  ( 27.16883889988623935, 68.32500000273118701, -19.73931689729374384 ) ) ;
#7539=CARTESIAN_POINT ( 'NONE',  ( 20.75514604977248467, 12.42500000273117777, -28.56700777964554305 ) ) ;
#7550=CARTESIAN_POINT ( 'NONE',  ( -10.04305231718578462, 30.39999999999999503, 30.90933677959249337 ) ) ;
#7561=CARTESIAN_POINT ( 'NONE',  ( 27.48632242023158767, 66.99999999999998579, -17.98641839608171011 ) ) ;
#7562=CARTESIAN_POINT ( 'NONE',  ( -33.58253175000000113, 37.22500000273119980, 10.91162601494193929 ) ) ;
#7563=DIRECTION ( 'NONE',  ( 0.4999999999999998890, -0.000000000000000000, 0.8660254037844387076 ) ) ;
#7568=CARTESIAN_POINT ( 'NONE',  ( 20.08610463437157279, 63.80000000546237970, -27.64615127144129758 ) ) ;
#7570=FILL_AREA_STYLE ('',( #2934 ) ) ;
#7576=CARTESIAN_POINT ( 'NONE',  ( -2.162160676586881955E-15, 36.87500000273116996, -35.31076352940723240 ) ) ;
#7577=( BOUNDED_CURVE ( )  B_SPLINE_CURVE ( 2, ( #10755, #21233, #16418, #31676, #16085, #13835, #776, #11258, #21734, #32179, #8674, #26200, #25035, #25206, #1683, #33086, #5083, #29378, #19257, #6036, #21668, #11031, #16683, #16515, #11358, #5877, #21500, #32614, #8441, #29875, #24730, #13770, #16355, #9111, #3634, #24402, #6375, #6203, #29698, #32114, #16853, #30040, #21836, #11686, #26967, #18932, #3468, #29533, #13938, #878, #24895, #31948, #27140, #32281, #8774, #26810, #3305, #19592, #24240, #27310, #1205, #19425, #14108, #19095, #17018, #24565, #3801, #1038, #11518, #21998, #32446, #22170, #711, #8947, #11197, #8612, #14273, #6545, #27478, #14440, #3967, #17190, #33471, #7217, #27648, #30722, #14951, #20104, #33299, #33120, #17528, #15295, #28328, #30206, #4816, #1548, #27820, #14611, #25067, #12371, #1895, #9623, #9971, #27989, #9799, #4303, #1381, #7391, #7046, #4476, #20447, #12197, #25417, #4646, #22839, #4136, #17876, #14778, #30897, #12024, #15126, #30550, #25243, #20275, #22493, #17700, #11855, #28160, #25589, #22334, #2069, #12545, #32944, #23016, #9273, #9445, #32779, #19757, #6708, #19929, #30375, #6876, #17356, #1718, #22668, #25755, #10822, #31409, #13399, #2928, #23869, #29000, #162 ),
 .UNSPECIFIED., .F., .T. ) 
 B_SPLINE_CURVE_WITH_KNOTS ( ( 3, 2, 2, 2, 2, 2, 2, 2, 2, 2, 2, 2, 2, 2, 2, 2, 2, 2, 2, 2, 2, 2, 2, 2, 2, 2, 2, 2, 2, 2, 2, 2, 2, 2, 2, 2, 2, 2, 2, 2, 2, 2, 2, 2, 2, 2, 2, 2, 2, 2, 2, 2, 2, 2, 2, 2, 2, 2, 2, 2, 2, 2, 2, 2, 2, 2, 2, 2, 2, 2, 2, 2, 2, 2, 2, 2, 3 ),
 ( 0.1586432617944051326, 0.1589743589743589647, 0.1615384615384615474, 0.1641025641025641024, 0.1666666666666666574, 0.1692307692307692402, 0.1717948717948717952, 0.1743589743589743501, 0.1769230769230769329, 0.1794871794871794879, 0.1820512820512820429, 0.1846153846153846256, 0.1871794871794871806, 0.1897435897435897356, 0.1923076923076923184, 0.1948717948717948734, 0.1974358974358974284, 0.2000000000000000111, 0.2025641025641025661, 0.2051282051282051211, 0.2076923076923077038, 0.2102564102564102588, 0.2128205128205128138, 0.2153846153846153966, 0.2179487179487179516, 0.2205128205128205066, 0.2230769230769230893, 0.2256410256410256443, 0.2282051282051281993, 0.2307692307692307820, 0.2333333333333333370, 0.2358974358974358920, 0.2384615384615384748, 0.2410256410256410298, 0.2435897435897435848, 0.2461538461538461675, 0.2487179487179487225, 0.2512820512820512775, 0.2538461538461538325, 0.2564102564102563875, 0.2589743589743589980, 0.2615384615384615530, 0.2641025641025641080, 0.2666666666666666630, 0.2692307692307692180, 0.2717948717948717730, 0.2743589743589743835, 0.2769230769230769384, 0.2794871794871794934, 0.2820512820512820484, 0.2846153846153846034, 0.2871794871794871584, 0.2897435897435897689, 0.2923076923076923239, 0.2948717948717948789, 0.2974358974358974339, 0.2999999999999999889, 0.3025641025641025439, 0.3051282051282051544, 0.3076923076923077094, 0.3102564102564102644, 0.3128205128205128194, 0.3153846153846153744, 0.3179487179487179294, 0.3205128205128205399, 0.3230769230769230949, 0.3256410256410257054, 0.3282051282051282048, 0.3307692307692307598, 0.3333333333333333148, 0.3358974358974358698, 0.3384615384615384803, 0.3410256410256410353, 0.3435897435897435903, 0.3461538461538461453, 0.3487179487179487003, 0.3509509541020974233 ),
 .UNSPECIFIED. ) 
 CURVE ( )  GEOMETRIC_REPRESENTATION_ITEM ( )  RATIONAL_B_SPLINE_CURVE ( ( 0.9889922301674716199, 0.9936800307216014927, 1.000000000000000000, 0.9510565162951535312, 1.000000000000000000, 0.9510565162951535312, 1.000000000000000000, 0.9510565162951535312, 1.000000000000000000, 0.9510565162951535312, 1.000000000000000000, 0.9510565162951535312, 1.000000000000000000, 0.9510565162951535312, 1.000000000000000000, 0.9510565162951535312, 1.000000000000000000, 0.9510565162951535312, 1.000000000000000000, 0.9510565162951535312, 1.000000000000000000, 0.9510565162951535312, 1.000000000000000000, 0.9510565162951535312, 1.000000000000000000, 0.9510565162951535312, 1.000000000000000000, 0.9510565162951535312, 1.000000000000000000, 0.9510565162951535312, 1.000000000000000000, 0.9510565162951535312, 1.000000000000000000, 0.9510565162951535312, 1.000000000000000000, 0.9510565162951535312, 1.000000000000000000, 0.9510565162951535312, 1.000000000000000000, 0.9510565162951535312, 1.000000000000000000, 0.9510565162951535312, 1.000000000000000000, 0.9510565162951535312, 1.000000000000000000, 0.9510565162951535312, 1.000000000000000000, 0.9510565162951535312, 1.000000000000000000, 0.9510565162951535312, 1.000000000000000000, 0.9510565162951535312, 1.000000000000000000, 0.9510565162951535312, 1.000000000000000000, 0.9510565162951535312, 1.000000000000000000, 0.9510565162951535312, 1.000000000000000000, 0.9510565162951535312, 1.000000000000000000, 0.9510565162951535312, 1.000000000000000000, 0.9510565162951535312, 1.000000000000000000, 0.9510565162951535312, 1.000000000000000000, 0.9510565162951535312, 1.000000000000000000, 0.9510565162951535312, 1.000000000000000000, 0.9510565162951535312, 1.000000000000000000, 0.9510565162951535312, 1.000000000000000000, 0.9510565162951535312, 1.000000000000000000, 0.9510565162951535312, 1.000000000000000000, 0.9510565162951535312, 1.000000000000000000, 0.9510565162951535312, 1.000000000000000000, 0.9510565162951535312, 1.000000000000000000, 0.9510565162951535312, 1.000000000000000000, 0.9510565162951535312, 1.000000000000000000, 0.9510565162951535312, 1.000000000000000000, 0.9510565162951535312, 1.000000000000000000, 0.9510565162951535312, 1.000000000000000000, 0.9510565162951535312, 1.000000000000000000, 0.9510565162951535312, 1.000000000000000000, 0.9510565162951535312, 1.000000000000000000, 0.9510565162951535312, 1.000000000000000000, 0.9510565162951535312, 1.000000000000000000, 0.9510565162951535312, 1.000000000000000000, 0.9510565162951535312, 1.000000000000000000, 0.9510565162951535312, 1.000000000000000000, 0.9510565162951535312, 1.000000000000000000, 0.9510565162951535312, 1.000000000000000000, 0.9510565162951535312, 1.000000000000000000, 0.9510565162951535312, 1.000000000000000000, 0.9510565162951535312, 1.000000000000000000, 0.9510565162951535312, 1.000000000000000000, 0.9510565162951535312, 1.000000000000000000, 0.9510565162951535312, 1.000000000000000000, 0.9510565162951535312, 1.000000000000000000, 0.9510565162951535312, 1.000000000000000000, 0.9510565162951535312, 1.000000000000000000, 0.9510565162951535312, 1.000000000000000000, 0.9510565162951535312, 1.000000000000000000, 0.9510565162951535312, 1.000000000000000000, 0.9510565162951535312, 1.000000000000000000, 0.9510565162951535312, 1.000000000000000000, 0.9510565162951535312, 1.000000000000000000, 0.9510565162951535312, 1.000000000000000000, 0.9510565162951535312, 1.000000000000000000, 0.9510565162951535312, 1.000000000000000000, 0.9573764855735520385, 0.9889922301674716199 ) ) 
 REPRESENTATION_ITEM ( '' )  );
#7582=CARTESIAN_POINT ( 'NONE',  ( -2.092463501923844636E-15, 26.00000000546237899, -34.17252228774368916 ) ) ;
#7592=CARTESIAN_POINT ( 'NONE',  ( 20.75514604977249178, 63.82500000273119412, 28.56700777964553950 ) ) ;
#7600=CARTESIAN_POINT ( 'NONE',  ( -20.75514604977248112, 77.67500000273119554, 28.56700777964554661 ) ) ;
#7605=CARTESIAN_POINT ( 'NONE',  ( -27.16883889988624290, 60.92500000273119554, -19.73931689729374028 ) ) ;
#7606=CARTESIAN_POINT ( 'NONE',  ( -33.58253175000000113, 15.37500000273118950, 0.000000000000000000 ) ) ;
#7607=CARTESIAN_POINT ( 'NONE',  ( 20.75514604977249178, 2.075000002731186122, 28.56700777964553950 ) ) ;
#7611=CARTESIAN_POINT ( 'NONE',  ( -2.162160676586881955E-15, 4.625000002731192161, -35.31076352940723240 ) ) ;
#7612=CARTESIAN_POINT ( 'NONE',  ( 21.77128556259169656, 51.99999999999997868, -24.67464075869979112 ) ) ;
#7613=CARTESIAN_POINT ( 'NONE',  ( -26.29305231718578995, 40.20000000000000284, 19.10302069950538595 ) ) ;
#7618=CARTESIAN_POINT ( 'NONE',  ( -27.16883889988624290, 57.17500000273119554, -19.73931689729374028 ) ) ;
#7622=ORIENTED_EDGE ( 'NONE', *, *, #765, .T. ) ;
#7623=CARTESIAN_POINT ( 'NONE',  ( -27.16883889988623935, 25.32500000273117635, 19.73931689729374739 ) ) ;
#7637=CARTESIAN_POINT ( 'NONE',  ( 32.50000000000000711, 18.90000000000001634, 10.55989012756945122 ) ) ;
#7643=CARTESIAN_POINT ( 'NONE',  ( -2.162160676586881955E-15, 78.62500000273115575, -35.31076352940723240 ) ) ;
#7644=CARTESIAN_POINT ( 'NONE',  ( 10.37757302488624056, 34.77500000273118985, -31.93888565452638417 ) ) ;
#7646=PRODUCT_DEFINITION ( 'UNKNOWN', '', #19203, #13396 ) ;
#7650=CARTESIAN_POINT ( 'NONE',  ( 26.29305231718578995, 59.20000000000001705, -19.10302069950538240 ) ) ;
#7654=CARTESIAN_POINT ( 'NONE',  ( -20.75514604977248823, 75.07500000273118701, -28.56700777964554305 ) ) ;
#7658=VERTEX_POINT ( 'NONE', #17326 ) ;
#7659=CARTESIAN_POINT ( 'NONE',  ( 27.16883889988623935, 44.32500000273119412, -19.73931689729374384 ) ) ;
#7663=CARTESIAN_POINT ( 'NONE',  ( -32.50000000000000000, 2.400000005462383790, -10.55989012756945478 ) ) ;
#7683=CARTESIAN_POINT ( 'NONE',  ( -27.16883889988623935, 53.57500000273117280, 19.73931689729374739 ) ) ;
#7690=CARTESIAN_POINT ( 'NONE',  ( 10.04305231718578817, 77.40000000000000568, -30.90933677959249337 ) ) ;
#7691=CARTESIAN_POINT ( 'NONE',  ( 33.58253175000000113, 16.12500000273119127, -4.112674001490185761E-15 ) ) ;
#7696=CARTESIAN_POINT ( 'NONE',  ( -20.08610463437156923, 36.80000000546239391, 27.64615127144130113 ) ) ;
#7701=CARTESIAN_POINT ( 'NONE',  ( 10.37757302488624767, 63.72500000273119269, 31.93888565452638417 ) ) ;
#7708=CARTESIAN_POINT ( 'NONE',  ( 10.37757302488624767, 7.725000002731172266, 31.93888565452638417 ) ) ;
#7715=CARTESIAN_POINT ( 'NONE',  ( 40.00000000000000000, 66.99999999999998579, -23.09401076758505766 ) ) ;
#7718=CARTESIAN_POINT ( 'NONE',  ( 10.04305231718579705, 32.60000000000000142, 30.90933677959248982 ) ) ;
#7728=CARTESIAN_POINT ( 'NONE',  ( -12.90513655866680587, 66.99999999999998579, -31.00393344628902881 ) ) ;
#7730=CARTESIAN_POINT ( 'NONE',  ( 10.37757302488624056, 32.52500000273118985, -31.93888565452638417 ) ) ;
#7734=CARTESIAN_POINT ( 'NONE',  ( -26.29305231718578995, 56.70000000546236407, 19.10302069950538595 ) ) ;
#7741=CARTESIAN_POINT ( 'NONE',  ( 33.58253175000000113, 36.37500000273118417, -4.112674001490185761E-15 ) ) ;
#7745=CARTESIAN_POINT ( 'NONE',  ( 26.29305231718579350, 21.30000000546237970, 19.10302069950537529 ) ) ;
#7750=ADVANCED_FACE ( 'NONE', ( #5599 ), #16415, .F. ) ;
#7758=CARTESIAN_POINT ( 'NONE',  ( -10.37757302488623701, 63.52500000273118985, 31.93888565452638417 ) ) ;
#7768=CARTESIAN_POINT ( 'NONE',  ( -10.37757302488624411, 76.97500000273120691, -31.93888565452638417 ) ) ;
#7772=CARTESIAN_POINT ( 'NONE',  ( -33.58253175000000113, 53.02500000273118985, -10.91162601494193218 ) ) ;
#7773=CARTESIAN_POINT ( 'NONE',  ( -27.16883889988623935, 17.57500000273119767, 19.73931689729374739 ) ) ;
#7774=CARTESIAN_POINT ( 'NONE',  ( 33.58253175000000113, 2.475000002731187809, -10.91162601494193751 ) ) ;
#7778=CARTESIAN_POINT ( 'NONE',  ( 10.04305231718578817, 73.90000000546235981, -30.90933677959249337 ) ) ;
#7779=CARTESIAN_POINT ( 'NONE',  ( 31.95463953835039206, 52.00000000000002842, 10.27070314127458772 ) ) ;
#7785=CARTESIAN_POINT ( 'NONE',  ( 27.16883889988623935, 54.57500000273117280, -19.73931689729374384 ) ) ;
#7789=CARTESIAN_POINT ( 'NONE',  ( 33.58253175000000823, 22.02500000273117919, 10.91162601494192863 ) ) ;
#7793=FACE_BOUND ( 'NONE', #20692, .T. ) ;
#7805=CARTESIAN_POINT ( 'NONE',  ( -20.08610463437156923, 14.29999999999998472, 27.64615127144130113 ) ) ;
#7811=CARTESIAN_POINT ( 'NONE',  ( -20.75514604977248823, 74.82500000273115859, -28.56700777964554305 ) ) ;
#7812=CARTESIAN_POINT ( 'NONE',  ( -27.16883889988623935, 33.57500000273118701, 19.73931689729374739 ) ) ;
#7819=CARTESIAN_POINT ( 'NONE',  ( -32.50000000000000000, 57.89999999999999858, -10.55989012756945478 ) ) ;
#7820=FACE_OUTER_BOUND ( 'NONE', #12602, .T. ) ;
#7824=CARTESIAN_POINT ( 'NONE',  ( 20.75514604977249178, 76.07500000273118701, 28.56700777964553950 ) ) ;
#7829=CARTESIAN_POINT ( 'NONE',  ( 33.58253175000000823, 42.02500000273118985, 10.91162601494192863 ) ) ;
#7833=CARTESIAN_POINT ( 'NONE',  ( 20.08610463437157279, 1.800000005462373709, -27.64615127144129758 ) ) ;
#7841=FACE_OUTER_BOUND ( 'NONE', #11089, .T. ) ;
#7852=CARTESIAN_POINT ( 'NONE',  ( 6.486482029760649416E-15, 53.87500000273118417, 35.31076352940723240 ) ) ;
#7856=FACE_OUTER_BOUND ( 'NONE', #25257, .T. ) ;
#7858=CARTESIAN_POINT ( 'NONE',  ( -33.58253175000000113, 15.12500000273118950, 0.000000000000000000 ) ) ;
#7859=DIRECTION ( 'NONE',  ( 0.000000000000000000, 1.000000000000000000, 0.000000000000000000 ) ) ;
#7863=CARTESIAN_POINT ( 'NONE',  ( -20.08610463437157989, 34.20000000546238539, -27.64615127144129758 ) ) ;
#7868=CARTESIAN_POINT ( 'NONE',  ( -33.58253175000000113, 65.22500000273117848, 10.91162601494193929 ) ) ;
#7875=CARTESIAN_POINT ( 'NONE',  ( 27.16883889988624290, 3.925000002731188431, 19.73931689729373673 ) ) ;
#7885=CARTESIAN_POINT ( 'NONE',  ( -20.08610463437157989, 21.69999999999998153, -27.64615127144129758 ) ) ;
#7900=CARTESIAN_POINT ( 'NONE',  ( 33.58253175000000113, 36.22500000273119980, -10.91162601494193751 ) ) ;
#7906=CARTESIAN_POINT ( 'NONE',  ( 26.29305231718578995, 55.70000000546236407, -19.10302069950538240 ) ) ;
#7913=CARTESIAN_POINT ( 'NONE',  ( -10.37757302488623701, 31.77500000273118630, 31.93888565452638417 ) ) ;
#7915=EDGE_LOOP ( 'NONE', ( #1051, #15161, #19943, #28255 ) ) ;
#7917=CARTESIAN_POINT ( 'NONE',  ( -32.50000000000000000, 18.40000000546238823, -10.55989012756945478 ) ) ;
#7927=CARTESIAN_POINT ( 'NONE',  ( 27.16883889988624290, 61.92500000273119554, 19.73931689729373673 ) ) ;
#7937=CARTESIAN_POINT ( 'NONE',  ( -33.58253175000000113, 75.37500000273118417, 0.000000000000000000 ) ) ;
#7942=CARTESIAN_POINT ( 'NONE',  ( 33.58253175000000823, 56.02500000273117564, 10.91162601494192863 ) ) ;
#7943=CARTESIAN_POINT ( 'NONE',  ( 27.16883889988623935, 16.57500000273119767, -19.73931689729374384 ) ) ;
#7944=CARTESIAN_POINT ( 'NONE',  ( 20.75514604977249178, 4.075000002731181681, 28.56700777964553950 ) ) ;
#7948=CARTESIAN_POINT ( 'NONE',  ( -32.50000000000000000, 74.50000000546238255, 0.000000000000000000 ) ) ;
#7950=CARTESIAN_POINT ( 'NONE',  ( 31.08180318173147327, 52.00000000000001421, -11.59917702625707214 ) ) ;
#7956=CARTESIAN_POINT ( 'NONE',  ( -20.75514604977248112, 53.67500000273119554, 28.56700777964554661 ) ) ;
#7961=CARTESIAN_POINT ( 'NONE',  ( 20.75514604977249178, 21.82500000273119056, 28.56700777964553950 ) ) ;
#7963=VECTOR ( 'NONE', #22596, 1000.000000000000000 ) ;
#7964=ORIENTED_EDGE ( 'NONE', *, *, #10518, .T. ) ;
#7975=CARTESIAN_POINT ( 'NONE',  ( -2.092463501923844636E-15, 13.50000000000001066, -34.17252228774368916 ) ) ;
#7981=CARTESIAN_POINT ( 'NONE',  ( 33.58253175000000113, 70.12500000273118417, -4.112674001490185761E-15 ) ) ;
#7982=CARTESIAN_POINT ( 'NONE',  ( 10.37757302488624056, 38.77500000273119696, -31.93888565452638417 ) ) ;
#7990=CARTESIAN_POINT ( 'NONE',  ( -10.04305231718579172, 53.60000000000002274, -30.90933677959248982 ) ) ;
#7996=CARTESIAN_POINT ( 'NONE',  ( 33.58253175000000823, 76.27500000273118985, 10.91162601494192863 ) ) ;
#8002=CARTESIAN_POINT ( 'NONE',  ( -27.16883889988623935, 41.32500000273119412, 19.73931689729374739 ) ) ;
#8007=CARTESIAN_POINT ( 'NONE',  ( -2.092463501923844636E-15, 4.000000005462377217, -34.17252228774368916 ) ) ;
#8025=CARTESIAN_POINT ( 'NONE',  ( -2.162160676586881955E-15, 58.87500000273117706, -35.31076352940723240 ) ) ;
#8031=CARTESIAN_POINT ( 'NONE',  ( -32.50000000000000000, 74.10000000000002274, 10.55989012756946366 ) ) ;
#8032=CARTESIAN_POINT ( 'NONE',  ( 33.58253175000000823, 14.02500000273117209, 10.91162601494192863 ) ) ;
#8036=CARTESIAN_POINT ( 'NONE',  ( -26.29305231718579350, 34.30000000546239391, -19.10302069950537884 ) ) ;
#8041=CARTESIAN_POINT ( 'NONE',  ( -20.75514604977248823, 64.82500000273120122, -28.56700777964554305 ) ) ;
#8045=CARTESIAN_POINT ( 'NONE',  ( 6.486482029760649416E-15, 3.625000002731194826, 35.31076352940723240 ) ) ;
#8055=VECTOR ( 'NONE', #27113, 1000.000000000000000 ) ;
#8056=CARTESIAN_POINT ( 'NONE',  ( -20.08610463437156923, 24.29999999999999005, 27.64615127144130113 ) ) ;
#8060=CARTESIAN_POINT ( 'NONE',  ( -23.28634348215024730, 66.99999999999997158, 23.32808161240111389 ) ) ;
#8066=CARTESIAN_POINT ( 'NONE',  ( 8.342407680043388396, 66.99999999999997158, -32.16802901964491213 ) ) ;
#8068=CARTESIAN_POINT ( 'NONE',  ( 10.37757302488624767, 35.72500000273119980, 31.93888565452638417 ) ) ;
#8073=CARTESIAN_POINT ( 'NONE',  ( 26.29305231718578995, 51.70000000546236407, -19.10302069950538240 ) ) ;
#8082=CARTESIAN_POINT ( 'NONE',  ( 27.16883889988623935, 28.57500000273117990, -19.73931689729374384 ) ) ;
#8084=EDGE_LOOP ( 'NONE', ( #1415, #5974, #24260, #1815 ) ) ;
#8086=CARTESIAN_POINT ( 'NONE',  ( 6.277390505771533514E-15, 19.00000000546236834, 34.17252228774368916 ) ) ;
#8096=CARTESIAN_POINT ( 'NONE',  ( 27.16883889988624290, 59.92500000273119554, 19.73931689729373673 ) ) ;
#8106=CARTESIAN_POINT ( 'NONE',  ( -10.37757302488624411, 72.97500000273120691, -31.93888565452638417 ) ) ;
#8110=CARTESIAN_POINT ( 'NONE',  ( -10.37757302488623701, 55.52500000273118275, 31.93888565452638417 ) ) ;
#8111=CARTESIAN_POINT ( 'NONE',  ( 27.16883889988624290, 20.17500000273118843, 19.73931689729373673 ) ) ;
#8112=CARTESIAN_POINT ( 'NONE',  ( -20.75514604977248823, 78.82500000273120122, -28.56700777964554305 ) ) ;
#8116=CARTESIAN_POINT ( 'NONE',  ( -32.50000000000000000, 70.60000000546234844, 10.55989012756946366 ) ) ;
#8124=CARTESIAN_POINT ( 'NONE',  ( 27.16883889988623935, 50.57500000273117280, -19.73931689729374384 ) ) ;
#8129=CARTESIAN_POINT ( 'NONE',  ( 20.75514604977248467, 22.42500000273119909, -28.56700777964554305 ) ) ;
#8144=CARTESIAN_POINT ( 'NONE',  ( -5.147494310547430452, 59.55125428154684641, -32.49999999999999289 ) ) ;
#8145=CARTESIAN_POINT ( 'NONE',  ( -32.50000000000000000, 15.89999999999999147, -10.55989012756945478 ) ) ;
#8151=CARTESIAN_POINT ( 'NONE',  ( -10.37757302488623701, 73.52500000273120406, 31.93888565452638417 ) ) ;
#8152=CARTESIAN_POINT ( 'NONE',  ( 27.16883889988623935, 36.57500000273118701, -19.73931689729374384 ) ) ;
#8157=CARTESIAN_POINT ( 'NONE',  ( 26.29305231718578995, 55.20000000000000995, -19.10302069950538240 ) ) ;
#8161=CARTESIAN_POINT ( 'NONE',  ( -10.37757302488623701, 63.77500000273118985, 31.93888565452638417 ) ) ;
#8166=CARTESIAN_POINT ( 'NONE',  ( -10.37757302488623701, 43.52500000273119696, 31.93888565452638417 ) ) ;
#8170=CARTESIAN_POINT ( 'NONE',  ( 6.277390505771533514E-15, 5.000000005462374553, 34.17252228774368916 ) ) ;
#8190=CARTESIAN_POINT ( 'NONE',  ( -20.75514604977248112, 57.67500000273118133, 28.56700777964554661 ) ) ;
#8192=CARTESIAN_POINT ( 'NONE',  ( 0.000000000000000000, 52.00000000000000711, 32.50000000000000000 ) ) ;
#8196=CARTESIAN_POINT ( 'NONE',  ( 6.277390505771533514E-15, 72.50000000000001421, 34.17252228774368916 ) ) ;
#8197=CARTESIAN_POINT ( 'NONE',  ( -27.16883889988623935, 13.32500000273119412, 19.73931689729374739 ) ) ;
#8201=CARTESIAN_POINT ( 'NONE',  ( -10.04305231718579172, 34.10000000546238397, -30.90933677959248982 ) ) ;
#8206=CARTESIAN_POINT ( 'NONE',  ( 20.75514604977248467, 60.42500000273118133, -28.56700777964554305 ) ) ;
#8207=ORIENTED_EDGE ( 'NONE', *, *, #31700, .T. ) ;
#8210=CARTESIAN_POINT ( 'NONE',  ( 33.58253175000000113, 6.225000002731185589, -10.91162601494193751 ) ) ;
#8216=CARTESIAN_POINT ( 'NONE',  ( -5.147494310547423346, 52.94874572391553613, 32.50000000000000000 ) ) ;
#8218=CARTESIAN_POINT ( 'NONE',  ( -32.50000000000000000, 26.00000000000001066, 0.000000000000000000 ) ) ;
#8222=CARTESIAN_POINT ( 'NONE',  ( -29.99227890624900894, 66.99999999999998579, 14.07346378240356266 ) ) ;
#8231=CARTESIAN_POINT ( 'NONE',  ( 33.58253175000000823, 34.02500000273118275, 10.91162601494192863 ) ) ;
#8236=CARTESIAN_POINT ( 'NONE',  ( -10.04305231718578462, 52.90000000546239534, 30.90933677959249337 ) ) ;
#8242=CARTESIAN_POINT ( 'NONE',  ( -27.16883889988624290, 31.17500000273119909, -19.73931689729374028 ) ) ;
#8246=CARTESIAN_POINT ( 'NONE',  ( -2.092463501923844636E-15, 14.00000000546237899, -34.17252228774368916 ) ) ;
#8257=CARTESIAN_POINT ( 'NONE',  ( 33.58253175000000113, 52.22500000273118559, -10.91162601494193574 ) ) ;
#8266=CARTESIAN_POINT ( 'NONE',  ( -10.37757302488623701, 65.77500000273118985, 31.93888565452638417 ) ) ;
#8270=CARTESIAN_POINT ( 'NONE',  ( -20.75514604977248823, 52.82500000273116569, -28.56700777964554305 ) ) ;
#8271=CARTESIAN_POINT ( 'NONE',  ( -33.58253175000000113, 9.475000002731185589, 10.91162601494193929 ) ) ;
#8272=CARTESIAN_POINT ( 'NONE',  ( 10.37757302488624767, 3.975000002731182924, 31.93888565452638417 ) ) ;
#8276=CARTESIAN_POINT ( 'NONE',  ( 26.29305231718578995, 73.70000000546238539, -19.10302069950538240 ) ) ;
#8277=CARTESIAN_POINT ( 'NONE',  ( 33.02351622650643037, 51.99999999999999289, -4.441931073548142983 ) ) ;
#8283=CARTESIAN_POINT ( 'NONE',  ( -27.16883889988624290, 49.17500000273118843, -19.73931689729374028 ) ) ;
#8290=CARTESIAN_POINT ( 'NONE',  ( -27.16883889988623935, 17.32500000273119767, 19.73931689729374739 ) ) ;
#8300=CARTESIAN_POINT ( 'NONE',  ( -10.04305231718578462, 64.40000000000000568, 30.90933677959249337 ) ) ;
#8305=CARTESIAN_POINT ( 'NONE',  ( 20.08610463437158344, 10.69999999999999574, 27.64615127144129403 ) ) ;
#8311=CARTESIAN_POINT ( 'NONE',  ( -20.75514604977248823, 72.82500000273118701, -28.56700777964554305 ) ) ;
#8313=CARTESIAN_POINT ( 'NONE',  ( 33.58253175000000113, 38.47500000273118559, -10.91162601494193751 ) ) ;
#8320=CARTESIAN_POINT ( 'NONE',  ( 32.50000000000000000, 51.00000000000000711, -3.980102097228898626E-15 ) ) ;
#8321=DIRECTION ( 'NONE',  ( 0.000000000000000000, 1.000000000000000000, 0.000000000000000000 ) ) ;
#8326=CARTESIAN_POINT ( 'NONE',  ( 20.75514604977249178, 64.07500000273120122, 28.56700777964553950 ) ) ;
#8330=ORIENTED_EDGE ( 'NONE', *, *, #21754, .F. ) ;
#8331=CARTESIAN_POINT ( 'NONE',  ( -10.37757302488623701, 37.52500000273118985, 31.93888565452638417 ) ) ;
#8336=CARTESIAN_POINT ( 'NONE',  ( -1.778240108872766143E-15, 59.50000000000000711, -32.49999999999999289 ) ) ;
#8353=CARTESIAN_POINT ( 'NONE',  ( 33.58253175000000113, 54.47500000273117138, -10.91162601494193751 ) ) ;
#8360=CARTESIAN_POINT ( 'NONE',  ( 32.50000000000000711, 72.90000000000000568, 10.55989012756945122 ) ) ;
#8361=CARTESIAN_POINT ( 'NONE',  ( -33.58253175000000113, 7.225000002731182924, 10.91162601494193929 ) ) ;
#8366=( BOUNDED_CURVE ( )  B_SPLINE_CURVE ( 2, ( #22177, #19600, #32950, #27485, #3975, #14447, #4309, #9280, #19764, #14785, #17363, #22501, #27827 ),
 .UNSPECIFIED., .F., .T. ) 
 B_SPLINE_CURVE_WITH_KNOTS ( ( 3, 2, 2, 2, 2, 2, 3 ),
 ( 0.3269230769230769273, 0.3282051282051282048, 0.3307692307692307598, 0.3333333333333333148, 0.3358974358974358698, 0.3384615384615384803, 0.3397435897435897578 ),
 .UNSPECIFIED. ) 
 CURVE ( )  GEOMETRIC_REPRESENTATION_ITEM ( )  RATIONAL_B_SPLINE_CURVE ( ( 0.9755282581475768211, 0.9755282581475768211, 1.000000000000000000, 0.9510565162951535312, 1.000000000000000000, 0.9510565162951535312, 1.000000000000000000, 0.9510565162951535312, 1.000000000000000000, 0.9510565162951535312, 1.000000000000000000, 0.9755282581475768211, 0.9755282581475768211 ) ) 
 REPRESENTATION_ITEM ( '' )  );
#8371=CARTESIAN_POINT ( 'NONE',  ( 27.16883889988623935, 64.32500000273121543, -19.73931689729374384 ) ) ;
#8376=CARTESIAN_POINT ( 'NONE',  ( -27.16883889988623935, 3.325000002731184789, 19.73931689729374739 ) ) ;
#8386=CARTESIAN_POINT ( 'NONE',  ( 26.29305231718578995, 23.19999999999998508, -19.10302069950538240 ) ) ;
#8390=CARTESIAN_POINT ( 'NONE',  ( -31.08180318173140577, 66.99999999999998579, 11.59917702625715030 ) ) ;
#8397=CARTESIAN_POINT ( 'NONE',  ( -29.12397828776023800, 52.00000000000000000, 15.02363756889442570 ) ) ;
#8398=CARTESIAN_POINT ( 'NONE',  ( -10.37757302488623701, 27.52500000273118275, 31.93888565452638417 ) ) ;
#8399=CARTESIAN_POINT ( 'NONE',  ( 26.29305231718579350, 64.80000000000001137, 19.10302069950537529 ) ) ;
#8404=CARTESIAN_POINT ( 'NONE',  ( -32.50000000000000000, 52.50000000546238255, 0.000000000000000000 ) ) ;
#8412=ORIENTED_EDGE ( 'NONE', *, *, #19074, .T. ) ;
#8414=CARTESIAN_POINT ( 'NONE',  ( 32.50000000000000711, 17.40000000546238823, 10.55989012756945122 ) ) ;
#8425=CARTESIAN_POINT ( 'NONE',  ( 20.75514604977248467, 54.42500000273117422, -28.56700777964554305 ) ) ;
#8434=CARTESIAN_POINT ( 'NONE',  ( -33.58253175000000113, 65.37500000273121259, 0.000000000000000000 ) ) ;
#8439=CARTESIAN_POINT ( 'NONE',  ( 20.75514604977249178, 55.82500000273119412, 28.56700777964553950 ) ) ;
#8440=CARTESIAN_POINT ( 'NONE',  ( -33.58253175000000113, 11.37500000273118594, 0.000000000000000000 ) ) ;
#8441=CARTESIAN_POINT ( 'NONE',  ( 33.58253175000000113, 64.37500000273121259, -4.112674001490185761E-15 ) ) ;
#8445=CARTESIAN_POINT ( 'NONE',  ( 20.08610463437157279, 75.80000000546237970, -27.64615127144129758 ) ) ;
#8455=CARTESIAN_POINT ( 'NONE',  ( 20.75514604977249178, 50.07500000273120122, 28.56700777964553950 ) ) ;
#8460=CARTESIAN_POINT ( 'NONE',  ( 33.58253175000000113, 20.12500000273119483, -4.112674001490185761E-15 ) ) ;
#8471=EDGE_CURVE ( 'NONE', #24301, #9005, #3575, .T. ) ;
#8472=( BOUNDED_CURVE ( )  B_SPLINE_CURVE ( 2, ( #3003, #18293, #21202, #18795, #18460, #5405, #13298, #26510, #20864, #29239, #13126, #8144, #31310 ),
 .UNSPECIFIED., .F., .T. ) 
 B_SPLINE_CURVE_WITH_KNOTS ( ( 3, 2, 2, 2, 2, 2, 3 ),
 ( 0.2500000000000000000, 0.2512820512820512775, 0.2538461538461538325, 0.2564102564102563875, 0.2589743589743589980, 0.2615384615384615530, 0.2628205128205128305 ),
 .UNSPECIFIED. ) 
 CURVE ( )  GEOMETRIC_REPRESENTATION_ITEM ( )  RATIONAL_B_SPLINE_CURVE ( ( 0.9755282581475768211, 0.9755282581475768211, 1.000000000000000000, 0.9510565162951535312, 1.000000000000000000, 0.9510565162951535312, 1.000000000000000000, 0.9510565162951535312, 1.000000000000000000, 0.9510565162951535312, 1.000000000000000000, 0.9755282581475768211, 0.9755282581475768211 ) ) 
 REPRESENTATION_ITEM ( '' )  );
#8477=CARTESIAN_POINT ( 'NONE',  ( 32.50000000000000000, 10.99999999999999645, -3.980102097228898626E-15 ) ) ;
#8483=CARTESIAN_POINT ( 'NONE',  ( -10.37757302488623701, 75.52500000273120406, 31.93888565452638417 ) ) ;
#8484=CARTESIAN_POINT ( 'NONE',  ( -10.37757302488624411, 28.97500000273119269, -31.93888565452638417 ) ) ;
#8490=CARTESIAN_POINT ( 'NONE',  ( -32.50000000000000000, 54.00000000000000711, 0.000000000000000000 ) ) ;
#8494=ORIENTED_EDGE ( 'NONE', *, *, #10556, .T. ) ;
#8495=CARTESIAN_POINT ( 'NONE',  ( 20.75514604977248467, 64.67500000273118133, -28.56700777964554305 ) ) ;
#8496=CARTESIAN_POINT ( 'NONE',  ( -26.29305231718579350, 61.80000000000000426, -19.10302069950537884 ) ) ;
#8500=CARTESIAN_POINT ( 'NONE',  ( 10.37757302488624767, 39.72500000273119980, 31.93888565452638417 ) ) ;
#8504=CARTESIAN_POINT ( 'NONE',  ( 1.093617666956751375E-13, 60.00000000546238255, -32.50000000000000711 ) ) ;
#8525=CARTESIAN_POINT ( 'NONE',  ( -33.58253175000000113, 47.37500000273119127, 0.000000000000000000 ) ) ;
#8531=CARTESIAN_POINT ( 'NONE',  ( -32.50000000000000000, 71.89999999999999147, -10.55989012756945478 ) ) ;
#8533=CARTESIAN_POINT ( 'NONE',  ( 33.58253175000000823, 10.02500000273118275, 10.91162601494192863 ) ) ;
#8543=CARTESIAN_POINT ( 'NONE',  ( -2.162160676586881955E-15, 54.62500000273116996, -35.31076352940723240 ) ) ;
#8559=CARTESIAN_POINT ( 'NONE',  ( -32.50000000000000000, 26.09999999999999076, 10.55989012756946366 ) ) ;
#8569=CARTESIAN_POINT ( 'NONE',  ( 1.076200423132605543E-16, 52.00000000000000711, -46.18802153517007980 ) ) ;
#8572=CARTESIAN_POINT ( 'NONE',  ( -20.75514604977248823, 30.82500000273119767, -28.56700777964554305 ) ) ;
#8576=CARTESIAN_POINT ( 'NONE',  ( -32.50000000000000000, 48.60000000546236976, 10.55989012756946366 ) ) ;
#8580=CARTESIAN_POINT ( 'NONE',  ( -33.58253175000000113, 75.22500000273119269, 10.91162601494193929 ) ) ;
#8585=CARTESIAN_POINT ( 'NONE',  ( -26.29305231718579350, 20.30000000546237970, -19.10302069950537884 ) ) ;
#8594=( NAMED_UNIT ( * ) PLANE_ANGLE_UNIT ( ) SI_UNIT ( $, .RADIAN. ) );
#8602=FACE_OUTER_BOUND ( 'NONE', #9304, .T. ) ;
#8604=CARTESIAN_POINT ( 'NONE',  ( 27.16883889988624290, 70.17500000273118133, 19.73931689729373673 ) ) ;
#8610=CARTESIAN_POINT ( 'NONE',  ( -27.16883889988623935, 45.32500000273119412, 19.73931689729374739 ) ) ;
#8611=CARTESIAN_POINT ( 'NONE',  ( 20.75514604977249178, 10.07500000273119234, 28.56700777964553950 ) ) ;
#8612=CARTESIAN_POINT ( 'NONE',  ( -20.75514604977248112, 59.67500000273118133, 28.56700777964554661 ) ) ;
#8617=CARTESIAN_POINT ( 'NONE',  ( 32.50000000000000000, 67.60000000546237686, -10.55989012756945833 ) ) ;
#8623=CARTESIAN_POINT ( 'NONE',  ( 27.16883889988624290, 50.17500000273118843, 19.73931689729373673 ) ) ;
#8628=CARTESIAN_POINT ( 'NONE',  ( 33.58253175000000113, 16.12500000273119127, -4.112674001490185761E-15 ) ) ;
#8642=CARTESIAN_POINT ( 'NONE',  ( -32.50000000000000000, 11.89999999999998614, -10.55989012756945478 ) ) ;
#8648=CARTESIAN_POINT ( 'NONE',  ( 6.486482029760649416E-15, 65.62500000273116996, 35.31076352940723240 ) ) ;
#8649=CARTESIAN_POINT ( 'NONE',  ( 33.58253175000000113, 32.47500000273117138, -10.91162601494193751 ) ) ;
#8650=CARTESIAN_POINT ( 'NONE',  ( 6.486482029760649416E-15, 17.87500000273119838, 35.31076352940723240 ) ) ;
#8657=CARTESIAN_POINT ( 'NONE',  ( 26.29305231718579350, 52.79999999999999716, 19.10302069950537529 ) ) ;
#8663=CARTESIAN_POINT ( 'NONE',  ( 33.58253175000000823, 68.27500000273120406, 10.91162601494192863 ) ) ;
#8669=CARTESIAN_POINT ( 'NONE',  ( 6.486482029760649416E-15, 35.62500000273119127, 35.31076352940723240 ) ) ;
#8674=CARTESIAN_POINT ( 'NONE',  ( 27.16883889988624290, 66.17500000273116711, 19.73931689729373673 ) ) ;
#8691=CARTESIAN_POINT ( 'NONE',  ( 33.58253175000000113, 50.47500000273117848, -10.91162601494193751 ) ) ;
#8697=CARTESIAN_POINT ( 'NONE',  ( 10.04305231718578817, 71.40000000000000568, -30.90933677959249337 ) ) ;
#8698=CARTESIAN_POINT ( 'NONE',  ( -10.37757302488623701, 9.525000002731195181, 31.93888565452638417 ) ) ;
#8706=ORIENTED_EDGE ( 'NONE', *, *, #20063, .F. ) ;
#8707=CARTESIAN_POINT ( 'NONE',  ( -33.58253175000000113, 55.02500000273118985, -10.91162601494193218 ) ) ;
#8735=CARTESIAN_POINT ( 'NONE',  ( -33.58253175000000113, 29.02500000273119340, -10.91162601494193218 ) ) ;
#8736=CARTESIAN_POINT ( 'NONE',  ( 5.779280353836490358E-15, 57.00000000546238965, 32.49999999999999289 ) ) ;
#8741=CARTESIAN_POINT ( 'NONE',  ( 20.08610463437158344, 47.20000000546238539, 27.64615127144129403 ) ) ;
#8743=LINE ( 'NONE', #21965, #12889 ) ;
#8745=CARTESIAN_POINT ( 'NONE',  ( 6.486482029760649416E-15, 75.62500000273121259, 35.31076352940723240 ) ) ;
#8750=CARTESIAN_POINT ( 'NONE',  ( 10.04305231718579705, 9.100000005462391073, 30.90933677959248982 ) ) ;
#8759=( NAMED_UNIT ( * ) SI_UNIT ( $, .STERADIAN. ) SOLID_ANGLE_UNIT ( ) );
#8767=CARTESIAN_POINT ( 'NONE',  ( 10.37757302488624767, 69.97500000273119269, 31.93888565452638417 ) ) ;
#8772=CARTESIAN_POINT ( 'NONE',  ( -33.58253175000000113, 49.12500000273119127, 0.000000000000000000 ) ) ;
#8773=CARTESIAN_POINT ( 'NONE',  ( 6.486482029760649416E-15, 9.875000002731187720, 35.31076352940723240 ) ) ;
#8774=CARTESIAN_POINT ( 'NONE',  ( -10.37757302488623701, 61.77500000273118985, 31.93888565452638417 ) ) ;
#8778=CARTESIAN_POINT ( 'NONE',  ( -20.08610463437156923, 68.80000000546236549, 27.64615127144130113 ) ) ;
#8785=CARTESIAN_POINT ( 'NONE',  ( 6.486482029760649416E-15, 45.87500000273117706, 35.31076352940723240 ) ) ;
#8790=CARTESIAN_POINT ( 'NONE',  ( -10.37757302488623701, 17.52500000273120406, 31.93888565452638417 ) ) ;
#8806=CARTESIAN_POINT ( 'NONE',  ( 26.29305231718579350, 12.79999999999999183, 19.10302069950537529 ) ) ;
#8812=CARTESIAN_POINT ( 'NONE',  ( 33.58253175000000113, 66.22500000273120691, -10.91162601494193751 ) ) ;
#8813=CARTESIAN_POINT ( 'NONE',  ( 10.37757302488624056, 32.77500000273118985, -31.93888565452638417 ) ) ;
#8814=CARTESIAN_POINT ( 'NONE',  ( -27.16883889988624290, 17.17500000273118488, -19.73931689729374028 ) ) ;
#8820=CARTESIAN_POINT ( 'NONE',  ( -10.04305231718579172, 49.60000000000001563, -30.90933677959248982 ) ) ;
#8827=CARTESIAN_POINT ( 'NONE',  ( -10.37757302488624411, 66.97500000273119269, -31.93888565452638417 ) ) ;
#8833=CARTESIAN_POINT ( 'NONE',  ( 33.58253175000000113, 34.12500000273117706, -4.112674001490185761E-15 ) ) ;
#8855=CARTESIAN_POINT ( 'NONE',  ( 33.58253175000000113, 48.37500000273119127, -4.112674001490185761E-15 ) ) ;
#8861=CARTESIAN_POINT ( 'NONE',  ( -26.29305231718578995, 66.19999999999998863, 19.10302069950538595 ) ) ;
#8862=CARTESIAN_POINT ( 'NONE',  ( 20.75514604977249178, 7.825000002731194115, 28.56700777964553950 ) ) ;
#8868=CARTESIAN_POINT ( 'NONE',  ( -1.778240108872766143E-15, 54.00000000546237544, -32.49999999999999289 ) ) ;
#8873=CARTESIAN_POINT ( 'NONE',  ( 33.58253175000000113, 54.12500000273119838, -4.112674001490185761E-15 ) ) ;
#8874=CARTESIAN_POINT ( 'NONE',  ( 27.16883889988624290, 28.17500000273119554, 19.73931689729373673 ) ) ;
#8899=DIRECTION ( 'NONE',  ( 0.000000000000000000, 0.000000000000000000, 1.000000000000000000 ) ) ;
#8901=CARTESIAN_POINT ( 'NONE',  ( -20.75514604977248112, 31.42500000273120619, 28.56700777964554661 ) ) ;
#8902=CARTESIAN_POINT ( 'NONE',  ( -20.08610463437157989, 56.20000000546238539, -27.64615127144129758 ) ) ;
#8904=CARTESIAN_POINT ( 'NONE',  ( 5.779280353836490358E-15, 60.49999999999998579, 32.49999999999999289 ) ) ;
#8906=CARTESIAN_POINT ( 'NONE',  ( -20.08610463437156923, 46.80000000546235839, 27.64615127144130113 ) ) ;
#8910=EDGE_LOOP ( 'NONE', ( #20164, #133, #31042, #47 ) ) ;
#8912=CARTESIAN_POINT ( 'NONE',  ( 20.75514604977248467, 72.42500000273119554, -28.56700777964554305 ) ) ;
#8915=EDGE_LOOP ( 'NONE', ( #19482, #9686, #23244, #18097 ) ) ;
#8917=CARTESIAN_POINT ( 'NONE',  ( 26.29305231718579350, 13.30000000546237260, 19.10302069950537529 ) ) ;
#8925=CARTESIAN_POINT ( 'NONE',  ( -32.50000000000000000, 62.50000000546239676, 0.000000000000000000 ) ) ;
#8929=CARTESIAN_POINT ( 'NONE',  ( 26.29305231718579350, 36.79999999999998295, 19.10302069950537529 ) ) ;
#8940=CARTESIAN_POINT ( 'NONE',  ( 33.58253175000000113, 70.47500000273117848, -10.91162601494193751 ) ) ;
#8945=CARTESIAN_POINT ( 'NONE',  ( -20.75514604977248823, 46.82500000273117990, -28.56700777964554305 ) ) ;
#8946=CARTESIAN_POINT ( 'NONE',  ( -33.58253175000000113, 9.275000002731177418, -10.91162601494193218 ) ) ;
#8947=CARTESIAN_POINT ( 'NONE',  ( 6.486482029760648627E-15, 59.87500000273118417, 35.31076352940722529 ) ) ;
#8951=CARTESIAN_POINT ( 'NONE',  ( 10.04305231718579705, 69.10000000546239107, 30.90933677959248982 ) ) ;
#8957=CARTESIAN_POINT ( 'NONE',  ( 27.16883889988624290, 40.17500000273120975, 19.73931689729373673 ) ) ;
#8958=CARTESIAN_POINT ( 'NONE',  ( 26.29305231718579350, 27.30000000546238681, 19.10302069950537529 ) ) ;
#8960=CARTESIAN_POINT ( 'NONE',  ( 10.37757302488624767, 15.72500000273117848, 31.93888565452638417 ) ) ;
#8977=CARTESIAN_POINT ( 'NONE',  ( -20.08610463437156923, 12.29999999999999183, 27.64615127144130113 ) ) ;
#8983=CARTESIAN_POINT ( 'NONE',  ( 10.37757302488624056, 64.52500000273118985, -31.93888565452638417 ) ) ;
#8984=CARTESIAN_POINT ( 'NONE',  ( 33.58253175000000823, 28.27500000273118985, 10.91162601494192863 ) ) ;
#8986=CARTESIAN_POINT ( 'NONE',  ( 33.58253175000000823, 14.27500000273119340, 10.91162601494192863 ) ) ;
#8992=CARTESIAN_POINT ( 'NONE',  ( -20.08610463437156923, 50.30000000000001137, 27.64615127144130113 ) ) ;
#8993=CARTESIAN_POINT ( 'NONE',  ( 32.50000000000000711, 57.40000000546237402, 10.55989012756945122 ) ) ;
#8997=CARTESIAN_POINT ( 'NONE',  ( 33.58253175000000113, 62.47500000273118559, -10.91162601494193751 ) ) ;
#9002=CARTESIAN_POINT ( 'NONE',  ( -27.16883889988624290, 36.92500000273117422, -19.73931689729374028 ) ) ;
#9005=VERTEX_POINT ( 'NONE', #3908 ) ;
#9008=CARTESIAN_POINT ( 'NONE',  ( 6.277390505771533514E-15, 1.000000005462384323, 34.17252228774368916 ) ) ;
#9019=DIRECTION ( 'NONE',  ( 0.000000000000000000, 1.000000000000000000, 0.000000000000000000 ) ) ;
#9024=CARTESIAN_POINT ( 'NONE',  ( -2.162160676586881955E-15, 48.87500000273117706, -35.31076352940723240 ) ) ;
#9031=CARTESIAN_POINT ( 'NONE',  ( 20.08610463437157279, 67.30000000000001137, -27.64615127144129758 ) ) ;
#9032=CARTESIAN_POINT ( 'NONE',  ( 20.75514604977249178, 9.825000002731188786, 28.56700777964553950 ) ) ;
#9042=CARTESIAN_POINT ( 'NONE',  ( -27.16883889988623935, 53.32500000273120122, 19.73931689729374739 ) ) ;
#9043=CARTESIAN_POINT ( 'NONE',  ( 20.75514604977248467, 26.67500000273118133, -28.56700777964554305 ) ) ;
#9057=CARTESIAN_POINT ( 'NONE',  ( -2.162160676586882350E-15, 56.62500000273116996, -35.31076352940722529 ) ) ;
#9072=CARTESIAN_POINT ( 'NONE',  ( -27.16883889988623935, 25.32500000273117635, 19.73931689729374739 ) ) ;
#9077=CARTESIAN_POINT ( 'NONE',  ( -26.29305231718578995, 46.70000000546238539, 19.10302069950538595 ) ) ;
#9081=CARTESIAN_POINT ( 'NONE',  ( 20.75514604977249178, 75.82500000273118701, 28.56700777964553950 ) ) ;
#9087=CARTESIAN_POINT ( 'NONE',  ( 32.50000000000000000, 13.60000000546239285, -10.55989012756945833 ) ) ;
#9097=CARTESIAN_POINT ( 'NONE',  ( -32.50000000000000000, 35.99999999999999289, 0.000000000000000000 ) ) ;
#9109=CARTESIAN_POINT ( 'NONE',  ( 33.58253175000000823, 46.02500000273118275, 10.91162601494192863 ) ) ;
#9110=CARTESIAN_POINT ( 'NONE',  ( 33.58253175000000113, 2.475000002731187809, -10.91162601494193751 ) ) ;
#9111=CARTESIAN_POINT ( 'NONE',  ( 6.486482029760648627E-15, 63.87500000273119127, 35.31076352940722529 ) ) ;
#9115=CARTESIAN_POINT ( 'NONE',  ( 10.04305231718579705, 65.10000000546239107, 30.90933677959248982 ) ) ;
#9118=CARTESIAN_POINT ( 'NONE',  ( 1.076200423132605543E-16, 52.00000000000000711, -46.18802153517007980 ) ) ;
#9121=CARTESIAN_POINT ( 'NONE',  ( 33.58253175000000823, 44.27500000273120406, 10.91162601494192863 ) ) ;
#9123=CARTESIAN_POINT ( 'NONE',  ( 32.50000000000000000, 31.60000000546237686, -10.55989012756945833 ) ) ;
#9132=LINE ( 'NONE', #29232, #2628 ) ;
#9141=CARTESIAN_POINT ( 'NONE',  ( -2.092463501923844636E-15, 3.500000000000005329, -34.17252228774368916 ) ) ;
#9147=CARTESIAN_POINT ( 'NONE',  ( 33.58253175000000113, 64.12500000273118417, -4.112674001490185761E-15 ) ) ;
#9148=CARTESIAN_POINT ( 'NONE',  ( -27.16883889988623935, 27.57500000273117990, 19.73931689729374739 ) ) ;
#9149=CARTESIAN_POINT ( 'NONE',  ( 20.75514604977249178, 16.07500000273119412, 28.56700777964553950 ) ) ;
#9155=CARTESIAN_POINT ( 'NONE',  ( -32.50000000000000000, 48.09999999999999432, 10.55989012756946366 ) ) ;
#9160=CARTESIAN_POINT ( 'NONE',  ( -27.16883889988624290, 63.17500000273117422, -19.73931689729374028 ) ) ;
#9165=CARTESIAN_POINT ( 'NONE',  ( -2.162160676586881955E-15, 32.62500000273119838, -35.31076352940723240 ) ) ;
#9186=CARTESIAN_POINT ( 'NONE',  ( -20.75514604977248112, 47.67500000273118843, 28.56700777964554661 ) ) ;
#9191=CARTESIAN_POINT ( 'NONE',  ( 10.04305231718578817, 69.40000000000000568, -30.90933677959249337 ) ) ;
#9196=FACE_OUTER_BOUND ( 'NONE', #15740, .T. ) ;
#9201=CARTESIAN_POINT ( 'NONE',  ( -2.162160676586881955E-15, 52.62500000273117706, -35.31076352940723240 ) ) ;
#9202=CARTESIAN_POINT ( 'NONE',  ( 20.75514604977248467, 20.67500000273119909, -28.56700777964554305 ) ) ;
#9218=CARTESIAN_POINT ( 'NONE',  ( 27.16883889988623935, 56.32500000273120122, -19.73931689729374384 ) ) ;
#9230=CARTESIAN_POINT ( 'NONE',  ( 26.29305231718578995, 63.70000000546237118, -19.10302069950538240 ) ) ;
#9232=CARTESIAN_POINT ( 'NONE',  ( -27.16883889988624290, 18.92500000273118843, -19.73931689729374028 ) ) ;
#9235=CARTESIAN_POINT ( 'NONE',  ( 26.29305231718578995, 61.20000000000001705, -19.10302069950538240 ) ) ;
#9237=CARTESIAN_POINT ( 'NONE',  ( -26.29305231718579350, 48.30000000546237970, -19.10302069950537884 ) ) ;
#9242=CARTESIAN_POINT ( 'NONE',  ( 33.58253175000000823, 74.02500000273120406, 10.91162601494192863 ) ) ;
#9245=PLANE ( 'NONE',  #15191 ) ;
#9248=CARTESIAN_POINT ( 'NONE',  ( 20.08610463437158344, 11.20000000546238184, 27.64615127144129403 ) ) ;
#9259=CARTESIAN_POINT ( 'NONE',  ( 10.04305231718579705, 34.60000000000000853, 30.90933677959248982 ) ) ;
#9267=ORIENTED_EDGE ( 'NONE', *, *, #32213, .F. ) ;
#9271=CARTESIAN_POINT ( 'NONE',  ( -33.58253175000000113, 49.02500000273116854, -10.91162601494193218 ) ) ;
#9272=CARTESIAN_POINT ( 'NONE',  ( -10.37757302488623701, 5.775000002731192517, 31.93888565452638417 ) ) ;
#9273=CARTESIAN_POINT ( 'NONE',  ( -10.37757302488623701, 53.77500000273120406, 31.93888565452638417 ) ) ;
#9277=CARTESIAN_POINT ( 'NONE',  ( -32.50000000000000000, 64.50000000546239676, 0.000000000000000000 ) ) ;
#9280=CARTESIAN_POINT ( 'NONE',  ( -32.50000000000000000, 53.90000000000001279, -10.55989012756945300 ) ) ;
#9283=CARTESIAN_POINT ( 'NONE',  ( 33.58253175000000823, 42.27500000273118275, 10.91162601494192863 ) ) ;
#9285=CARTESIAN_POINT ( 'NONE',  ( 32.50000000000000000, 29.50000000546236478, -3.980102097228898626E-15 ) ) ;
#9302=CARTESIAN_POINT ( 'NONE',  ( 22.23068731925703645, 52.00000000000002132, 25.26668985625460095 ) ) ;
#9303=CARTESIAN_POINT ( 'NONE',  ( -10.37757302488624411, 78.97500000273120691, -31.93888565452638417 ) ) ;
#9304=EDGE_LOOP ( 'NONE', ( #20510, #12779, #2816, #31753 ) ) ;
#9308=CARTESIAN_POINT ( 'NONE',  ( 27.16883889988624290, 67.92500000273120975, 19.73931689729373673 ) ) ;
#9309=CARTESIAN_POINT ( 'NONE',  ( 6.486482029760649416E-15, 23.87500000273117706, 35.31076352940723240 ) ) ;
#9310=CARTESIAN_POINT ( 'NONE',  ( 33.58253175000000113, 14.47500000273118737, -10.91162601494193751 ) ) ;
#9315=CARTESIAN_POINT ( 'NONE',  ( 10.04305231718579705, 50.59999999999999432, 30.90933677959248982 ) ) ;
#9320=CARTESIAN_POINT ( 'NONE',  ( -10.37757302488623701, 61.77500000273118985, 31.93888565452638417 ) ) ;
#9326=CARTESIAN_POINT ( 'NONE',  ( -33.58253175000000113, 31.22500000273118559, 10.91162601494193929 ) ) ;
#9351=CARTESIAN_POINT ( 'NONE',  ( -27.16883889988624290, 45.17500000273118133, -19.73931689729374028 ) ) ;
#9357=CARTESIAN_POINT ( 'NONE',  ( -26.29305231718579350, 65.80000000000001137, -19.10302069950537884 ) ) ;
#9362=CARTESIAN_POINT ( 'NONE',  ( 3.980102097228898626E-15, 52.00000000000000711, -32.50000000000000000 ) ) ;
#9367=CARTESIAN_POINT ( 'NONE',  ( -27.16883889988624290, 50.92500000273118843, -19.73931689729374028 ) ) ;
#9368=CARTESIAN_POINT ( 'NONE',  ( 33.58253175000000823, 22.27500000273116854, 10.91162601494192863 ) ) ;
#9384=CARTESIAN_POINT ( 'NONE',  ( -27.16883889988624290, 52.92500000273118843, -19.73931689729374028 ) ) ;
#9399=CARTESIAN_POINT ( 'NONE',  ( -33.58253175000000113, 21.22500000273117848, 10.91162601494193929 ) ) ;
#9402=CARTESIAN_POINT ( 'NONE',  ( 20.08610463437157279, 55.80000000546236549, -27.64615127144129758 ) ) ;
#9405=CARTESIAN_POINT ( 'NONE',  ( -26.29305231718578995, 42.70000000546238539, 19.10302069950538595 ) ) ;
#9411=CARTESIAN_POINT ( 'NONE',  ( -33.58253175000000113, 71.02500000273118985, -10.91162601494193218 ) ) ;
#9417=CARTESIAN_POINT ( 'NONE',  ( -32.50000000000000000, 8.400000005462368691, -10.55989012756945478 ) ) ;
#9427=CARTESIAN_POINT ( 'NONE',  ( 26.29305231718579350, 32.80000000000001137, 19.10302069950537529 ) ) ;
#9443=CARTESIAN_POINT ( 'NONE',  ( 20.75514604977249178, 39.82500000273116569, 28.56700777964553950 ) ) ;
#9444=CARTESIAN_POINT ( 'NONE',  ( -33.58253175000000113, 3.275000002731191628, -10.91162601494193218 ) ) ;
#9445=CARTESIAN_POINT ( 'NONE',  ( -20.75514604977248112, 53.67500000273119554, 28.56700777964554661 ) ) ;
#9450=CARTESIAN_POINT ( 'NONE',  ( -20.08610463437157989, 62.20000000546237828, -27.64615127144129758 ) ) ;
#9456=CARTESIAN_POINT ( 'NONE',  ( -33.58253175000000113, 39.37500000273118417, 0.000000000000000000 ) ) ;
#9460=CARTESIAN_POINT ( 'NONE',  ( 10.04305231718578817, 31.90000000546237757, -30.90933677959249337 ) ) ;
#9472=CARTESIAN_POINT ( 'NONE',  ( 33.58253175000000823, 66.02500000273118985, 10.91162601494192685 ) ) ;
#9482=CARTESIAN_POINT ( 'NONE',  ( -2.092463501923844636E-15, 5.500000000000000888, -34.17252228774368916 ) ) ;
#9487=CARTESIAN_POINT ( 'NONE',  ( 20.75514604977248467, 60.42500000273118133, -28.56700777964554305 ) ) ;
#9488=CARTESIAN_POINT ( 'NONE',  ( -10.37757302488623701, 25.77500000273118275, 31.93888565452638417 ) ) ;
#9489=CARTESIAN_POINT ( 'NONE',  ( -20.75514604977248823, 11.07500000273119056, -28.56700777964554305 ) ) ;
#9496=CARTESIAN_POINT ( 'NONE',  ( 20.08610463437158344, 44.69999999999998153, 27.64615127144129403 ) ) ;
#9502=CARTESIAN_POINT ( 'NONE',  ( 20.75514604977249178, 58.07500000273117990, 28.56700777964553950 ) ) ;
#9507=CARTESIAN_POINT ( 'NONE',  ( -27.16883889988624290, 32.92500000273117422, -19.73931689729374028 ) ) ;
#9529=CARTESIAN_POINT ( 'NONE',  ( -33.58253175000000113, 79.12500000273118417, 0.000000000000000000 ) ) ;
#9530=CARTESIAN_POINT ( 'NONE',  ( 33.58253175000000113, 40.47500000273118559, -10.91162601494193751 ) ) ;
#9535=CARTESIAN_POINT ( 'NONE',  ( -26.29305231718579350, 67.80000000000001137, -19.10302069950537884 ) ) ;
#9546=CARTESIAN_POINT ( 'NONE',  ( 33.58253175000000113, 48.22500000273119269, -10.91162601494193751 ) ) ;
#9548=CARTESIAN_POINT ( 'NONE',  ( -33.58253175000000113, 25.27500000273119696, -10.91162601494193218 ) ) ;
#9574=CARTESIAN_POINT ( 'NONE',  ( 10.37757302488624767, 59.97500000273119269, 31.93888565452638417 ) ) ;
#9580=CARTESIAN_POINT ( 'NONE',  ( 5.147494310547426899, 63.94874572391552903, -32.50000000000000000 ) ) ;
#9582=CARTESIAN_POINT ( 'NONE',  ( -10.37757302488623701, 21.52500000273117919, 31.93888565452638417 ) ) ;
#9586=CARTESIAN_POINT ( 'NONE',  ( 10.04305231718578817, 41.90000000546238823, -30.90933677959249337 ) ) ;
#9591=CARTESIAN_POINT ( 'NONE',  ( -2.162160676586881955E-15, 70.62500000273118417, -35.31076352940723240 ) ) ;
#9598=CARTESIAN_POINT ( 'NONE',  ( -10.37757302488623701, 13.52500000273119873, 31.93888565452638417 ) ) ;
#9607=SHAPE_REPRESENTATION_RELATIONSHIP ( 'NONE' , 'NONE' ,  #31529, #10725 ) ;
#9608=CARTESIAN_POINT ( 'NONE',  ( -32.50000000000000000, 33.90000000000001279, -10.55989012756945478 ) ) ;
#9612=CARTESIAN_POINT ( 'NONE',  ( 5.147494310547434893, 62.55125428154684641, 32.49999999999999289 ) ) ;
#9615=VERTEX_POINT ( 'NONE', #28901 ) ;
#9618=( GEOMETRIC_REPRESENTATION_CONTEXT ( 3 ) GLOBAL_UNCERTAINTY_ASSIGNED_CONTEXT ( ( #16812 ) ) GLOBAL_UNIT_ASSIGNED_CONTEXT ( ( #6530, #8594, #19911 ) ) REPRESENTATION_CONTEXT ( 'NONE', 'WORKASPACE' ) );
#9621=CARTESIAN_POINT ( 'NONE',  ( -2.162160676586881955E-15, 42.62500000273119838, -35.31076352940723240 ) ) ;
#9622=CARTESIAN_POINT ( 'NONE',  ( -20.75514604977248823, 7.075000002731188786, -28.56700777964554305 ) ) ;
#9623=CARTESIAN_POINT ( 'NONE',  ( -20.75514604977248823, 57.07500000273117990, -28.56700777964554305 ) ) ;
#9626=CARTESIAN_POINT ( 'NONE',  ( 10.04305231718578817, 57.90000000546240244, -30.90933677959249337 ) ) ;
#9633=CARTESIAN_POINT ( 'NONE',  ( 27.16883889988624290, 42.17500000273118133, 19.73931689729373673 ) ) ;
#9637=CARTESIAN_POINT ( 'NONE',  ( 10.04305231718579705, 31.10000000546238397, 30.90933677959248982 ) ) ;
#9641=EDGE_CURVE ( 'NONE', #9615, #25517, #29700, .T. ) ;
#9649=CARTESIAN_POINT ( 'NONE',  ( 33.58253175000000113, 66.22500000273120691, -10.91162601494193574 ) ) ;
#9657=CARTESIAN_POINT ( 'NONE',  ( 0.000000000000000000, 52.00000000000000711, 0.000000000000000000 ) ) ;
#9659=CARTESIAN_POINT ( 'NONE',  ( 27.16883889988624290, 78.17500000273118133, 19.73931689729373673 ) ) ;
#9664=CARTESIAN_POINT ( 'NONE',  ( -10.37757302488624411, 60.72500000273119269, -31.93888565452638417 ) ) ;
#9665=CARTESIAN_POINT ( 'NONE',  ( 27.16883889988623935, 24.57500000273120477, -19.73931689729374384 ) ) ;
#9666=CARTESIAN_POINT ( 'NONE',  ( -27.16883889988624290, 13.17500000273118310, -19.73931689729374028 ) ) ;
#9670=CARTESIAN_POINT ( 'NONE',  ( 32.50000000000000711, 77.40000000546240244, 10.55989012756945122 ) ) ;
#9673=CARTESIAN_POINT ( 'NONE',  ( -20.08610463437156923, 44.30000000000000426, 27.64615127144130113 ) ) ;
#9676=ORIENTED_EDGE ( 'NONE', *, *, #33754, .T. ) ;
#9677=CARTESIAN_POINT ( 'NONE',  ( -27.16883889988623935, 57.57500000273117990, 19.73931689729374739 ) ) ;
#9681=VERTEX_POINT ( 'NONE', #10549 ) ;
#9682=CARTESIAN_POINT ( 'NONE',  ( 33.58253175000000113, 32.22500000273117848, -10.91162601494193751 ) ) ;
#9686=ORIENTED_EDGE ( 'NONE', *, *, #26712, .T. ) ;
#9703=CARTESIAN_POINT ( 'NONE',  ( -10.37757302488624411, 76.72500000273117848, -31.93888565452638417 ) ) ;
#9704=CARTESIAN_POINT ( 'NONE',  ( -33.58253175000000113, 45.37500000273119127, 0.000000000000000000 ) ) ;
#9709=CARTESIAN_POINT ( 'NONE',  ( 32.50000000000000000, 59.09999999999999432, -10.55989012756945833 ) ) ;
#9718=CARTESIAN_POINT ( 'NONE',  ( -20.75514604977248823, 48.82500000273117280, -28.56700777964554305 ) ) ;
#9719=CARTESIAN_POINT ( 'NONE',  ( -20.75514604977248112, 23.67500000273118843, 28.56700777964554661 ) ) ;
#9731=CARTESIAN_POINT ( 'NONE',  ( 32.50000000000000000, 66.99999999999998579, -3.980102097228898626E-15 ) ) ;
#9742=CARTESIAN_POINT ( 'NONE',  ( -2.162160676586881955E-15, 60.87500000273116996, -35.31076352940723240 ) ) ;
#9750=CARTESIAN_POINT ( 'NONE',  ( -33.58253175000000113, 23.12500000273119838, 0.000000000000000000 ) ) ;
#9755=CARTESIAN_POINT ( 'NONE',  ( -32.50000000000000000, 42.60000000546238397, 10.55989012756946366 ) ) ;
#9761=CARTESIAN_POINT ( 'NONE',  ( 10.37757302488624767, 67.72500000273116427, 31.93888565452638417 ) ) ;
#9768=CARTESIAN_POINT ( 'NONE',  ( 10.37757302488624056, 10.52500000273119696, -31.93888565452638417 ) ) ;
#9781=CARTESIAN_POINT ( 'NONE',  ( 32.50000000000000000, 27.09999999999999076, -10.55989012756945833 ) ) ;
#9797=CARTESIAN_POINT ( 'NONE',  ( -10.37757302488623701, 41.52500000273119696, 31.93888565452638417 ) ) ;
#9798=CARTESIAN_POINT ( 'NONE',  ( -2.162160676586881955E-15, 4.875000002731200155, -35.31076352940723240 ) ) ;
#9799=CARTESIAN_POINT ( 'NONE',  ( 10.37757302488624056, 56.77500000273121117, -31.93888565452638417 ) ) ;
#9803=CARTESIAN_POINT ( 'NONE',  ( 32.50000000000000000, 63.60000000546238397, -10.55989012756945833 ) ) ;
#9809=CARTESIAN_POINT ( 'NONE',  ( 33.58253175000000113, 34.37500000273117706, -4.112674001490185761E-15 ) ) ;
#9813=CARTESIAN_POINT ( 'NONE',  ( -20.08610463437156923, 22.80000000546236194, 27.64615127144130113 ) ) ;
#9830=FACE_OUTER_BOUND ( 'NONE', #1767, .T. ) ;
#9831=CARTESIAN_POINT ( 'NONE',  ( 20.08610463437158344, 2.700000000000001954, 27.64615127144129403 ) ) ;
#9836=CARTESIAN_POINT ( 'NONE',  ( 20.75514604977249178, 59.82500000273117280, 28.56700777964553950 ) ) ;
#9837=CARTESIAN_POINT ( 'NONE',  ( -33.58253175000000113, 25.47500000273118914, 10.91162601494193929 ) ) ;
#9838=CARTESIAN_POINT ( 'NONE',  ( 10.37757302488624056, 10.77500000273116854, -31.93888565452638417 ) ) ;
#9843=CARTESIAN_POINT ( 'NONE',  ( 33.58253175000000113, 4.125000002731193938, -4.112674001490185761E-15 ) ) ;
#9844=EDGE_CURVE ( 'NONE', #24911, #29266, #14638, .T. ) ;
#9846=CARTESIAN_POINT ( 'NONE',  ( -32.50000000000000000, 39.89999999999999858, -10.55989012756945478 ) ) ;
#9851=CARTESIAN_POINT ( 'NONE',  ( -33.58253175000000113, 57.27500000273120406, -10.91162601494193218 ) ) ;
#9855=ORIENTED_EDGE ( 'NONE', *, *, #19956, .F. ) ;
#9856=CARTESIAN_POINT ( 'NONE',  ( -27.16883889988623935, 29.32500000273117990, 19.73931689729374739 ) ) ;
#9876=CARTESIAN_POINT ( 'NONE',  ( 10.37757302488624767, 41.97500000273117138, 31.93888565452638417 ) ) ;
#9882=CARTESIAN_POINT ( 'NONE',  ( 26.29305231718579350, 62.80000000000001137, 19.10302069950537529 ) ) ;
#9883=CARTESIAN_POINT ( 'NONE',  ( 0.000000000000000000, 52.00000000000000711, 0.000000000000000000 ) ) ;
#9889=CARTESIAN_POINT ( 'NONE',  ( 27.16883889988623935, 76.57500000273120122, -19.73931689729374384 ) ) ;
#9894=CARTESIAN_POINT ( 'NONE',  ( 33.58253175000000113, 48.12500000273119127, -4.112674001490185761E-15 ) ) ;
#9895=CARTESIAN_POINT ( 'NONE',  ( -20.75514604977248112, 21.67500000273119554, 28.56700777964554661 ) ) ;
#9907=CARTESIAN_POINT ( 'NONE',  ( -12.90513655866680587, 66.99999999999998579, -31.00393344628902881 ) ) ;
#9919=CARTESIAN_POINT ( 'NONE',  ( 10.37757302488624767, 63.97500000273119269, 31.93888565452638417 ) ) ;
#9925=CARTESIAN_POINT ( 'NONE',  ( 26.29305231718578995, 77.20000000000000284, -19.10302069950538240 ) ) ;
#9926=CARTESIAN_POINT ( 'NONE',  ( -10.37757302488624411, 22.72500000273118559, -31.93888565452638417 ) ) ;
#9929=CARTESIAN_POINT ( 'NONE',  ( 0.000000000000000000, 52.00000000000000711, 32.50000000000000000 ) ) ;
#9931=CARTESIAN_POINT ( 'NONE',  ( -32.50000000000000000, 38.60000000546239818, 10.55989012756946366 ) ) ;
#9937=ORIENTED_EDGE ( 'NONE', *, *, #32022, .F. ) ;
#9938=CARTESIAN_POINT ( 'NONE',  ( 27.16883889988624290, 71.92500000273120975, 19.73931689729373673 ) ) ;
#9945=CARTESIAN_POINT ( 'NONE',  ( 27.16883889988624290, 9.925000002731207971, 19.73931689729373673 ) ) ;
#9955=CARTESIAN_POINT ( 'NONE',  ( 26.29305231718579350, 28.80000000000000782, 19.10302069950537529 ) ) ;
#9959=CARTESIAN_POINT ( 'NONE',  ( 10.04305231718579705, 62.60000000000000142, 30.90933677959248982 ) ) ;
#9969=CARTESIAN_POINT ( 'NONE',  ( 10.37757302488624767, 43.72500000273120691, 31.93888565452638417 ) ) ;
#9971=CARTESIAN_POINT ( 'NONE',  ( -10.37757302488624411, 56.97500000273118559, -31.93888565452638417 ) ) ;
#9975=CARTESIAN_POINT ( 'NONE',  ( -10.04305231718578462, 60.90000000546237402, 30.90933677959249337 ) ) ;
#9977=CARTESIAN_POINT ( 'NONE',  ( -1.778240108872766143E-15, 58.00000000546237544, -32.49999999999999289 ) ) ;
#9979=( BOUNDED_CURVE ( )  B_SPLINE_CURVE ( 2, ( #1539, #23174, #33636, #4805, #30365, #18039, #33109, #4292, #12360, #33460, #9959, #9612, #1706 ),
 .UNSPECIFIED., .F., .T. ) 
 B_SPLINE_CURVE_WITH_KNOTS ( ( 3, 2, 2, 2, 2, 2, 3 ),
 ( 0.2115384615384615363, 0.2128205128205128138, 0.2153846153846153966, 0.2179487179487179516, 0.2205128205128205066, 0.2230769230769230893, 0.2243589743589743668 ),
 .UNSPECIFIED. ) 
 CURVE ( )  GEOMETRIC_REPRESENTATION_ITEM ( )  RATIONAL_B_SPLINE_CURVE ( ( 0.9755282581475768211, 0.9755282581475768211, 1.000000000000000000, 0.9510565162951535312, 1.000000000000000000, 0.9510565162951535312, 1.000000000000000000, 0.9510565162951535312, 1.000000000000000000, 0.9510565162951535312, 1.000000000000000000, 0.9755282581475768211, 0.9755282581475768211 ) ) 
 REPRESENTATION_ITEM ( '' )  );
#9984=CARTESIAN_POINT ( 'NONE',  ( 27.16883889988623935, 36.57500000273118701, -19.73931689729374384 ) ) ;
#9989=CARTESIAN_POINT ( 'NONE',  ( 10.04305231718578817, 21.90000000546237047, -30.90933677959249337 ) ) ;
#10000=CARTESIAN_POINT ( 'NONE',  ( -27.16883889988624290, 58.92500000273119554, -19.73931689729374028 ) ) ;
#10012=CARTESIAN_POINT ( 'NONE',  ( 33.58253175000000113, 76.47500000273117848, -10.91162601494193751 ) ) ;
#10017=CARTESIAN_POINT ( 'NONE',  ( -20.75514604977248823, 60.82500000273121543, -28.56700777964554305 ) ) ;
#10018=CARTESIAN_POINT ( 'NONE',  ( 10.37757302488624056, 20.77500000273117919, -31.93888565452638417 ) ) ;
#10019=CARTESIAN_POINT ( 'NONE',  ( 33.58253175000000823, 12.27500000273118452, 10.91162601494192863 ) ) ;
#10023=CARTESIAN_POINT ( 'NONE',  ( 33.58253175000000113, 2.225000002731181592, -10.91162601494193751 ) ) ;
#10025=CARTESIAN_POINT ( 'NONE',  ( -32.50000000000000000, 42.09999999999997300, 10.55989012756946366 ) ) ;
#10030=CARTESIAN_POINT ( 'NONE',  ( -27.16883889988623935, 53.57500000273117280, 19.73931689729374739 ) ) ;
#10036=CARTESIAN_POINT ( 'NONE',  ( 20.75514604977248467, 24.42500000273119554, -28.56700777964554305 ) ) ;
#10053=CARTESIAN_POINT ( 'NONE',  ( -20.75514604977248112, 77.42500000273119554, 28.56700777964554661 ) ) ;
#10054=CARTESIAN_POINT ( 'NONE',  ( -10.37757302488623701, 43.77500000273119696, 31.93888565452638417 ) ) ;
#10060=CARTESIAN_POINT ( 'NONE',  ( 20.08610463437158344, 58.70000000000000995, 27.64615127144129403 ) ) ;
#10064=CARTESIAN_POINT ( 'NONE',  ( -10.37757302488623701, 73.77500000273120406, 31.93888565452638417 ) ) ;
#10069=CARTESIAN_POINT ( 'NONE',  ( 20.75514604977248467, 44.42500000273120264, -28.56700777964554305 ) ) ;
#10072=DIRECTION ( 'NONE',  ( 0.000000000000000000, 0.000000000000000000, 1.000000000000000000 ) ) ;
#10073=CARTESIAN_POINT ( 'NONE',  ( 10.04305231718579705, 5.100000005462374197, 30.90933677959248982 ) ) ;
#10096=CARTESIAN_POINT ( 'NONE',  ( -10.37757302488624411, 62.97500000273119269, -31.93888565452638417 ) ) ;
#10101=CARTESIAN_POINT ( 'NONE',  ( 32.50000000000000000, 77.00000000000000000, -3.980102097228898626E-15 ) ) ;
#10102=CARTESIAN_POINT ( 'NONE',  ( 20.75514604977248467, 14.42500000273119021, -28.56700777964554305 ) ) ;
#10105=CLOSED_SHELL ( 'NONE', ( #25625, #6835, #20931, #10408, #7750, #3421, #21827, #13530, #23304, #28199, #19493, #5189, #12156, #29681, #29828, #31587, #27193, #4853, #13262, #25709, #26367, #16701, #4459, #7122, #33155, #13221, #26664 ) ) ;
#10108=CARTESIAN_POINT ( 'NONE',  ( -32.50000000000000000, 44.50000000546237544, 0.000000000000000000 ) ) ;
#10114=CARTESIAN_POINT ( 'NONE',  ( -27.16883889988624290, 70.92500000273120975, -19.73931689729374028 ) ) ;
#10120=CARTESIAN_POINT ( 'NONE',  ( 33.58253175000000113, 10.12500000273118594, -4.112674001490185761E-15 ) ) ;
#10131=CARTESIAN_POINT ( 'NONE',  ( -32.50000000000000000, 30.00000000000001421, 0.000000000000000000 ) ) ;
#10142=CARTESIAN_POINT ( 'NONE',  ( 25.10896554811106540, 66.99999999999997158, -21.28139962774331906 ) ) ;
#10143=CARTESIAN_POINT ( 'NONE',  ( -20.75514604977248112, 33.42500000273120264, 28.56700777964554661 ) ) ;
#10144=FACE_OUTER_BOUND ( 'NONE', #7915, .T. ) ;
#10148=CARTESIAN_POINT ( 'NONE',  ( 10.04305231718579705, 61.10000000546238397, 30.90933677959248982 ) ) ;
#10156=CARTESIAN_POINT ( 'NONE',  ( -33.58253175000000113, 37.37500000273118417, 0.000000000000000000 ) ) ;
#10160=CARTESIAN_POINT ( 'NONE',  ( -10.04305231718579172, 22.10000000546237686, -30.90933677959248982 ) ) ;
#10172=CARTESIAN_POINT ( 'NONE',  ( 27.16883889988624290, 63.92500000273120264, 19.73931689729373673 ) ) ;
#10174=( GEOMETRIC_REPRESENTATION_CONTEXT ( 3 ) GLOBAL_UNCERTAINTY_ASSIGNED_CONTEXT ( ( #29833 ) ) GLOBAL_UNIT_ASSIGNED_CONTEXT ( ( #30188, #3785, #8759 ) ) REPRESENTATION_CONTEXT ( 'NONE', 'WORKASPACE' ) );
#10183=CARTESIAN_POINT ( 'NONE',  ( 20.75514604977248467, 72.67500000273118133, -28.56700777964554305 ) ) ;
#10189=CARTESIAN_POINT ( 'NONE',  ( -33.58253175000000113, 57.22500000273117848, 10.91162601494193929 ) ) ;
#10190=CARTESIAN_POINT ( 'NONE',  ( 33.58253175000000113, 16.47500000273118204, -10.91162601494193751 ) ) ;
#10191=CARTESIAN_POINT ( 'NONE',  ( -20.75514604977248112, 7.675000002731199089, 28.56700777964554661 ) ) ;
#10198=CARTESIAN_POINT ( 'NONE',  ( -26.29305231718579350, 78.30000000546237970, -19.10302069950537884 ) ) ;
#10199=CARTESIAN_POINT ( 'NONE',  ( 30.28308157046064153, 52.00000000000001421, -13.46430247876119601 ) ) ;
#10200=CARTESIAN_POINT ( 'NONE',  ( -20.08610463437156923, 42.30000000000000426, 27.64615127144130113 ) ) ;
#10205=CARTESIAN_POINT ( 'NONE',  ( -20.75514604977248823, 51.07500000273116569, -28.56700777964554305 ) ) ;
#10209=CARTESIAN_POINT ( 'NONE',  ( -27.16883889988624290, 24.92500000273119198, -19.73931689729374028 ) ) ;
#10225=CARTESIAN_POINT ( 'NONE',  ( 32.50000000000000711, 14.89999999999999680, 10.55989012756945122 ) ) ;
#10231=CARTESIAN_POINT ( 'NONE',  ( 27.16883889988624290, 34.17500000273120264, 19.73931689729373673 ) ) ;
#10236=CARTESIAN_POINT ( 'NONE',  ( 32.50000000000000000, 58.99999999999998579, -3.980102097228898626E-15 ) ) ;
#10240=AXIS2_PLACEMENT_3D ( 'NONE', #8569, #27266, #501 ) ;
#10241=CARTESIAN_POINT ( 'NONE',  ( 27.16883889988623935, 72.57500000273118701, -19.73931689729374384 ) ) ;
#10246=CARTESIAN_POINT ( 'NONE',  ( -33.58253175000000113, 45.12500000273119127, 0.000000000000000000 ) ) ;
#10250=CARTESIAN_POINT ( 'NONE',  ( 26.29305231718579350, 1.300000005462376151, 19.10302069950537529 ) ) ;
#10261=SHAPE_DEFINITION_REPRESENTATION ( #20558, #31529 ) ;
#10268=CARTESIAN_POINT ( 'NONE',  ( -27.16883889988624290, 63.17500000273117422, -19.73931689729374028 ) ) ;
#10276=CARTESIAN_POINT ( 'NONE',  ( -2.162160676586881955E-15, 18.62500000273117351, -35.31076352940723240 ) ) ;
#10281=CARTESIAN_POINT ( 'NONE',  ( 32.50000000000000711, 33.40000000546238113, 10.55989012756945122 ) ) ;
#10287=ORIENTED_EDGE ( 'NONE', *, *, #31033, .T. ) ;
#10288=CARTESIAN_POINT ( 'NONE',  ( -20.75514604977248112, 59.42500000273118843, 28.56700777964554661 ) ) ;
#10294=CARTESIAN_POINT ( 'NONE',  ( 20.75514604977249178, 1.825000002731179460, 28.56700777964553950 ) ) ;
#10303=CARTESIAN_POINT ( 'NONE',  ( -10.04305231718578462, 28.39999999999999503, 30.90933677959249337 ) ) ;
#10314=CARTESIAN_POINT ( 'NONE',  ( -33.58253175000000113, 33.22500000273117138, 10.91162601494193929 ) ) ;
#10315=CARTESIAN_POINT ( 'NONE',  ( 5.147494310547535257, 57.44874571845314648, -32.49999999999996447 ) ) ;
#10319=CARTESIAN_POINT ( 'NONE',  ( -32.50000000000000000, 52.60000000546235555, 10.55989012756946366 ) ) ;
#10320=AXIS2_PLACEMENT_3D ( 'NONE', #1118, #21915, #11438 ) ;
#10323=SURFACE_STYLE_USAGE ( .BOTH. , #13579 ) ;
#10329=CARTESIAN_POINT ( 'NONE',  ( 6.486482029760649416E-15, 37.87500000273117706, 35.31076352940723240 ) ) ;
#10331=ORIENTED_EDGE ( 'NONE', *, *, #6211, .T. ) ;
#10333=CARTESIAN_POINT ( 'NONE',  ( 26.29305231718579350, 23.30000000546238326, 19.10302069950537529 ) ) ;
#10343=CARTESIAN_POINT ( 'NONE',  ( 20.75514604977249178, 59.82500000273117280, 28.56700777964553950 ) ) ;
#10352=CARTESIAN_POINT ( 'NONE',  ( -10.37757302488623701, 73.77500000273120406, 31.93888565452638417 ) ) ;
#10356=CARTESIAN_POINT ( 'NONE',  ( 6.486482029760649416E-15, 53.62500000273119838, 35.31076352940723240 ) ) ;
#10357=CARTESIAN_POINT ( 'NONE',  ( 20.75514604977249178, 20.07500000273118346, 28.56700777964553950 ) ) ;
#10358=CARTESIAN_POINT ( 'NONE',  ( 27.16883889988623935, 2.575000002731184345, -19.73931689729374384 ) ) ;
#10362=CARTESIAN_POINT ( 'NONE',  ( 33.58253175000000823, 4.025000002731196957, 10.91162601494192863 ) ) ;
#10363=CARTESIAN_POINT ( 'NONE',  ( 12.54892211412375680, 52.00000000000002842, -30.22116052075408987 ) ) ;
#10366=CARTESIAN_POINT ( 'NONE',  ( -1.778240108872766143E-15, 64.00000000546238255, -32.49999999999999289 ) ) ;
#10368=CARTESIAN_POINT ( 'NONE',  ( 27.16883889988624290, 52.17500000273118843, 19.73931689729373673 ) ) ;
#10369=CARTESIAN_POINT ( 'NONE',  ( 5.147494310547434893, 59.05125428700922896, 32.49999999999999289 ) ) ;
#10373=CARTESIAN_POINT ( 'NONE',  ( -20.75514604977248823, 22.82500000273118701, -28.56700777964554305 ) ) ;
#10387=CARTESIAN_POINT ( 'NONE',  ( 10.04305231718579705, 14.59999999999998721, 30.90933677959248982 ) ) ;
#10393=CARTESIAN_POINT ( 'NONE',  ( -27.16883889988623935, 71.32500000273118701, 19.73931689729374739 ) ) ;
#10394=CARTESIAN_POINT ( 'NONE',  ( -10.37757302488623701, 33.77500000273118985, 31.93888565452638417 ) ) ;
#10400=CARTESIAN_POINT ( 'NONE',  ( 6.277390505771533514E-15, 62.50000000000000000, 34.17252228774368916 ) ) ;
#10404=CARTESIAN_POINT ( 'NONE',  ( -33.58253175000000113, 75.27500000273118985, -10.91162601494193218 ) ) ;
#10408=ADVANCED_FACE ( 'NONE', ( #28016 ), #20825, .F. ) ;
#10410=CARTESIAN_POINT ( 'NONE',  ( 20.75514604977249178, 45.82500000273118701, 28.56700777964553950 ) ) ;
#10414=CARTESIAN_POINT ( 'NONE',  ( 20.08610463437157279, 3.800000005462383257, -27.64615127144129758 ) ) ;
#10434=CARTESIAN_POINT ( 'NONE',  ( -20.75514604977248823, 53.07500000273118701, -28.56700777964554305 ) ) ;
#10441=CARTESIAN_POINT ( 'NONE',  ( -33.58253175000000113, 17.22500000273118559, 10.91162601494193929 ) ) ;
#10446=CARTESIAN_POINT ( 'NONE',  ( -26.29305231718578995, 36.70000000546237828, 19.10302069950538595 ) ) ;
#10452=CARTESIAN_POINT ( 'NONE',  ( -20.75514604977248823, 62.82500000273119412, -28.56700777964554305 ) ) ;
#10458=CARTESIAN_POINT ( 'NONE',  ( 33.58253175000000823, 2.025000002731187632, 10.91162601494192863 ) ) ;
#10467=CARTESIAN_POINT ( 'NONE',  ( -26.29305231718579350, 27.80000000000000426, -19.10302069950537884 ) ) ;
#10478=CARTESIAN_POINT ( 'NONE',  ( 17.00271606754840903, 67.00000000000000000, -28.39578712880048528 ) ) ;
#10480=CARTESIAN_POINT ( 'NONE',  ( -27.16883889988624290, 36.92500000273117422, -19.73931689729374028 ) ) ;
#10485=CARTESIAN_POINT ( 'NONE',  ( 32.50000000000000711, 55.40000000546238113, 10.55989012756945122 ) ) ;
#10492=CARTESIAN_POINT ( 'NONE',  ( 10.37757302488624767, 31.97500000273119269, 31.93888565452638417 ) ) ;
#10496=CARTESIAN_POINT ( 'NONE',  ( -10.04305231718578462, 22.90000000546237047, 30.90933677959249337 ) ) ;
#10507=CARTESIAN_POINT ( 'NONE',  ( -10.37757302488624411, 62.72500000273119269, -31.93888565452638417 ) ) ;
#10513=CARTESIAN_POINT ( 'NONE',  ( 1.093617666956751375E-13, 66.00000000546238255, -32.50000000000000711 ) ) ;
#10518=EDGE_CURVE ( 'NONE', #19648, #1729, #21419, .T. ) ;
#10519=CARTESIAN_POINT ( 'NONE',  ( 6.486482029760649416E-15, 75.87500000273119838, 35.31076352940723240 ) ) ;
#10523=CARTESIAN_POINT ( 'NONE',  ( 10.37757302488624767, 55.72500000273118559, 31.93888565452638417 ) ) ;
#10524=CARTESIAN_POINT ( 'NONE',  ( 33.58253175000000823, 14.27500000273119340, 10.91162601494192863 ) ) ;
#10525=CARTESIAN_POINT ( 'NONE',  ( -33.58253175000000113, 3.475000002731185589, 10.91162601494193929 ) ) ;
#10529=CARTESIAN_POINT ( 'NONE',  ( 26.29305231718579350, 71.30000000546236549, 19.10302069950537529 ) ) ;
#10530=CARTESIAN_POINT ( 'NONE',  ( 16.81447360525979917, 52.00000000000001421, -28.18961368868568229 ) ) ;
#10535=ORIENTED_EDGE ( 'NONE', *, *, #21696, .F. ) ;
#10536=CARTESIAN_POINT ( 'NONE',  ( -33.58253175000000113, 55.27500000273120406, -10.91162601494193218 ) ) ;
#10541=CARTESIAN_POINT ( 'NONE',  ( 33.58253175000000113, 22.22500000273117493, -10.91162601494193751 ) ) ;
#10549=CARTESIAN_POINT ( 'NONE',  ( 5.779280353836490358E-15, 59.00000000546238255, 32.49999999999999289 ) ) ;
#10552=CARTESIAN_POINT ( 'NONE',  ( 5.147494310547481966, 65.94874572391553613, -32.49999999999998579 ) ) ;
#10554=CARTESIAN_POINT ( 'NONE',  ( 32.50000000000000711, 16.89999999999998437, 10.55989012756945122 ) ) ;
#10556=EDGE_CURVE ( 'NONE', #32671, #29627, #20991, .T. ) ;
#10562=CARTESIAN_POINT ( 'NONE',  ( -33.58253175000000113, 71.22500000273117848, 10.91162601494193929 ) ) ;
#10563=CARTESIAN_POINT ( 'NONE',  ( -20.75514604977248112, 39.67500000273118133, 28.56700777964554661 ) ) ;
#10570=CARTESIAN_POINT ( 'NONE',  ( 26.29305231718579350, 54.80000000000000426, 19.10302069950537529 ) ) ;
#10576=CARTESIAN_POINT ( 'NONE',  ( 33.58253175000000113, 74.47500000273116427, -10.91162601494193751 ) ) ;
#10580=VERTEX_POINT ( 'NONE', #15841 ) ;
#10581=CARTESIAN_POINT ( 'NONE',  ( 20.75514604977248467, 46.42500000273119554, -28.56700777964554305 ) ) ;
#10586=CARTESIAN_POINT ( 'NONE',  ( 32.50000000000000000, 1.500000005462381880, -3.980102097228898626E-15 ) ) ;
#10605=CARTESIAN_POINT ( 'NONE',  ( 20.75514604977249178, 56.07500000273117990, 28.56700777964553950 ) ) ;
#10611=CARTESIAN_POINT ( 'NONE',  ( -32.50000000000000000, 70.10000000000000853, 10.55989012756946366 ) ) ;
#10612=CARTESIAN_POINT ( 'NONE',  ( 33.58253175000000113, 14.22500000273119625, -10.91162601494193751 ) ) ;
#10617=CARTESIAN_POINT ( 'NONE',  ( -20.08610463437157989, 38.20000000546236407, -27.64615127144129758 ) ) ;
#10624=CARTESIAN_POINT ( 'NONE',  ( 20.75514604977248467, 64.42500000273116711, -28.56700777964554305 ) ) ;
#10628=CARTESIAN_POINT ( 'NONE',  ( -33.58253175000000113, 3.125000002731193049, 0.000000000000000000 ) ) ;
#10636=CARTESIAN_POINT ( 'NONE',  ( -10.04305231718578462, 20.40000000000001634, 30.90933677959249337 ) ) ;
#10648=CARTESIAN_POINT ( 'NONE',  ( 1.683996601885203503, 67.00000000000000000, -33.30202823065786788 ) ) ;
#10650=CARTESIAN_POINT ( 'NONE',  ( -2.162160676586881955E-15, 32.62500000273119838, -35.31076352940723240 ) ) ;
#10651=CARTESIAN_POINT ( 'NONE',  ( -20.08610463437156923, 64.80000000546237970, 27.64615127144130113 ) ) ;
#10655=CARTESIAN_POINT ( 'NONE',  ( -20.08610463437156923, 52.80000000546237260, 27.64615127144130113 ) ) ;
#10657=PRESENTATION_STYLE_ASSIGNMENT (( #10323 ) ) ;
#10662=CARTESIAN_POINT ( 'NONE',  ( 6.486482029760649416E-15, 29.87500000273119838, 35.31076352940723240 ) ) ;
#10666=CARTESIAN_POINT ( 'NONE',  ( -32.50000000000000000, 14.40000000546236691, -10.55989012756945478 ) ) ;
#10675=CARTESIAN_POINT ( 'NONE',  ( 20.75514604977248467, 60.42500000273118133, -28.56700777964554305 ) ) ;
#10684=CARTESIAN_POINT ( 'NONE',  ( -33.58253175000000113, 77.37500000273118417, 0.000000000000000000 ) ) ;
#10689=( BOUNDED_SURFACE ( )  B_SPLINE_SURFACE ( 1, 2, ( 
 ( #25509, #20196, #17617, #22934, #25333, #1297, #14701, #24990, #19681, #28078, #17452, #30468, #1811, #25159, #27912, #7307, #20366, #30127, #30814, #27568, #4395, #4567, #1473, #27401, #14869, #1989, #17109, #11779, #9889, #15567, #4909, #7996, #20544, #7824, #28584, #18313, #26360, #5254, #5424, #2335, #2158, #10404, #30989, #7654, #23453, #23793, #2849, #15215, #15904, #10576, #21054, #13320, #15736, #25678, #31162, #15389, #10064, #13146, #31332, #2511, #26191, #26020, #33915, #31667, #10745, #12632, #21224, #17969, #10241, #7489, #28419, #28759, #2686, #23619, #88, #31504, #20883, #25845, #33745, #4734, #12979, #23280, #18481, #28925, #18141, #12808, #259, #20721, #17792, #23102, #5081, #28251, #33566, #3519, #3356, #593, #6258, #31832, #767, #29753, #13826, #1089, #13991, #3194, #24452, #18815, #27024, #16075, #16241, #24295, #11408, #8663, #5593, #928, #21724, #16737, #29258, #24127, #21884, #32334, #431, #11248, #11571, #16407, #8827, #18651, #13494, #6087, #26697, #29089, #19147, #10915, #26530, #26861, #3024, #29585, #3685, #11084, #32170, #23961, #27195, #18982, #19311, #13663, #21387, #21556, #31999, #8495, #5762, #16569, #14159, #29427, #24615, #8326, #22052, #5930, #8161, #27528, #29927, #4017, #17069, #14491, #9160, #33175, #30086, #32498, #24949, #32830, #27364, #8997, #6592, #30255, #19644, #22726, #1258, #22545, #9320, #32994, #7099, #19983, #20159, #1431, #16902, #25121, #11738, #22381, #4189, #4529, #17582, #6430, #30603, #25299, #1768, #28043, #30430, #3849, #11909, #19807, #24779, #27874, #12076, #17239, #6929, #6759, #14661, #12426, #25473, #14324, #1951, #32665, #27699, #22218, #1599, #9502, #17412, #4357, #14833, #12249, #9677, #15004, #19478, #9851, #7618, #28384, #31291, #28719, #2299, #30952, #18098, #25644, #13109, #17754, #23067, #31125, #31464, #18272, #28545, #15354, #21013, #12597, #15527, #10536, #5043, #15864, #5215, #17934, #15698, #33527, #7785, #30778, #7449, #25980, #26152, #23414, #20328, #2646, #2473, #7956, #10030, #4873, #23583, #48, #15179, #12940, #26320, #33875, #18443, #33354, #28212, #20846, #25808, #7270, #10368, #2122, #4699, #28886, #20506, #12771, #23245, #5386, #33706, #2809, #22896, #10205, #20685, #31960, #16034, #3478, #8124, #13452, #21511, #21846, #8623, #8455, #5725, #11370, #2984, #5889, #889, #18944, #6214, #19105, #8283, #29544, #23920, #32127, #21184, #21351, #29389, #16526, #13783, #10704, #6045, #26821, #32291, #391, #29219, #26979, #13949, #5553, #16367, #16694, #3317, #24412, #23751, #18612, #11208, #31793, #217, #24252, #26489, #31626, #722, #29050, #21681, #8785, #16203, #19268, #10876, #29710, #24089, #27151, #18775, #26657, #3153, #13624, #557, #11045, #13276, #1216, #3644, #9121, #3978, #32456, #14119, #11696, #1394, #24740, #27830, #6386, #27658, #14451, #4147, #12207, #25076, #25252, #22180, #22010, #30217, #16863, #27488, #9283, #9633, #22678, #1048, #1727, #30385, #6887, #33129, #1557, #11528, #17029, #32625, #29885, #32954, #17200, #22343, #12033, #11867, #19767, #17539, #30560, #8957, #7056, #3812, #30050, #27324, #14283, #14620, #22503, #9456, #19938, #17367, #6718, #19603, #32790, #6554, #20116, #24908, #4313, #24576, #14788, #19437, #23371, #23027, #10329, #4658, #12896, #1906, #2081, #10156, #31249, #28501, #25428, #33832, #7576, #15656, #15138, #9984, #20805, #7741, #20286, #20638, #20969, #2252, #18230, #4486, #33310, #25935, #12556, #14962, #4998, #30733, #12383, #12726, #22852, #15481, #23541, #20458, #23196, #9809, #13065, #4827, #28676, #33484, #7226, #30909, #7403, #17889, #25602, #5172, #28342, #27999, #15307, #25766, #17712, #28170, #33658, #31081, #18056, #26106, #2428, #2604, #2, #10492, #31420, #7913, #6477, #2938, #2767, #11454, #31582, #8242, #24498, #24825, #27407, #15823, #16949, #11617, #22099, #3897, #16780, #26277, #31751, #5510, #10662, #14204, #32378, #3563, #27240, #16160, #971, #32707, #11785, #13232, #22265, #18569, #10831, #8082, #29010, #29802, #19358, #8874, #3733, #6304, #21928, #15991, #347, #5342, #14036, #23877, #24660, #1132, #18735, #26447, #32544, #21141, #9043, #23706, #13409, #26614, #14368, #19522, #21310, #172, #29970, #29177, #1304, #18397, #5682, #28843, #9548, #24996, #17623, #27574, #22422, #33044, #25516, #33220, #20028, #4233, #1995, #11953, #6973, #4573, #30474, #33396, #9719, #6803, #20202, #32871, #22767, #6636, #19850, #17458, #30645, #14875, #30133, #7142, #27918, #15051, #9368, #27743, #28084, #12470, #1479, #4401, #9895, #25340, #22940, #19687, #4063, #1817, #30304, #17116, #12295, #14535, #9202, #20372, #1643, #17282, #14707, #25165, #12119, #22591, #24936, #16726, #6582, #917, #3345, #11396, #24440, #21873, #16557, #17057, #3507, #5918, #32323, #6246, #751, #16395, #13977, #3674, #27010, #30076, #8650, #29916, #27181, #6418, #14480, #27353, #27519, #8814, #24282, #32484, #19135, #29741, #11558, #11899, #1421, #13815, #4006, #32654, #9149, #22371, #3838, #11235, #19297, #14148, #32157, #1246, #19467, #24604, #14313, #1078, #22040, #19795, #32818, #21711, #9310, #6073, #8986, #29572, #16890, #24768, #11725, #22207, #19631, #26848, #1936, #27863, #22884, #9666, #25633, #25461, #4516, #6917, #15167, #33514, #2112, #20147, #10019, #12585, #14991, #14652, #12414, #25285, #30941, #1588, #2285, #32985, #12064, #1757, #9489, #33341, #17922, #9838, #30591, #4861, #4688, #12237, #4345, #12760, #20316, #23055, #30765, #28029, #7255, #22713, #7436, #25112, #14820, #33163, #23232, #7087, #33692, #17742, #17571, #25796, #28202, #19972, #20490, #30418, #17399, #22535, #28373, #15341, #10191, #30243, #6748, #17228, #27688, #4178, #15516, #18764, #18599, #25967, #21002, #2798, #204, #28876, #29208, #13265, #29039, #23571, #543, #26646, #5714, #5542, #31451, #26138, #10692, #23908, #26309, #23404, #3140, #36, #16192, #20836, #379, #16023, #2461, #13613, #7944, #8272, #24078, #23740, #33865, #26478, #10525, #15689, #2971, #18432, #21173, #12927, #13441, #2635, #10865, #10358, #7774, #5372, #31281, #13098, #7607, #18087, #20674, #31113, #31615, #28535, #31780, #5030 ),
 ( #15853, #18261, #28707, #8112, #21339, #5205, #19064, #19395, #22138, #16654, #27618, #19729, #11827, #32582, #24535, #19229, #3771, #16987, #29843, #16482, #30174, #27109, #22303, #13908, #27445, #11657, #29503, #32749, #1006, #1346, #6677, #16822, #26938, #9081, #3602, #8745, #19562, #14076, #6344, #8580, #30010, #29666, #6516, #6008, #847, #11489, #3438, #6172, #681, #11167, #13739, #9242, #27278, #17161, #24865, #24208, #3937, #14412, #21638, #24374, #32084, #11326, #21803, #32252, #14242, #21968, #32416, #8912, #24699, #1176, #22981, #7356, #9938, #17497, #17843, #33440, #22809, #22461, #12339, #33089, #4784, #9411, #10114, #6846, #19895, #9591, #17324, #30688, #25725, #20246, #27959, #12682, #12514, #20073, #12163, #20593, #17666, #20413, #28127, #1862, #33268, #30516, #15263, #32912, #1687, #22637, #31039, #14917, #7534, #4615, #7014, #33614, #15091, #27787, #9761, #25209, #28297, #4273, #25559, #25385, #2039, #23149, #30864, #2204, #4441, #30345, #7185, #14747, #18018, #4104, #14577, #25038, #1518, #11993, #21271, #31714, #13541, #26407, #25889, #7868, #15615, #20766, #23840, #8041, #13192, #2899, #26239, #10624, #8371, #21433, #23330, #31875, #28630, #20930, #7701, #18189, #5469, #16122, #28464, #31378, #26575, #131, #26067, #10452, #15437, #23669, #33958, #13368, #305, #18360, #2560, #21101, #31210, #18696, #33794, #5129, #2728, #3071, #10793, #31545, #28804, #24004, #13027, #18527, #475, #28973, #4957, #8206, #23501, #29136, #5301, #5638, #2385, #15783, #15951, #10958, #12855, #10288, #24659, #32377, #6476, #29468, #811, #3732, #11616, #11129, #970, #11784, #27070, #22098, #29305, #24169, #16779, #26902, #5806, #29801, #21600, #16285, #3562, #13704, #6303, #14367, #11292, #14035, #640, #3896, #29628, #19521, #13871, #26743, #24338, #3401, #21771, #5973, #29969, #16450, #18858, #32215, #19190, #32043, #3236, #8707, #32543, #24824, #27239, #8543, #6131, #16615, #19028, #14203, #8873, #24497, #1131, #11452, #21927, #32706, #22264, #19357, #9042, #16948, #27406, #1303, #32870, #20201, #30820, #9201, #12118, #7312, #14874, #6802, #25164, #30132, #27917, #14706, #17622, #15050, #22590, #17281, #4400, #11952, #33395, #4062, #9367, #17457, #17797, #4572, #25339, #1642, #28256, #19849, #1816, #4740, #12294, #2163, #25515, #4232, #1994, #30302, #28083, #17115, #27742, #22766, #12469, #9718, #6635, #22939, #33219, #15220, #33043, #9546, #9894, #20371, #1478, #30644, #12637, #7141, #25683, #19686, #14534, #23107, #20027, #27573, #24995, #22421, #30473, #6972, #28425, #10581, #29094, #15572, #18318, #4914, #18656, #10410, #264, #28589, #30996, #5087, #18146, #26026, #10246, #10751, #31168, #33571, #2518, #33920, #15394, #10069, #7659, #31337, #20727, #23798, #2340, #23626, #20888, #93, #8166, #21059, #21229, #12985, #17975, #26196, #12813, #23458, #5260, #5598, #16081, #7494, #31672, #26365, #26535, #7829, #2855, #20549, #25850, #31509, #28764, #23285, #8002, #33752, #15742, #2691, #13151, #18487, #3029, #28930, #5429, #15910, #13501, #13325, #24620, #18988, #21392, #29432, #8500, #5935, #598, #1094, #21560, #23966, #16414, #24300, #18820, #436, #32004, #21730, #11090, #14164, #26703, #13997, #772, #24458, #32502, #11413, #11577, #26866, #8331, #16574, #3200, #13831, #29591, #29932, #9002, #31837, #22058, #16742, #27200, #19483, #21889, #29264, #3361, #11253, #16247, #19316, #3524, #8669, #32339, #32175, #6092, #3855, #16907, #5767, #27369, #24132, #19152, #13668, #27029, #934, #6436, #10920, #8833, #29758, #6264, #3691, #30262, #1264, #33000, #19812, #22731, #20165, #27705, #22386, #9507, #17074, #4535, #9165, #14497, #22549, #22901, #9682, #19988, #6765, #12432, #4022, #6935, #1958, #30435, #7276, #30608, #9326, #7104, #24954, #33180, #22223, #32835, #17418, #17587, #14838, #11743, #28048, #27879, #33360, #1436, #17244, #15009, #25479, #6598, #4363, #9856, #20333, #30783, #4194, #17759, #28217, #25304, #32670, #1774, #14666, #14329, #19649, #24785, #27534, #30091, #25126, #11915, #12254, #1604, #12081, #18103, #13281, #13114, #33711, #12776, #10709, #18279, #23588, #28725, #2478, #12945, #31131, #5391, #23072, #2304, #23250, #21189, #15532, #31631, #5220, #7623, #221, #15703, #28389, #10209, #4878, #25814, #33533, #28551, #10036, #25985, #15869, #20511, #20690, #26326, #5049, #30957, #2814, #2652, #7455, #23418, #20851, #21018, #23756, #17939, #10373, #53, #33880, #18617, #8129, #4704, #10541, #31297, #7789, #26157, #7961, #31470, #15359, #15185, #18448, #25649, #28891, #2127, #12603, #10881, #14124, #5894, #16700, #22015, #32133, #31798, #24417, #8460, #24094, #13954, #18949, #11213, #23927, #894, #11052, #11375, #396, #16208, #29394, #21356, #21517, #16039, #26494, #29055, #24581, #727, #27156, #6219, #3648, #32296, #3483, #1052, #29224, #8790, #19274, #8290, #11532, #21686, #16373, #21851, #24257, #3322, #5730, #18780, #26662, #562, #3159, #8628, #32460, #19111, #26826, #8960, #29715, #31966, #13630, #5560, #29550, #2989, #6050, #13789, #16533, #26984, #13458, #4279, #17503, #27965, #2391, #30694, #12860, #33446, #12346, #15443, #30870, #9598, #14924, #20080, #7021, #14753, #33274, #25215, #7191, #31046, #1693, #4447, #7539, #20252, #12169, #18024, #17850, #22643, #17673, #2045, #2210, #25565, #30522, #12520, #25391, #1868, #6853, #4621, #22815, #28303, #25731, #9768, #28134, #15100, #33095, #10120, #22988, #9945, #20421, #28470, #15270, #7364, #4790, #4963, #12689, #23157, #25897, #33621, #23337, #20600, #33799, #19441, #30351, #17331, #27794, #18364, #26411, #13545, #10797, #7708, #16126, #23844, #31880, #20936, #26244, #29140, #3076, #2566, #2904, #3240, #18531, #24008, #20771, #15620, #8210, #28809, #31215, #21275, #13034, #18194, #28977, #5134, #31718, #5811, #2733, #5475, #26072, #29309, #21105, #10962, #5305, #28637, #15788, #13196, #23673, #31384, #21437, #7875, #5643, #309, #8045, #15955, #137, #8376, #23506, #10628, #31549, #26747, #13373, #13708, #18701, #26580, #16289, #479, #33964, #18862, #10458, #24174, #10294, #14040, #19033, #21932, #11790, #5977, #32221, #22269 ) ),
 .UNSPECIFIED., .F., .F., .T. ) 
 B_SPLINE_SURFACE_WITH_KNOTS ( ( 2, 2 ),
 ( 3, 2, 2, 2, 2, 2, 2, 2, 2, 2, 2, 2, 2, 2, 2, 2, 2, 2, 2, 2, 2, 2, 2, 2, 2, 2, 2, 2, 2, 2, 2, 2, 2, 2, 2, 2, 2, 2, 2, 2, 2, 2, 2, 2, 2, 2, 2, 2, 2, 2, 2, 2, 2, 2, 2, 2, 2, 2, 2, 2, 2, 2, 2, 2, 2, 2, 2, 2, 2, 2, 2, 2, 2, 2, 2, 2, 2, 2, 2, 2, 2, 2, 2, 2, 2, 2, 2, 2, 2, 2, 2, 2, 2, 2, 2, 2, 2, 2, 2, 2, 2, 2, 2, 2, 2, 2, 2, 2, 2, 2, 2, 2, 2, 2, 2, 2, 2, 2, 2, 2, 2, 2, 2, 2, 2, 2, 2, 2, 2, 2, 2, 2, 2, 2, 2, 2, 2, 2, 2, 2, 2, 2, 2, 2, 2, 2, 2, 2, 2, 2, 2, 2, 2, 2, 2, 2, 2, 2, 2, 2, 2, 2, 2, 2, 2, 2, 2, 2, 2, 2, 2, 2, 2, 2, 2, 2, 2, 2, 2, 2, 2, 2, 2, 2, 2, 2, 2, 2, 2, 2, 2, 2, 2, 2, 2, 2, 2, 2, 2, 2, 2, 2, 2, 2, 2, 2, 2, 2, 2, 2, 2, 2, 2, 2, 2, 2, 2, 2, 2, 2, 2, 2, 2, 2, 2, 2, 2, 2, 2, 2, 2, 2, 2, 2, 2, 2, 2, 2, 2, 2, 2, 2, 2, 2, 2, 2, 2, 2, 2, 2, 2, 2, 2, 2, 2, 2, 2, 2, 2, 2, 2, 2, 2, 2, 2, 2, 2, 2, 2, 2, 2, 2, 2, 2, 2, 2, 2, 2, 2, 2, 2, 2, 2, 2, 2, 2, 2, 2, 2, 2, 2, 2, 2, 2, 2, 2, 2, 2, 2, 2, 2, 2, 2, 2, 2, 2, 2, 2, 2, 2, 2, 2, 2, 2, 2, 2, 2, 2, 2, 2, 2, 2, 2, 2, 2, 2, 2, 2, 2, 2, 2, 2, 2, 2, 2, 2, 2, 2, 2, 2, 2, 2, 2, 2, 2, 2, 2, 2, 2, 2, 2, 2, 2, 2, 2, 2, 2, 2, 2, 2, 2, 2, 2, 2, 2, 2, 2, 2, 2, 2, 2, 2, 2, 2, 2, 2, 2, 2, 2, 2, 2, 2, 2, 2, 2, 2, 2, 2, 2, 2, 3 ),
 ( 0.000000000000000000, 1.000000000000000000 ),
 ( 0.000000000000000000, 0.002564102564102564100, 0.005128205128205128201, 0.007692307692307692735, 0.01025641025641025640, 0.01282051282051282007, 0.01538461538461538547, 0.01794871794871794740, 0.02051282051282051280, 0.02307692307692307820, 0.02564102564102564014, 0.02820512820512820554, 0.03076923076923077094, 0.03333333333333333287, 0.03589743589743589480, 0.03846153846153846367, 0.04102564102564102561, 0.04358974358974358754, 0.04615384615384615641, 0.04871794871794871834, 0.05128205128205128027, 0.05384615384615384914, 0.05641025641025641107, 0.05897435897435897301, 0.06153846153846154188, 0.06410256410256409687, 0.06666666666666666574, 0.06923076923076923461, 0.07179487179487178961, 0.07435897435897435848, 0.07692307692307692735, 0.07948717948717948234, 0.08205128205128205121, 0.08461538461538462008, 0.08717948717948717507, 0.08974358974358974395, 0.09230769230769231282, 0.09487179487179486781, 0.09743589743589743668, 0.1000000000000000056, 0.1025641025641025605, 0.1051282051282051294, 0.1076923076923076983, 0.1102564102564102533, 0.1128205128205128221, 0.1153846153846153910, 0.1179487179487179460, 0.1205128205128205149, 0.1230769230769230838, 0.1256410256410256387, 0.1282051282051281937, 0.1307692307692307765, 0.1333333333333333315, 0.1358974358974358865, 0.1384615384615384692, 0.1410256410256410242, 0.1435897435897435792, 0.1461538461538461620, 0.1487179487179487170, 0.1512820512820512719, 0.1538461538461538547, 0.1564102564102564097, 0.1589743589743589647, 0.1615384615384615474, 0.1641025641025641024, 0.1666666666666666574, 0.1692307692307692402, 0.1717948717948717952, 0.1743589743589743501, 0.1769230769230769329, 0.1794871794871794879, 0.1820512820512820429, 0.1846153846153846256, 0.1871794871794871806, 0.1897435897435897356, 0.1923076923076923184, 0.1948717948717948734, 0.1974358974358974284, 0.2000000000000000111, 0.2025641025641025661, 0.2051282051282051211, 0.2076923076923077038, 0.2102564102564102588, 0.2128205128205128138, 0.2153846153846153966, 0.2179487179487179516, 0.2205128205128205066, 0.2230769230769230893, 0.2256410256410256443, 0.2282051282051281993, 0.2307692307692307820, 0.2333333333333333370, 0.2358974358974358920, 0.2384615384615384748, 0.2410256410256410298, 0.2435897435897435848, 0.2461538461538461675, 0.2487179487179487225, 0.2512820512820512775, 0.2538461538461538325, 0.2564102564102563875, 0.2589743589743589980, 0.2615384615384615530, 0.2641025641025641080, 0.2666666666666666630, 0.2692307692307692180, 0.2717948717948717730, 0.2743589743589743835, 0.2769230769230769384, 0.2794871794871794934, 0.2820512820512820484, 0.2846153846153846034, 0.2871794871794871584, 0.2897435897435897689, 0.2923076923076923239, 0.2948717948717948789, 0.2974358974358974339, 0.2999999999999999889, 0.3025641025641025439, 0.3051282051282051544, 0.3076923076923077094, 0.3102564102564102644, 0.3128205128205128194, 0.3153846153846153744, 0.3179487179487179294, 0.3205128205128205399, 0.3230769230769230949, 0.3256410256410256499, 0.3282051282051282048, 0.3307692307692307598, 0.3333333333333333148, 0.3358974358974358698, 0.3384615384615384803, 0.3410256410256410353, 0.3435897435897435903, 0.3461538461538461453, 0.3487179487179487003, 0.3512820512820512553, 0.3538461538461538658, 0.3564102564102564208, 0.3589743589743589758, 0.3615384615384615308, 0.3641025641025640858, 0.3666666666666666408, 0.3692307692307692513, 0.3717948717948718063, 0.3743589743589743613, 0.3769230769230769162, 0.3794871794871794712, 0.3820512820512820262, 0.3846153846153846367, 0.3871794871794871917, 0.3897435897435897467, 0.3923076923076923017, 0.3948717948717948567, 0.3974358974358974117, 0.4000000000000000222, 0.4025641025641025772, 0.4051282051282051322, 0.4076923076923076872, 0.4102564102564102422, 0.4128205128205127972, 0.4153846153846154077, 0.4179487179487179627, 0.4205128205128205177, 0.4230769230769230727, 0.4256410256410256276, 0.4282051282051281826, 0.4307692307692307931, 0.4333333333333333481, 0.4358974358974359031, 0.4384615384615384581, 0.4410256410256410131, 0.4435897435897435681, 0.4461538461538461786, 0.4487179487179487336, 0.4512820512820512886, 0.4538461538461538436, 0.4564102564102563986, 0.4589743589743589536, 0.4615384615384615641, 0.4641025641025641191, 0.4666666666666666741, 0.4692307692307692291, 0.4717948717948717841, 0.4743589743589743390, 0.4769230769230769496, 0.4794871794871795045, 0.4820512820512820595, 0.4846153846153846145, 0.4871794871794871695, 0.4897435897435897245, 0.4923076923076923350, 0.4948717948717948900, 0.4974358974358974450, 0.5000000000000000000, 0.5025641025641025550, 0.5051282051282051100, 0.5076923076923076650, 0.5102564102564102200, 0.5128205128205127750, 0.5153846153846153300, 0.5179487179487179960, 0.5205128205128205510, 0.5230769230769231060, 0.5256410256410256610, 0.5282051282051282159, 0.5307692307692307709, 0.5333333333333333259, 0.5358974358974358809, 0.5384615384615384359, 0.5410256410256409909, 0.5435897435897435459, 0.5461538461538461009, 0.5487179487179487669, 0.5512820512820513219, 0.5538461538461538769, 0.5564102564102564319, 0.5589743589743589869, 0.5615384615384615419, 0.5641025641025640969, 0.5666666666666666519, 0.5692307692307692069, 0.5717948717948717618, 0.5743589743589743168, 0.5769230769230768718, 0.5794871794871795379, 0.5820512820512820928, 0.5846153846153846478, 0.5871794871794872028, 0.5897435897435897578, 0.5923076923076923128, 0.5948717948717948678, 0.5974358974358974228, 0.5999999999999999778, 0.6025641025641025328, 0.6051282051282050878, 0.6076923076923076428, 0.6102564102564103088, 0.6128205128205128638, 0.6153846153846154188, 0.6179487179487179738, 0.6205128205128205288, 0.6230769230769230838, 0.6256410256410256387, 0.6282051282051281937, 0.6307692307692307487, 0.6333333333333333037, 0.6358974358974358587, 0.6384615384615384137, 0.6410256410256410797, 0.6435897435897436347, 0.6461538461538461897, 0.6487179487179487447, 0.6512820512820512997, 0.6538461538461538547, 0.6564102564102564097, 0.6589743589743589647, 0.6615384615384615197, 0.6641025641025640747, 0.6666666666666666297, 0.6692307692307691847, 0.6717948717948717396, 0.6743589743589744057, 0.6769230769230769607, 0.6794871794871795156, 0.6820512820512820706, 0.6846153846153846256, 0.6871794871794871806, 0.6897435897435897356, 0.6923076923076922906, 0.6948717948717948456, 0.6974358974358974006, 0.6999999999999999556, 0.7025641025641025106, 0.7051282051282051766, 0.7076923076923077316, 0.7102564102564102866, 0.7128205128205128416, 0.7153846153846153966, 0.7179487179487179516, 0.7205128205128205066, 0.7230769230769230616, 0.7256410256410256165, 0.7282051282051281715, 0.7307692307692307265, 0.7333333333333332815, 0.7358974358974359475, 0.7384615384615385025, 0.7410256410256410575, 0.7435897435897436125, 0.7461538461538461675, 0.7487179487179487225, 0.7512820512820512775, 0.7538461538461538325, 0.7564102564102563875, 0.7589743589743589425, 0.7615384615384614975, 0.7641025641025640525, 0.7666666666666667185, 0.7692307692307692735, 0.7717948717948718285, 0.7743589743589743835, 0.7769230769230769384, 0.7794871794871794934, 0.7820512820512820484, 0.7846153846153846034, 0.7871794871794871584, 0.7897435897435897134, 0.7923076923076922684, 0.7948717948717948234, 0.7974358974358974894, 0.8000000000000000444, 0.8025641025641025994, 0.8051282051282051544, 0.8076923076923077094, 0.8102564102564102644, 0.8128205128205128194, 0.8153846153846153744, 0.8179487179487179294, 0.8205128205128204844, 0.8230769230769230393, 0.8256410256410255943, 0.8282051282051282604, 0.8307692307692308153, 0.8333333333333333703, 0.8358974358974359253, 0.8384615384615384803, 0.8410256410256410353, 0.8435897435897435903, 0.8461538461538461453, 0.8487179487179487003, 0.8512820512820512553, 0.8538461538461538103, 0.8564102564102563653, 0.8589743589743589203, 0.8615384615384615863, 0.8641025641025641413, 0.8666666666666666963, 0.8692307692307692513, 0.8717948717948718063, 0.8743589743589743613, 0.8769230769230769162, 0.8794871794871794712, 0.8820512820512820262, 0.8846153846153845812, 0.8871794871794871362, 0.8897435897435896912, 0.8923076923076923572, 0.8948717948717949122, 0.8974358974358974672, 0.9000000000000000222, 0.9025641025641025772, 0.9051282051282051322, 0.9076923076923076872, 0.9102564102564102422, 0.9128205128205127972, 0.9153846153846153522, 0.9179487179487179072, 0.9205128205128204621, 0.9230769230769231282, 0.9256410256410256832, 0.9282051282051282382, 0.9307692307692307931, 0.9333333333333333481, 0.9358974358974359031, 0.9384615384615384581, 0.9410256410256410131, 0.9435897435897435681, 0.9461538461538461231, 0.9487179487179486781, 0.9512820512820512331, 0.9538461538461538991, 0.9564102564102564541, 0.9589743589743590091, 0.9615384615384615641, 0.9641025641025641191, 0.9666666666666666741, 0.9692307692307692291, 0.9717948717948717841, 0.9743589743589743390, 0.9769230769230768940, 0.9794871794871794490, 0.9820512820512820040, 0.9846153846153846700, 0.9871794871794872250, 0.9897435897435897800, 0.9923076923076923350, 0.9948717948717948900, 0.9974358974358974450, 1.000000000000000000 ),
 .UNSPECIFIED. ) 
 GEOMETRIC_REPRESENTATION_ITEM ( )  RATIONAL_B_SPLINE_SURFACE ( (
 ( 1.000000000000000000, 0.9510565162951535312, 1.000000000000000000, 0.9510565162951535312, 1.000000000000000000, 0.9510565162951535312, 1.000000000000000000, 0.9510565162951535312, 1.000000000000000000, 0.9510565162951535312, 1.000000000000000000, 0.9510565162951535312, 1.000000000000000000, 0.9510565162951535312, 1.000000000000000000, 0.9510565162951535312, 1.000000000000000000, 0.9510565162951535312, 1.000000000000000000, 0.9510565162951535312, 1.000000000000000000, 0.9510565162951535312, 1.000000000000000000, 0.9510565162951535312, 1.000000000000000000, 0.9510565162951535312, 1.000000000000000000, 0.9510565162951535312, 1.000000000000000000, 0.9510565162951535312, 1.000000000000000000, 0.9510565162951535312, 1.000000000000000000, 0.9510565162951535312, 1.000000000000000000, 0.9510565162951535312, 1.000000000000000000, 0.9510565162951535312, 1.000000000000000000, 0.9510565162951535312, 1.000000000000000000, 0.9510565162951535312, 1.000000000000000000, 0.9510565162951535312, 1.000000000000000000, 0.9510565162951535312, 1.000000000000000000, 0.9510565162951535312, 1.000000000000000000, 0.9510565162951535312, 1.000000000000000000, 0.9510565162951535312, 1.000000000000000000, 0.9510565162951535312, 1.000000000000000000, 0.9510565162951535312, 1.000000000000000000, 0.9510565162951535312, 1.000000000000000000, 0.9510565162951535312, 1.000000000000000000, 0.9510565162951535312, 1.000000000000000000, 0.9510565162951535312, 1.000000000000000000, 0.9510565162951535312, 1.000000000000000000, 0.9510565162951535312, 1.000000000000000000, 0.9510565162951535312, 1.000000000000000000, 0.9510565162951535312, 1.000000000000000000, 0.9510565162951535312, 1.000000000000000000, 0.9510565162951535312, 1.000000000000000000, 0.9510565162951535312, 1.000000000000000000, 0.9510565162951535312, 1.000000000000000000, 0.9510565162951535312, 1.000000000000000000, 0.9510565162951535312, 1.000000000000000000, 0.9510565162951535312, 1.000000000000000000, 0.9510565162951535312, 1.000000000000000000, 0.9510565162951535312, 1.000000000000000000, 0.9510565162951535312, 1.000000000000000000, 0.9510565162951535312, 1.000000000000000000, 0.9510565162951535312, 1.000000000000000000, 0.9510565162951535312, 1.000000000000000000, 0.9510565162951535312, 1.000000000000000000, 0.9510565162951535312, 1.000000000000000000, 0.9510565162951535312, 1.000000000000000000, 0.9510565162951535312, 1.000000000000000000, 0.9510565162951535312, 1.000000000000000000, 0.9510565162951535312, 1.000000000000000000, 0.9510565162951535312, 1.000000000000000000, 0.9510565162951535312, 1.000000000000000000, 0.9510565162951535312, 1.000000000000000000, 0.9510565162951535312, 1.000000000000000000, 0.9510565162951535312, 1.000000000000000000, 0.9510565162951535312, 1.000000000000000000, 0.9510565162951535312, 1.000000000000000000, 0.9510565162951535312, 1.000000000000000000, 0.9510565162951535312, 1.000000000000000000, 0.9510565162951535312, 1.000000000000000000, 0.9510565162951535312, 1.000000000000000000, 0.9510565162951535312, 1.000000000000000000, 0.9510565162951535312, 1.000000000000000000, 0.9510565162951535312, 1.000000000000000000, 0.9510565162951535312, 1.000000000000000000, 0.9510565162951535312, 1.000000000000000000, 0.9510565162951535312, 1.000000000000000000, 0.9510565162951535312, 1.000000000000000000, 0.9510565162951535312, 1.000000000000000000, 0.9510565162951535312, 1.000000000000000000, 0.9510565162951535312, 1.000000000000000000, 0.9510565162951535312, 1.000000000000000000, 0.9510565162951535312, 1.000000000000000000, 0.9510565162951535312, 1.000000000000000000, 0.9510565162951535312, 1.000000000000000000, 0.9510565162951535312, 1.000000000000000000, 0.9510565162951535312, 1.000000000000000000, 0.9510565162951535312, 1.000000000000000000, 0.9510565162951535312, 1.000000000000000000, 0.9510565162951535312, 1.000000000000000000, 0.9510565162951535312, 1.000000000000000000, 0.9510565162951535312, 1.000000000000000000, 0.9510565162951535312, 1.000000000000000000, 0.9510565162951535312, 1.000000000000000000, 0.9510565162951535312, 1.000000000000000000, 0.9510565162951535312, 1.000000000000000000, 0.9510565162951535312, 1.000000000000000000, 0.9510565162951535312, 1.000000000000000000, 0.9510565162951535312, 1.000000000000000000, 0.9510565162951535312, 1.000000000000000000, 0.9510565162951535312, 1.000000000000000000, 0.9510565162951535312, 1.000000000000000000, 0.9510565162951535312, 1.000000000000000000, 0.9510565162951535312, 1.000000000000000000, 0.9510565162951535312, 1.000000000000000000, 0.9510565162951535312, 1.000000000000000000, 0.9510565162951535312, 1.000000000000000000, 0.9510565162951535312, 1.000000000000000000, 0.9510565162951535312, 1.000000000000000000, 0.9510565162951535312, 1.000000000000000000, 0.9510565162951535312, 1.000000000000000000, 0.9510565162951535312, 1.000000000000000000, 0.9510565162951535312, 1.000000000000000000, 0.9510565162951535312, 1.000000000000000000, 0.9510565162951535312, 1.000000000000000000, 0.9510565162951535312, 1.000000000000000000, 0.9510565162951535312, 1.000000000000000000, 0.9510565162951535312, 1.000000000000000000, 0.9510565162951535312, 1.000000000000000000, 0.9510565162951535312, 1.000000000000000000, 0.9510565162951535312, 1.000000000000000000, 0.9510565162951535312, 1.000000000000000000, 0.9510565162951535312, 1.000000000000000000, 0.9510565162951535312, 1.000000000000000000, 0.9510565162951535312, 1.000000000000000000, 0.9510565162951535312, 1.000000000000000000, 0.9510565162951535312, 1.000000000000000000, 0.9510565162951535312, 1.000000000000000000, 0.9510565162951535312, 1.000000000000000000, 0.9510565162951535312, 1.000000000000000000, 0.9510565162951535312, 1.000000000000000000, 0.9510565162951535312, 1.000000000000000000, 0.9510565162951535312, 1.000000000000000000, 0.9510565162951535312, 1.000000000000000000, 0.9510565162951535312, 1.000000000000000000, 0.9510565162951535312, 1.000000000000000000, 0.9510565162951535312, 1.000000000000000000, 0.9510565162951535312, 1.000000000000000000, 0.9510565162951535312, 1.000000000000000000, 0.9510565162951535312, 1.000000000000000000, 0.9510565162951535312, 1.000000000000000000, 0.9510565162951535312, 1.000000000000000000, 0.9510565162951535312, 1.000000000000000000, 0.9510565162951535312, 1.000000000000000000, 0.9510565162951535312, 1.000000000000000000, 0.9510565162951535312, 1.000000000000000000, 0.9510565162951535312, 1.000000000000000000, 0.9510565162951535312, 1.000000000000000000, 0.9510565162951535312, 1.000000000000000000, 0.9510565162951535312, 1.000000000000000000, 0.9510565162951535312, 1.000000000000000000, 0.9510565162951535312, 1.000000000000000000, 0.9510565162951535312, 1.000000000000000000, 0.9510565162951535312, 1.000000000000000000, 0.9510565162951535312, 1.000000000000000000, 0.9510565162951535312, 1.000000000000000000, 0.9510565162951535312, 1.000000000000000000, 0.9510565162951535312, 1.000000000000000000, 0.9510565162951535312, 1.000000000000000000, 0.9510565162951535312, 1.000000000000000000, 0.9510565162951535312, 1.000000000000000000, 0.9510565162951535312, 1.000000000000000000, 0.9510565162951535312, 1.000000000000000000, 0.9510565162951535312, 1.000000000000000000, 0.9510565162951535312, 1.000000000000000000, 0.9510565162951535312, 1.000000000000000000, 0.9510565162951535312, 1.000000000000000000, 0.9510565162951535312, 1.000000000000000000, 0.9510565162951535312, 1.000000000000000000, 0.9510565162951535312, 1.000000000000000000, 0.9510565162951535312, 1.000000000000000000, 0.9510565162951535312, 1.000000000000000000, 0.9510565162951535312, 1.000000000000000000, 0.9510565162951535312, 1.000000000000000000, 0.9510565162951535312, 1.000000000000000000, 0.9510565162951535312, 1.000000000000000000, 0.9510565162951535312, 1.000000000000000000, 0.9510565162951535312, 1.000000000000000000, 0.9510565162951535312, 1.000000000000000000, 0.9510565162951535312, 1.000000000000000000, 0.9510565162951535312, 1.000000000000000000, 0.9510565162951535312, 1.000000000000000000, 0.9510565162951535312, 1.000000000000000000, 0.9510565162951535312, 1.000000000000000000, 0.9510565162951535312, 1.000000000000000000, 0.9510565162951535312, 1.000000000000000000, 0.9510565162951535312, 1.000000000000000000, 0.9510565162951535312, 1.000000000000000000, 0.9510565162951535312, 1.000000000000000000, 0.9510565162951535312, 1.000000000000000000, 0.9510565162951535312, 1.000000000000000000, 0.9510565162951535312, 1.000000000000000000, 0.9510565162951535312, 1.000000000000000000, 0.9510565162951535312, 1.000000000000000000, 0.9510565162951535312, 1.000000000000000000, 0.9510565162951535312, 1.000000000000000000, 0.9510565162951535312, 1.000000000000000000, 0.9510565162951535312, 1.000000000000000000, 0.9510565162951535312, 1.000000000000000000, 0.9510565162951535312, 1.000000000000000000, 0.9510565162951535312, 1.000000000000000000, 0.9510565162951535312, 1.000000000000000000, 0.9510565162951535312, 1.000000000000000000, 0.9510565162951535312, 1.000000000000000000, 0.9510565162951535312, 1.000000000000000000, 0.9510565162951535312, 1.000000000000000000, 0.9510565162951535312, 1.000000000000000000, 0.9510565162951535312, 1.000000000000000000, 0.9510565162951535312, 1.000000000000000000, 0.9510565162951535312, 1.000000000000000000, 0.9510565162951535312, 1.000000000000000000, 0.9510565162951535312, 1.000000000000000000, 0.9510565162951535312, 1.000000000000000000, 0.9510565162951535312, 1.000000000000000000, 0.9510565162951535312, 1.000000000000000000, 0.9510565162951535312, 1.000000000000000000, 0.9510565162951535312, 1.000000000000000000, 0.9510565162951535312, 1.000000000000000000, 0.9510565162951535312, 1.000000000000000000, 0.9510565162951535312, 1.000000000000000000, 0.9510565162951535312, 1.000000000000000000, 0.9510565162951535312, 1.000000000000000000, 0.9510565162951535312, 1.000000000000000000, 0.9510565162951535312, 1.000000000000000000, 0.9510565162951535312, 1.000000000000000000, 0.9510565162951535312, 1.000000000000000000, 0.9510565162951535312, 1.000000000000000000, 0.9510565162951535312, 1.000000000000000000, 0.9510565162951535312, 1.000000000000000000, 0.9510565162951535312, 1.000000000000000000, 0.9510565162951535312, 1.000000000000000000, 0.9510565162951535312, 1.000000000000000000, 0.9510565162951535312, 1.000000000000000000, 0.9510565162951535312, 1.000000000000000000, 0.9510565162951535312, 1.000000000000000000, 0.9510565162951535312, 1.000000000000000000, 0.9510565162951535312, 1.000000000000000000, 0.9510565162951535312, 1.000000000000000000, 0.9510565162951535312, 1.000000000000000000, 0.9510565162951535312, 1.000000000000000000, 0.9510565162951535312, 1.000000000000000000, 0.9510565162951535312, 1.000000000000000000, 0.9510565162951535312, 1.000000000000000000, 0.9510565162951535312, 1.000000000000000000, 0.9510565162951535312, 1.000000000000000000, 0.9510565162951535312, 1.000000000000000000, 0.9510565162951535312, 1.000000000000000000, 0.9510565162951535312, 1.000000000000000000, 0.9510565162951535312, 1.000000000000000000, 0.9510565162951535312, 1.000000000000000000, 0.9510565162951535312, 1.000000000000000000, 0.9510565162951535312, 1.000000000000000000, 0.9510565162951535312, 1.000000000000000000, 0.9510565162951535312, 1.000000000000000000, 0.9510565162951535312, 1.000000000000000000, 0.9510565162951535312, 1.000000000000000000, 0.9510565162951535312, 1.000000000000000000, 0.9510565162951535312, 1.000000000000000000, 0.9510565162951535312, 1.000000000000000000, 0.9510565162951535312, 1.000000000000000000, 0.9510565162951535312, 1.000000000000000000, 0.9510565162951535312, 1.000000000000000000, 0.9510565162951535312, 1.000000000000000000, 0.9510565162951535312, 1.000000000000000000, 0.9510565162951535312, 1.000000000000000000, 0.9510565162951535312, 1.000000000000000000, 0.9510565162951535312, 1.000000000000000000, 0.9510565162951535312, 1.000000000000000000, 0.9510565162951535312, 1.000000000000000000, 0.9510565162951535312, 1.000000000000000000, 0.9510565162951535312, 1.000000000000000000, 0.9510565162951535312, 1.000000000000000000, 0.9510565162951535312, 1.000000000000000000, 0.9510565162951535312, 1.000000000000000000, 0.9510565162951535312, 1.000000000000000000, 0.9510565162951535312, 1.000000000000000000, 0.9510565162951535312, 1.000000000000000000, 0.9510565162951535312, 1.000000000000000000, 0.9510565162951535312, 1.000000000000000000, 0.9510565162951535312, 1.000000000000000000, 0.9510565162951535312, 1.000000000000000000, 0.9510565162951535312, 1.000000000000000000, 0.9510565162951535312, 1.000000000000000000, 0.9510565162951535312, 1.000000000000000000, 0.9510565162951535312, 1.000000000000000000, 0.9510565162951535312, 1.000000000000000000, 0.9510565162951535312, 1.000000000000000000, 0.9510565162951535312, 1.000000000000000000, 0.9510565162951535312, 1.000000000000000000, 0.9510565162951535312, 1.000000000000000000, 0.9510565162951535312, 1.000000000000000000, 0.9510565162951535312, 1.000000000000000000, 0.9510565162951535312, 1.000000000000000000, 0.9510565162951535312, 1.000000000000000000, 0.9510565162951535312, 1.000000000000000000, 0.9510565162951535312, 1.000000000000000000, 0.9510565162951535312, 1.000000000000000000, 0.9510565162951535312, 1.000000000000000000, 0.9510565162951535312, 1.000000000000000000, 0.9510565162951535312, 1.000000000000000000, 0.9510565162951535312, 1.000000000000000000, 0.9510565162951535312, 1.000000000000000000, 0.9510565162951535312, 1.000000000000000000, 0.9510565162951535312, 1.000000000000000000, 0.9510565162951535312, 1.000000000000000000, 0.9510565162951535312, 1.000000000000000000, 0.9510565162951535312, 1.000000000000000000, 0.9510565162951535312, 1.000000000000000000, 0.9510565162951535312, 1.000000000000000000, 0.9510565162951535312, 1.000000000000000000, 0.9510565162951535312, 1.000000000000000000, 0.9510565162951535312, 1.000000000000000000, 0.9510565162951535312, 1.000000000000000000, 0.9510565162951535312, 1.000000000000000000, 0.9510565162951535312, 1.000000000000000000, 0.9510565162951535312, 1.000000000000000000, 0.9510565162951535312, 1.000000000000000000, 0.9510565162951535312, 1.000000000000000000, 0.9510565162951535312, 1.000000000000000000, 0.9510565162951535312, 1.000000000000000000, 0.9510565162951535312, 1.000000000000000000, 0.9510565162951535312, 1.000000000000000000, 0.9510565162951535312, 1.000000000000000000, 0.9510565162951535312, 1.000000000000000000, 0.9510565162951535312, 1.000000000000000000, 0.9510565162951535312, 1.000000000000000000, 0.9510565162951535312, 1.000000000000000000, 0.9510565162951535312, 1.000000000000000000, 0.9510565162951535312, 1.000000000000000000, 0.9510565162951535312, 1.000000000000000000, 0.9510565162951535312, 1.000000000000000000, 0.9510565162951535312, 1.000000000000000000, 0.9510565162951535312, 1.000000000000000000, 0.9510565162951535312, 1.000000000000000000, 0.9510565162951535312, 1.000000000000000000, 0.9510565162951535312, 1.000000000000000000, 0.9510565162951535312, 1.000000000000000000, 0.9510565162951535312, 1.000000000000000000, 0.9510565162951535312, 1.000000000000000000, 0.9510565162951535312, 1.000000000000000000, 0.9510565162951535312, 1.000000000000000000, 0.9510565162951535312, 1.000000000000000000, 0.9510565162951535312, 1.000000000000000000, 0.9510565162951535312, 1.000000000000000000, 0.9510565162951535312, 1.000000000000000000, 0.9510565162951535312, 1.000000000000000000, 0.9510565162951535312, 1.000000000000000000, 0.9510565162951535312, 1.000000000000000000, 0.9510565162951535312, 1.000000000000000000, 0.9510565162951535312, 1.000000000000000000, 0.9510565162951535312, 1.000000000000000000, 0.9510565162951535312, 1.000000000000000000, 0.9510565162951535312, 1.000000000000000000, 0.9510565162951535312, 1.000000000000000000, 0.9510565162951535312, 1.000000000000000000, 0.9510565162951535312, 1.000000000000000000, 0.9510565162951535312, 1.000000000000000000, 0.9510565162951535312, 1.000000000000000000, 0.9510565162951535312, 1.000000000000000000, 0.9510565162951535312, 1.000000000000000000, 0.9510565162951535312, 1.000000000000000000, 0.9510565162951535312, 1.000000000000000000, 0.9510565162951535312, 1.000000000000000000, 0.9510565162951535312, 1.000000000000000000, 0.9510565162951535312, 1.000000000000000000, 0.9510565162951535312, 1.000000000000000000, 0.9510565162951535312, 1.000000000000000000, 0.9510565162951535312, 1.000000000000000000, 0.9510565162951535312, 1.000000000000000000, 0.9510565162951535312, 1.000000000000000000, 0.9510565162951535312, 1.000000000000000000, 0.9510565162951535312, 1.000000000000000000, 0.9510565162951535312, 1.000000000000000000, 0.9510565162951535312, 1.000000000000000000, 0.9510565162951535312, 1.000000000000000000, 0.9510565162951535312, 1.000000000000000000, 0.9510565162951535312, 1.000000000000000000, 0.9510565162951535312, 1.000000000000000000, 0.9510565162951535312, 1.000000000000000000, 0.9510565162951535312, 1.000000000000000000, 0.9510565162951535312, 1.000000000000000000, 0.9510565162951535312, 1.000000000000000000, 0.9510565162951535312, 1.000000000000000000, 0.9510565162951535312, 1.000000000000000000, 0.9510565162951535312, 1.000000000000000000, 0.9510565162951535312, 1.000000000000000000, 0.9510565162951535312, 1.000000000000000000, 0.9510565162951535312, 1.000000000000000000, 0.9510565162951535312, 1.000000000000000000, 0.9510565162951535312, 1.000000000000000000, 0.9510565162951535312, 1.000000000000000000, 0.9510565162951535312, 1.000000000000000000, 0.9510565162951535312, 1.000000000000000000, 0.9510565162951535312, 1.000000000000000000, 0.9510565162951535312, 1.000000000000000000),
 ( 1.000000000000000000, 0.9510565162951535312, 1.000000000000000000, 0.9510565162951535312, 1.000000000000000000, 0.9510565162951535312, 1.000000000000000000, 0.9510565162951535312, 1.000000000000000000, 0.9510565162951535312, 1.000000000000000000, 0.9510565162951535312, 1.000000000000000000, 0.9510565162951535312, 1.000000000000000000, 0.9510565162951535312, 1.000000000000000000, 0.9510565162951535312, 1.000000000000000000, 0.9510565162951535312, 1.000000000000000000, 0.9510565162951535312, 1.000000000000000000, 0.9510565162951535312, 1.000000000000000000, 0.9510565162951535312, 1.000000000000000000, 0.9510565162951535312, 1.000000000000000000, 0.9510565162951535312, 1.000000000000000000, 0.9510565162951535312, 1.000000000000000000, 0.9510565162951535312, 1.000000000000000000, 0.9510565162951535312, 1.000000000000000000, 0.9510565162951535312, 1.000000000000000000, 0.9510565162951535312, 1.000000000000000000, 0.9510565162951535312, 1.000000000000000000, 0.9510565162951535312, 1.000000000000000000, 0.9510565162951535312, 1.000000000000000000, 0.9510565162951535312, 1.000000000000000000, 0.9510565162951535312, 1.000000000000000000, 0.9510565162951535312, 1.000000000000000000, 0.9510565162951535312, 1.000000000000000000, 0.9510565162951535312, 1.000000000000000000, 0.9510565162951535312, 1.000000000000000000, 0.9510565162951535312, 1.000000000000000000, 0.9510565162951535312, 1.000000000000000000, 0.9510565162951535312, 1.000000000000000000, 0.9510565162951535312, 1.000000000000000000, 0.9510565162951535312, 1.000000000000000000, 0.9510565162951535312, 1.000000000000000000, 0.9510565162951535312, 1.000000000000000000, 0.9510565162951535312, 1.000000000000000000, 0.9510565162951535312, 1.000000000000000000, 0.9510565162951535312, 1.000000000000000000, 0.9510565162951535312, 1.000000000000000000, 0.9510565162951535312, 1.000000000000000000, 0.9510565162951535312, 1.000000000000000000, 0.9510565162951535312, 1.000000000000000000, 0.9510565162951535312, 1.000000000000000000, 0.9510565162951535312, 1.000000000000000000, 0.9510565162951535312, 1.000000000000000000, 0.9510565162951535312, 1.000000000000000000, 0.9510565162951535312, 1.000000000000000000, 0.9510565162951535312, 1.000000000000000000, 0.9510565162951535312, 1.000000000000000000, 0.9510565162951535312, 1.000000000000000000, 0.9510565162951535312, 1.000000000000000000, 0.9510565162951535312, 1.000000000000000000, 0.9510565162951535312, 1.000000000000000000, 0.9510565162951535312, 1.000000000000000000, 0.9510565162951535312, 1.000000000000000000, 0.9510565162951535312, 1.000000000000000000, 0.9510565162951535312, 1.000000000000000000, 0.9510565162951535312, 1.000000000000000000, 0.9510565162951535312, 1.000000000000000000, 0.9510565162951535312, 1.000000000000000000, 0.9510565162951535312, 1.000000000000000000, 0.9510565162951535312, 1.000000000000000000, 0.9510565162951535312, 1.000000000000000000, 0.9510565162951535312, 1.000000000000000000, 0.9510565162951535312, 1.000000000000000000, 0.9510565162951535312, 1.000000000000000000, 0.9510565162951535312, 1.000000000000000000, 0.9510565162951535312, 1.000000000000000000, 0.9510565162951535312, 1.000000000000000000, 0.9510565162951535312, 1.000000000000000000, 0.9510565162951535312, 1.000000000000000000, 0.9510565162951535312, 1.000000000000000000, 0.9510565162951535312, 1.000000000000000000, 0.9510565162951535312, 1.000000000000000000, 0.9510565162951535312, 1.000000000000000000, 0.9510565162951535312, 1.000000000000000000, 0.9510565162951535312, 1.000000000000000000, 0.9510565162951535312, 1.000000000000000000, 0.9510565162951535312, 1.000000000000000000, 0.9510565162951535312, 1.000000000000000000, 0.9510565162951535312, 1.000000000000000000, 0.9510565162951535312, 1.000000000000000000, 0.9510565162951535312, 1.000000000000000000, 0.9510565162951535312, 1.000000000000000000, 0.9510565162951535312, 1.000000000000000000, 0.9510565162951535312, 1.000000000000000000, 0.9510565162951535312, 1.000000000000000000, 0.9510565162951535312, 1.000000000000000000, 0.9510565162951535312, 1.000000000000000000, 0.9510565162951535312, 1.000000000000000000, 0.9510565162951535312, 1.000000000000000000, 0.9510565162951535312, 1.000000000000000000, 0.9510565162951535312, 1.000000000000000000, 0.9510565162951535312, 1.000000000000000000, 0.9510565162951535312, 1.000000000000000000, 0.9510565162951535312, 1.000000000000000000, 0.9510565162951535312, 1.000000000000000000, 0.9510565162951535312, 1.000000000000000000, 0.9510565162951535312, 1.000000000000000000, 0.9510565162951535312, 1.000000000000000000, 0.9510565162951535312, 1.000000000000000000, 0.9510565162951535312, 1.000000000000000000, 0.9510565162951535312, 1.000000000000000000, 0.9510565162951535312, 1.000000000000000000, 0.9510565162951535312, 1.000000000000000000, 0.9510565162951535312, 1.000000000000000000, 0.9510565162951535312, 1.000000000000000000, 0.9510565162951535312, 1.000000000000000000, 0.9510565162951535312, 1.000000000000000000, 0.9510565162951535312, 1.000000000000000000, 0.9510565162951535312, 1.000000000000000000, 0.9510565162951535312, 1.000000000000000000, 0.9510565162951535312, 1.000000000000000000, 0.9510565162951535312, 1.000000000000000000, 0.9510565162951535312, 1.000000000000000000, 0.9510565162951535312, 1.000000000000000000, 0.9510565162951535312, 1.000000000000000000, 0.9510565162951535312, 1.000000000000000000, 0.9510565162951535312, 1.000000000000000000, 0.9510565162951535312, 1.000000000000000000, 0.9510565162951535312, 1.000000000000000000, 0.9510565162951535312, 1.000000000000000000, 0.9510565162951535312, 1.000000000000000000, 0.9510565162951535312, 1.000000000000000000, 0.9510565162951535312, 1.000000000000000000, 0.9510565162951535312, 1.000000000000000000, 0.9510565162951535312, 1.000000000000000000, 0.9510565162951535312, 1.000000000000000000, 0.9510565162951535312, 1.000000000000000000, 0.9510565162951535312, 1.000000000000000000, 0.9510565162951535312, 1.000000000000000000, 0.9510565162951535312, 1.000000000000000000, 0.9510565162951535312, 1.000000000000000000, 0.9510565162951535312, 1.000000000000000000, 0.9510565162951535312, 1.000000000000000000, 0.9510565162951535312, 1.000000000000000000, 0.9510565162951535312, 1.000000000000000000, 0.9510565162951535312, 1.000000000000000000, 0.9510565162951535312, 1.000000000000000000, 0.9510565162951535312, 1.000000000000000000, 0.9510565162951535312, 1.000000000000000000, 0.9510565162951535312, 1.000000000000000000, 0.9510565162951535312, 1.000000000000000000, 0.9510565162951535312, 1.000000000000000000, 0.9510565162951535312, 1.000000000000000000, 0.9510565162951535312, 1.000000000000000000, 0.9510565162951535312, 1.000000000000000000, 0.9510565162951535312, 1.000000000000000000, 0.9510565162951535312, 1.000000000000000000, 0.9510565162951535312, 1.000000000000000000, 0.9510565162951535312, 1.000000000000000000, 0.9510565162951535312, 1.000000000000000000, 0.9510565162951535312, 1.000000000000000000, 0.9510565162951535312, 1.000000000000000000, 0.9510565162951535312, 1.000000000000000000, 0.9510565162951535312, 1.000000000000000000, 0.9510565162951535312, 1.000000000000000000, 0.9510565162951535312, 1.000000000000000000, 0.9510565162951535312, 1.000000000000000000, 0.9510565162951535312, 1.000000000000000000, 0.9510565162951535312, 1.000000000000000000, 0.9510565162951535312, 1.000000000000000000, 0.9510565162951535312, 1.000000000000000000, 0.9510565162951535312, 1.000000000000000000, 0.9510565162951535312, 1.000000000000000000, 0.9510565162951535312, 1.000000000000000000, 0.9510565162951535312, 1.000000000000000000, 0.9510565162951535312, 1.000000000000000000, 0.9510565162951535312, 1.000000000000000000, 0.9510565162951535312, 1.000000000000000000, 0.9510565162951535312, 1.000000000000000000, 0.9510565162951535312, 1.000000000000000000, 0.9510565162951535312, 1.000000000000000000, 0.9510565162951535312, 1.000000000000000000, 0.9510565162951535312, 1.000000000000000000, 0.9510565162951535312, 1.000000000000000000, 0.9510565162951535312, 1.000000000000000000, 0.9510565162951535312, 1.000000000000000000, 0.9510565162951535312, 1.000000000000000000, 0.9510565162951535312, 1.000000000000000000, 0.9510565162951535312, 1.000000000000000000, 0.9510565162951535312, 1.000000000000000000, 0.9510565162951535312, 1.000000000000000000, 0.9510565162951535312, 1.000000000000000000, 0.9510565162951535312, 1.000000000000000000, 0.9510565162951535312, 1.000000000000000000, 0.9510565162951535312, 1.000000000000000000, 0.9510565162951535312, 1.000000000000000000, 0.9510565162951535312, 1.000000000000000000, 0.9510565162951535312, 1.000000000000000000, 0.9510565162951535312, 1.000000000000000000, 0.9510565162951535312, 1.000000000000000000, 0.9510565162951535312, 1.000000000000000000, 0.9510565162951535312, 1.000000000000000000, 0.9510565162951535312, 1.000000000000000000, 0.9510565162951535312, 1.000000000000000000, 0.9510565162951535312, 1.000000000000000000, 0.9510565162951535312, 1.000000000000000000, 0.9510565162951535312, 1.000000000000000000, 0.9510565162951535312, 1.000000000000000000, 0.9510565162951535312, 1.000000000000000000, 0.9510565162951535312, 1.000000000000000000, 0.9510565162951535312, 1.000000000000000000, 0.9510565162951535312, 1.000000000000000000, 0.9510565162951535312, 1.000000000000000000, 0.9510565162951535312, 1.000000000000000000, 0.9510565162951535312, 1.000000000000000000, 0.9510565162951535312, 1.000000000000000000, 0.9510565162951535312, 1.000000000000000000, 0.9510565162951535312, 1.000000000000000000, 0.9510565162951535312, 1.000000000000000000, 0.9510565162951535312, 1.000000000000000000, 0.9510565162951535312, 1.000000000000000000, 0.9510565162951535312, 1.000000000000000000, 0.9510565162951535312, 1.000000000000000000, 0.9510565162951535312, 1.000000000000000000, 0.9510565162951535312, 1.000000000000000000, 0.9510565162951535312, 1.000000000000000000, 0.9510565162951535312, 1.000000000000000000, 0.9510565162951535312, 1.000000000000000000, 0.9510565162951535312, 1.000000000000000000, 0.9510565162951535312, 1.000000000000000000, 0.9510565162951535312, 1.000000000000000000, 0.9510565162951535312, 1.000000000000000000, 0.9510565162951535312, 1.000000000000000000, 0.9510565162951535312, 1.000000000000000000, 0.9510565162951535312, 1.000000000000000000, 0.9510565162951535312, 1.000000000000000000, 0.9510565162951535312, 1.000000000000000000, 0.9510565162951535312, 1.000000000000000000, 0.9510565162951535312, 1.000000000000000000, 0.9510565162951535312, 1.000000000000000000, 0.9510565162951535312, 1.000000000000000000, 0.9510565162951535312, 1.000000000000000000, 0.9510565162951535312, 1.000000000000000000, 0.9510565162951535312, 1.000000000000000000, 0.9510565162951535312, 1.000000000000000000, 0.9510565162951535312, 1.000000000000000000, 0.9510565162951535312, 1.000000000000000000, 0.9510565162951535312, 1.000000000000000000, 0.9510565162951535312, 1.000000000000000000, 0.9510565162951535312, 1.000000000000000000, 0.9510565162951535312, 1.000000000000000000, 0.9510565162951535312, 1.000000000000000000, 0.9510565162951535312, 1.000000000000000000, 0.9510565162951535312, 1.000000000000000000, 0.9510565162951535312, 1.000000000000000000, 0.9510565162951535312, 1.000000000000000000, 0.9510565162951535312, 1.000000000000000000, 0.9510565162951535312, 1.000000000000000000, 0.9510565162951535312, 1.000000000000000000, 0.9510565162951535312, 1.000000000000000000, 0.9510565162951535312, 1.000000000000000000, 0.9510565162951535312, 1.000000000000000000, 0.9510565162951535312, 1.000000000000000000, 0.9510565162951535312, 1.000000000000000000, 0.9510565162951535312, 1.000000000000000000, 0.9510565162951535312, 1.000000000000000000, 0.9510565162951535312, 1.000000000000000000, 0.9510565162951535312, 1.000000000000000000, 0.9510565162951535312, 1.000000000000000000, 0.9510565162951535312, 1.000000000000000000, 0.9510565162951535312, 1.000000000000000000, 0.9510565162951535312, 1.000000000000000000, 0.9510565162951535312, 1.000000000000000000, 0.9510565162951535312, 1.000000000000000000, 0.9510565162951535312, 1.000000000000000000, 0.9510565162951535312, 1.000000000000000000, 0.9510565162951535312, 1.000000000000000000, 0.9510565162951535312, 1.000000000000000000, 0.9510565162951535312, 1.000000000000000000, 0.9510565162951535312, 1.000000000000000000, 0.9510565162951535312, 1.000000000000000000, 0.9510565162951535312, 1.000000000000000000, 0.9510565162951535312, 1.000000000000000000, 0.9510565162951535312, 1.000000000000000000, 0.9510565162951535312, 1.000000000000000000, 0.9510565162951535312, 1.000000000000000000, 0.9510565162951535312, 1.000000000000000000, 0.9510565162951535312, 1.000000000000000000, 0.9510565162951535312, 1.000000000000000000, 0.9510565162951535312, 1.000000000000000000, 0.9510565162951535312, 1.000000000000000000, 0.9510565162951535312, 1.000000000000000000, 0.9510565162951535312, 1.000000000000000000, 0.9510565162951535312, 1.000000000000000000, 0.9510565162951535312, 1.000000000000000000, 0.9510565162951535312, 1.000000000000000000, 0.9510565162951535312, 1.000000000000000000, 0.9510565162951535312, 1.000000000000000000, 0.9510565162951535312, 1.000000000000000000, 0.9510565162951535312, 1.000000000000000000, 0.9510565162951535312, 1.000000000000000000, 0.9510565162951535312, 1.000000000000000000, 0.9510565162951535312, 1.000000000000000000, 0.9510565162951535312, 1.000000000000000000, 0.9510565162951535312, 1.000000000000000000, 0.9510565162951535312, 1.000000000000000000, 0.9510565162951535312, 1.000000000000000000, 0.9510565162951535312, 1.000000000000000000, 0.9510565162951535312, 1.000000000000000000, 0.9510565162951535312, 1.000000000000000000, 0.9510565162951535312, 1.000000000000000000, 0.9510565162951535312, 1.000000000000000000, 0.9510565162951535312, 1.000000000000000000, 0.9510565162951535312, 1.000000000000000000, 0.9510565162951535312, 1.000000000000000000, 0.9510565162951535312, 1.000000000000000000, 0.9510565162951535312, 1.000000000000000000, 0.9510565162951535312, 1.000000000000000000, 0.9510565162951535312, 1.000000000000000000, 0.9510565162951535312, 1.000000000000000000, 0.9510565162951535312, 1.000000000000000000, 0.9510565162951535312, 1.000000000000000000, 0.9510565162951535312, 1.000000000000000000, 0.9510565162951535312, 1.000000000000000000, 0.9510565162951535312, 1.000000000000000000, 0.9510565162951535312, 1.000000000000000000, 0.9510565162951535312, 1.000000000000000000, 0.9510565162951535312, 1.000000000000000000, 0.9510565162951535312, 1.000000000000000000, 0.9510565162951535312, 1.000000000000000000, 0.9510565162951535312, 1.000000000000000000, 0.9510565162951535312, 1.000000000000000000, 0.9510565162951535312, 1.000000000000000000, 0.9510565162951535312, 1.000000000000000000, 0.9510565162951535312, 1.000000000000000000, 0.9510565162951535312, 1.000000000000000000, 0.9510565162951535312, 1.000000000000000000, 0.9510565162951535312, 1.000000000000000000, 0.9510565162951535312, 1.000000000000000000, 0.9510565162951535312, 1.000000000000000000, 0.9510565162951535312, 1.000000000000000000, 0.9510565162951535312, 1.000000000000000000, 0.9510565162951535312, 1.000000000000000000, 0.9510565162951535312, 1.000000000000000000, 0.9510565162951535312, 1.000000000000000000, 0.9510565162951535312, 1.000000000000000000, 0.9510565162951535312, 1.000000000000000000, 0.9510565162951535312, 1.000000000000000000, 0.9510565162951535312, 1.000000000000000000, 0.9510565162951535312, 1.000000000000000000, 0.9510565162951535312, 1.000000000000000000, 0.9510565162951535312, 1.000000000000000000, 0.9510565162951535312, 1.000000000000000000, 0.9510565162951535312, 1.000000000000000000, 0.9510565162951535312, 1.000000000000000000, 0.9510565162951535312, 1.000000000000000000, 0.9510565162951535312, 1.000000000000000000, 0.9510565162951535312, 1.000000000000000000, 0.9510565162951535312, 1.000000000000000000, 0.9510565162951535312, 1.000000000000000000, 0.9510565162951535312, 1.000000000000000000, 0.9510565162951535312, 1.000000000000000000, 0.9510565162951535312, 1.000000000000000000, 0.9510565162951535312, 1.000000000000000000, 0.9510565162951535312, 1.000000000000000000, 0.9510565162951535312, 1.000000000000000000, 0.9510565162951535312, 1.000000000000000000, 0.9510565162951535312, 1.000000000000000000, 0.9510565162951535312, 1.000000000000000000, 0.9510565162951535312, 1.000000000000000000, 0.9510565162951535312, 1.000000000000000000, 0.9510565162951535312, 1.000000000000000000, 0.9510565162951535312, 1.000000000000000000, 0.9510565162951535312, 1.000000000000000000, 0.9510565162951535312, 1.000000000000000000, 0.9510565162951535312, 1.000000000000000000, 0.9510565162951535312, 1.000000000000000000, 0.9510565162951535312, 1.000000000000000000, 0.9510565162951535312, 1.000000000000000000, 0.9510565162951535312, 1.000000000000000000, 0.9510565162951535312, 1.000000000000000000, 0.9510565162951535312, 1.000000000000000000, 0.9510565162951535312, 1.000000000000000000, 0.9510565162951535312, 1.000000000000000000, 0.9510565162951535312, 1.000000000000000000, 0.9510565162951535312, 1.000000000000000000, 0.9510565162951535312, 1.000000000000000000, 0.9510565162951535312, 1.000000000000000000, 0.9510565162951535312, 1.000000000000000000, 0.9510565162951535312, 1.000000000000000000, 0.9510565162951535312, 1.000000000000000000, 0.9510565162951535312, 1.000000000000000000, 0.9510565162951535312, 1.000000000000000000, 0.9510565162951535312, 1.000000000000000000, 0.9510565162951535312, 1.000000000000000000, 0.9510565162951535312, 1.000000000000000000, 0.9510565162951535312, 1.000000000000000000) ) ) 
 REPRESENTATION_ITEM ( '' )  SURFACE ( )  );
#10690=CARTESIAN_POINT ( 'NONE',  ( 33.58253175000000823, 52.02500000273118985, 10.91162601494192863 ) ) ;
#10691=CARTESIAN_POINT ( 'NONE',  ( -10.37757302488623701, 19.77500000273117564, 31.93888565452638417 ) ) ;
#10692=CARTESIAN_POINT ( 'NONE',  ( -33.58253175000000113, 5.275000002731187188, -10.91162601494193218 ) ) ;
#10696=CARTESIAN_POINT ( 'NONE',  ( 26.29305231718578995, 71.70000000546238539, -19.10302069950538240 ) ) ;
#10697=CARTESIAN_POINT ( 'NONE',  ( 32.61426705943282656, 52.00000000000002842, 7.648559219946585053 ) ) ;
#10704=CARTESIAN_POINT ( 'NONE',  ( 33.58253175000000823, 48.27500000273119696, 10.91162601494192863 ) ) ;
#10709=CARTESIAN_POINT ( 'NONE',  ( -20.75514604977248823, 26.82500000273117280, -28.56700777964554305 ) ) ;
#10723=CARTESIAN_POINT ( 'NONE',  ( 5.779280353836490358E-15, 65.00000000546236834, 32.49999999999999289 ) ) ;
#10725=ADVANCED_BREP_SHAPE_REPRESENTATION ( '', ( #32129, #1376 ), #10174 ) ;
#10726=CARTESIAN_POINT ( 'NONE',  ( -32.50000000000000000, 18.00000000000000355, 0.000000000000000000 ) ) ;
#10732=CARTESIAN_POINT ( 'NONE',  ( 20.75514604977249178, 73.82500000273121543, 28.56700777964553950 ) ) ;
#10733=CARTESIAN_POINT ( 'NONE',  ( 33.58253175000000823, 36.27500000273119696, 10.91162601494192863 ) ) ;
#10739=CARTESIAN_POINT ( 'NONE',  ( -20.08610463437156923, 56.29999999999999716, 27.64615127144130113 ) ) ;
#10745=CARTESIAN_POINT ( 'NONE',  ( -10.37757302488624411, 72.97500000273120691, -31.93888565452638417 ) ) ;
#10747=AXIS2_PLACEMENT_3D ( 'NONE', #21490, #21328, #26126 ) ;
#10751=CARTESIAN_POINT ( 'NONE',  ( -33.58253175000000113, 45.02500000273117564, -10.91162601494193218 ) ) ;
#10755=CARTESIAN_POINT ( 'NONE',  ( -12.90513655866680587, 66.99999999999998579, -31.00393344628902881 ) ) ;
#10756=CARTESIAN_POINT ( 'NONE',  ( 32.50000000000000711, 7.400000005462386454, 10.55989012756945122 ) ) ;
#10776=CARTESIAN_POINT ( 'NONE',  ( -27.16883889988624290, 57.17500000273119554, -19.73931689729374028 ) ) ;
#10782=CARTESIAN_POINT ( 'NONE',  ( -10.04305231718578462, 74.40000000000000568, 30.90933677959249337 ) ) ;
#10783=CARTESIAN_POINT ( 'NONE',  ( 10.37757302488624767, 13.72500000273117671, 31.93888565452638417 ) ) ;
#10787=CARTESIAN_POINT ( 'NONE',  ( -20.08610463437156923, 34.80000000546240102, 27.64615127144130113 ) ) ;
#10793=CARTESIAN_POINT ( 'NONE',  ( -27.16883889988623935, 61.32500000273120833, 19.73931689729374739 ) ) ;
#10797=CARTESIAN_POINT ( 'NONE',  ( 20.75514604977249178, 7.825000002731194115, 28.56700777964553950 ) ) ;
#10807=CARTESIAN_POINT ( 'NONE',  ( 32.50000000000000000, 21.00000000000000355, -3.980102097228898626E-15 ) ) ;
#10811=CARTESIAN_POINT ( 'NONE',  ( -21.25115026575266697, 67.00000000000004263, 25.10892607490235306 ) ) ;
#10818=CARTESIAN_POINT ( 'NONE',  ( 7.689115195225237898, 67.00000000000000000, -32.34176759466016904 ) ) ;
#10819=CARTESIAN_POINT ( 'NONE',  ( 2.376701315729479624, 51.99999999999999289, 33.34874525913693333 ) ) ;
#10820=CARTESIAN_POINT ( 'NONE',  ( -10.37757302488624411, 36.72500000273119980, -31.93888565452638417 ) ) ;
#10822=CARTESIAN_POINT ( 'NONE',  ( 27.16883889988623935, 52.57500000273117280, -19.73931689729374384 ) ) ;
#10825=CARTESIAN_POINT ( 'NONE',  ( 32.50000000000000000, 51.50000000546238255, -3.980102097228898626E-15 ) ) ;
#10831=CARTESIAN_POINT ( 'NONE',  ( 20.75514604977248467, 28.67500000273117777, -28.56700777964554305 ) ) ;
#10835=CARTESIAN_POINT ( 'NONE',  ( -32.50000000000000000, 14.60000000546239107, 10.55989012756946366 ) ) ;
#10847=CARTESIAN_POINT ( 'NONE',  ( 10.37757302488624056, 56.52500000273118275, -31.93888565452638417 ) ) ;
#10858=CARTESIAN_POINT ( 'NONE',  ( -20.75514604977248112, 67.67500000273116711, 28.56700777964554661 ) ) ;
#10859=ORIENTED_EDGE ( 'NONE', *, *, #12067, .T. ) ;
#10863=CARTESIAN_POINT ( 'NONE',  ( -2.162160676586881955E-15, 54.62500000273116996, -35.31076352940723240 ) ) ;
#10864=CARTESIAN_POINT ( 'NONE',  ( -2.162160676586881955E-15, 14.87500000273120193, -35.31076352940723240 ) ) ;
#10865=CARTESIAN_POINT ( 'NONE',  ( 20.75514604977248467, 2.675000002731181770, -28.56700777964554305 ) ) ;
#10869=CARTESIAN_POINT ( 'NONE',  ( 32.50000000000000711, 75.40000000546240244, 10.55989012756945122 ) ) ;
#10876=CARTESIAN_POINT ( 'NONE',  ( -27.16883889988623935, 45.57500000273119412, 19.73931689729374739 ) ) ;
#10881=CARTESIAN_POINT ( 'NONE',  ( -27.16883889988624290, 20.92500000273118843, -19.73931689729374028 ) ) ;
#10897=CARTESIAN_POINT ( 'NONE',  ( -32.50000000000000000, 9.899999999999991473, -10.55989012756945478 ) ) ;
#10904=CARTESIAN_POINT ( 'NONE',  ( -2.162160676586881955E-15, 70.62500000273118417, -35.31076352940723240 ) ) ;
#10905=CARTESIAN_POINT ( 'NONE',  ( 27.16883889988623935, 34.57500000273118701, -19.73931689729374384 ) ) ;
#10910=CARTESIAN_POINT ( 'NONE',  ( 26.29305231718578995, 51.20000000000000995, -19.10302069950538240 ) ) ;
#10915=CARTESIAN_POINT ( 'NONE',  ( 33.58253175000000823, 66.27500000273118985, 10.91162601494192863 ) ) ;
#10920=CARTESIAN_POINT ( 'NONE',  ( 33.58253175000000113, 34.22500000273117848, -10.91162601494193751 ) ) ;
#10937=CARTESIAN_POINT ( 'NONE',  ( 40.00000000000000000, 52.00000000000000711, 23.09401076758503990 ) ) ;
#10942=CARTESIAN_POINT ( 'NONE',  ( -33.58253175000000113, 55.27500000273120406, -10.91162601494193218 ) ) ;
#10949=CARTESIAN_POINT ( 'NONE',  ( -32.50000000000000000, 73.90000000000003411, -10.55989012756945478 ) ) ;
#10950=CARTESIAN_POINT ( 'NONE',  ( -2.162160676586881955E-15, 8.625000002731180615, -35.31076352940723240 ) ) ;
#10958=CARTESIAN_POINT ( 'NONE',  ( 6.486482029760649416E-15, 59.62500000273118417, 35.31076352940723240 ) ) ;
#10962=CARTESIAN_POINT ( 'NONE',  ( -10.37757302488624411, 4.725000002731183812, -31.93888565452638417 ) ) ;
#10973=CARTESIAN_POINT ( 'NONE',  ( -32.50000000000000000, 24.09999999999999787, 10.55989012756946366 ) ) ;
#10977=CARTESIAN_POINT ( 'NONE',  ( -31.04172217648553556, 66.99999999999998579, -12.81397374188210136 ) ) ;
#10987=CARTESIAN_POINT ( 'NONE',  ( -5.714234795769386643, 52.00000000000003553, 32.80324308525976562 ) ) ;
#10989=CARTESIAN_POINT ( 'NONE',  ( 33.58253175000000113, 30.22500000273118559, -10.91162601494193751 ) ) ;
#10990=CARTESIAN_POINT ( 'NONE',  ( 20.08610463437157279, 65.29999999999999716, -27.64615127144129758 ) ) ;
#10994=CARTESIAN_POINT ( 'NONE',  ( -10.04305231718578462, 54.90000000546239534, 30.90933677959249337 ) ) ;
#11005=CARTESIAN_POINT ( 'NONE',  ( 10.04305231718578817, 19.90000000546236691, -30.90933677959249337 ) ) ;
#11015=CARTESIAN_POINT ( 'NONE',  ( -33.58253175000000113, 55.22500000273117848, 10.91162601494193929 ) ) ;
#11024=CARTESIAN_POINT ( 'NONE',  ( 33.58253175000000113, 66.47500000273119269, -10.91162601494193751 ) ) ;
#11029=CARTESIAN_POINT ( 'NONE',  ( -20.75514604977248823, 50.82500000273116569, -28.56700777964554305 ) ) ;
#11030=CARTESIAN_POINT ( 'NONE',  ( -20.75514604977248112, 9.675000002731193760, 28.56700777964554661 ) ) ;
#11031=CARTESIAN_POINT ( 'NONE',  ( -20.75514604977248823, 65.07500000273118701, -28.56700777964554305 ) ) ;
#11035=CARTESIAN_POINT ( 'NONE',  ( -26.29305231718578995, 72.70000000546238539, 19.10302069950538595 ) ) ;
#11045=CARTESIAN_POINT ( 'NONE',  ( 20.75514604977248467, 44.67500000273118843, -28.56700777964554305 ) ) ;
#11047=VECTOR ( 'NONE', #9019, 1000.000000000000000 ) ;
#11052=CARTESIAN_POINT ( 'NONE',  ( -20.75514604977248112, 19.42500000273117777, 28.56700777964554661 ) ) ;
#11063=CARTESIAN_POINT ( 'NONE',  ( -20.08610463437156923, 64.29999999999996874, 27.64615127144130113 ) ) ;
#11066=CARTESIAN_POINT ( 'NONE',  ( -26.29305231718579350, 9.800000000000016698, -19.10302069950537884 ) ) ;
#11072=CARTESIAN_POINT ( 'NONE',  ( -33.58253175000000113, 71.02500000273118985, -10.91162601494193218 ) ) ;
#11074=CARTESIAN_POINT ( 'NONE',  ( -10.37757302488623701, 29.77500000273118630, 31.93888565452638417 ) ) ;
#11079=CARTESIAN_POINT ( 'NONE',  ( -32.50000000000000000, 56.00000000000000711, 0.000000000000000000 ) ) ;
#11080=DIRECTION ( 'NONE',  ( 0.000000000000000000, -0.000000000000000000, 1.000000000000000000 ) ) ;
#11084=CARTESIAN_POINT ( 'NONE',  ( -20.75514604977248112, 65.67500000273118133, 28.56700777964554661 ) ) ;
#11089=EDGE_LOOP ( 'NONE', ( #5344, #9676, #30223, #30819 ) ) ;
#11090=CARTESIAN_POINT ( 'NONE',  ( 10.37757302488624056, 38.52500000273119696, -31.93888565452638417 ) ) ;
#11096=CARTESIAN_POINT ( 'NONE',  ( 10.04305231718578817, 59.39999999999999147, -30.90933677959249337 ) ) ;
#11111=VECTOR ( 'NONE', #2031, 1000.000000000000000 ) ;
#11113=CARTESIAN_POINT ( 'NONE',  ( 20.75514604977248467, 56.67500000273119554, -28.56700777964554305 ) ) ;
#11120=CARTESIAN_POINT ( 'NONE',  ( -10.04305231718578462, 72.40000000000000568, 30.90933677959249337 ) ) ;
#11121=CARTESIAN_POINT ( 'NONE',  ( 10.37757302488624767, 11.72500000273117493, 31.93888565452638417 ) ) ;
#11128=ORIENTED_EDGE ( 'NONE', *, *, #20063, .T. ) ;
#11129=CARTESIAN_POINT ( 'NONE',  ( -2.162160676586881955E-15, 58.62500000273118417, -35.31076352940723240 ) ) ;
#11144=CARTESIAN_POINT ( 'NONE',  ( 32.50000000000000000, 23.09999999999999787, -10.55989012756945833 ) ) ;
#11154=CARTESIAN_POINT ( 'NONE',  ( 32.46022989551244819, 67.00000000000000000, -2.703243202363984299 ) ) ;
#11156=CARTESIAN_POINT ( 'NONE',  ( -20.75514604977248112, 29.42500000273118133, 28.56700777964554661 ) ) ;
#11157=CARTESIAN_POINT ( 'NONE',  ( -32.50000000000000000, 56.60000000546236976, 10.55989012756946366 ) ) ;
#11158=CARTESIAN_POINT ( 'NONE',  ( 10.04305231718579705, 61.10000000546238397, 30.90933677959248982 ) ) ;
#11162=CARTESIAN_POINT ( 'NONE',  ( -2.092463501923844636E-15, 48.00000000546238255, -34.17252228774368916 ) ) ;
#11164=CARTESIAN_POINT ( 'NONE',  ( -26.29305231718578995, 58.70000000546237118, 19.10302069950538595 ) ) ;
#11167=CARTESIAN_POINT ( 'NONE',  ( 33.58253175000000113, 74.22500000273119269, -10.91162601494193751 ) ) ;
#11172=CARTESIAN_POINT ( 'NONE',  ( -10.04305231718579172, 16.10000000546236976, -30.90933677959248982 ) ) ;
#11190=CARTESIAN_POINT ( 'NONE',  ( -10.37757302488624411, 68.97500000273119269, -31.93888565452638417 ) ) ;
#11195=CARTESIAN_POINT ( 'NONE',  ( -10.37757302488623701, 47.52500000273117564, 31.93888565452638417 ) ) ;
#11196=CARTESIAN_POINT ( 'NONE',  ( -27.16883889988624290, 13.17500000273118310, -19.73931689729374028 ) ) ;
#11197=CARTESIAN_POINT ( 'NONE',  ( -10.37757302488623701, 59.77500000273121117, 31.93888565452638417 ) ) ;
#11201=CARTESIAN_POINT ( 'NONE',  ( 10.04305231718579705, 67.10000000546239107, 30.90933677959248982 ) ) ;
#11208=CARTESIAN_POINT ( 'NONE',  ( 10.37757302488624056, 46.77500000273120406, -31.93888565452638417 ) ) ;
#11213=CARTESIAN_POINT ( 'NONE',  ( 10.37757302488624767, 19.72500000273118204, 31.93888565452638417 ) ) ;
#11227=CARTESIAN_POINT ( 'NONE',  ( 6.277390505771533514E-15, 10.49999999999998757, 34.17252228774368916 ) ) ;
#11233=CARTESIAN_POINT ( 'NONE',  ( 6.486482029760649416E-15, 69.62500000273118417, 35.31076352940723240 ) ) ;
#11234=CARTESIAN_POINT ( 'NONE',  ( -2.162160676586881955E-15, 30.87500000273119483, -35.31076352940723240 ) ) ;
#11235=CARTESIAN_POINT ( 'NONE',  ( -10.37757302488623701, 15.77500000273117386, 31.93888565452638417 ) ) ;
#11242=CARTESIAN_POINT ( 'NONE',  ( -32.50000000000000000, 56.10000000000000853, 10.55989012756946366 ) ) ;
#11248=CARTESIAN_POINT ( 'NONE',  ( -33.58253175000000113, 67.27500000273117564, -10.91162601494193218 ) ) ;
#11253=CARTESIAN_POINT ( 'NONE',  ( 33.58253175000000823, 36.02500000273117564, 10.91162601494192863 ) ) ;
#11258=CARTESIAN_POINT ( 'NONE',  ( 33.58253175000000113, 66.47500000273119269, -10.91162601494193574 ) ) ;
#11259=CARTESIAN_POINT ( 'NONE',  ( 32.50000000000000000, 59.09999999999999432, -10.55989012756945833 ) ) ;
#11276=CARTESIAN_POINT ( 'NONE',  ( -10.37757302488624411, 48.97500000273117848, -31.93888565452638417 ) ) ;
#11282=CARTESIAN_POINT ( 'NONE',  ( -10.04305231718579172, 73.59999999999998010, -30.90933677959248982 ) ) ;
#11283=CARTESIAN_POINT ( 'NONE',  ( 27.16883889988624290, 7.925000002731205306, 19.73931689729373673 ) ) ;
#11285=CYLINDRICAL_SURFACE ( 'NONE', #24781, 32.50000000000000000 ) ;
#11292=CARTESIAN_POINT ( 'NONE',  ( -27.16883889988624290, 56.92500000273119554, -19.73931689729374028 ) ) ;
#11305=CARTESIAN_POINT ( 'NONE',  ( 20.08610463437157279, 23.29999999999999361, -27.64615127144129758 ) ) ;
#11313=EDGE_CURVE ( 'NONE', #25517, #31633, #9979, .T. ) ;
#11316=CARTESIAN_POINT ( 'NONE',  ( -2.162160676586881955E-15, 28.62500000273118062, -35.31076352940723240 ) ) ;
#11322=CARTESIAN_POINT ( 'NONE',  ( -10.04305231718579172, 48.10000000546236976, -30.90933677959248982 ) ) ;
#11325=ORIENTED_EDGE ( 'NONE', *, *, #3903, .T. ) ;
#11326=CARTESIAN_POINT ( 'NONE',  ( -33.58253175000000113, 73.02500000273120406, -10.91162601494193218 ) ) ;
#11332=CARTESIAN_POINT ( 'NONE',  ( -20.08610463437156923, 10.80000000546236549, 27.64615127144130113 ) ) ;
#11350=CARTESIAN_POINT ( 'NONE',  ( -27.16883889988623935, 69.57500000273118701, 19.73931689729374739 ) ) ;
#11354=EDGE_CURVE ( 'NONE', #19648, #17565, #32951, .T. ) ;
#11356=CARTESIAN_POINT ( 'NONE',  ( 33.58253175000000113, 46.12500000273119127, -4.112674001490185761E-15 ) ) ;
#11357=CARTESIAN_POINT ( 'NONE',  ( 10.37757302488624056, 8.775000002731166759, -31.93888565452638417 ) ) ;
#11358=CARTESIAN_POINT ( 'NONE',  ( 10.37757302488624056, 64.77500000273118985, -31.93888565452638417 ) ) ;
#11364=CARTESIAN_POINT ( 'NONE',  ( 20.08610463437158344, 65.20000000546235697, 27.64615127144129403 ) ) ;
#11370=CARTESIAN_POINT ( 'NONE',  ( 6.486482029760649416E-15, 49.87500000273119838, 35.31076352940723240 ) ) ;
#11375=CARTESIAN_POINT ( 'NONE',  ( -27.16883889988623935, 19.32500000273117280, 19.73931689729374739 ) ) ;
#11388=CARTESIAN_POINT ( 'NONE',  ( -10.04305231718578462, 12.40000000000000746, 30.90933677959249337 ) ) ;
#11394=CARTESIAN_POINT ( 'NONE',  ( 33.58253175000000113, 68.22500000273116427, -10.91162601494193751 ) ) ;
#11395=CARTESIAN_POINT ( 'NONE',  ( 27.16883889988623935, 30.57500000273117990, -19.73931689729374384 ) ) ;
#11396=CARTESIAN_POINT ( 'NONE',  ( -33.58253175000000113, 19.37500000273119483, 0.000000000000000000 ) ) ;
#11402=CARTESIAN_POINT ( 'NONE',  ( 6.277390505771533514E-15, 44.49999999999999289, 34.17252228774368916 ) ) ;
#11408=CARTESIAN_POINT ( 'NONE',  ( 33.58253175000000113, 68.37500000273121259, -4.112674001490185761E-15 ) ) ;
#11413=CARTESIAN_POINT ( 'NONE',  ( 20.75514604977249178, 37.82500000273117280, 28.56700777964553950 ) ) ;
#11430=LINE ( 'NONE', #10937, #11047 ) ;
#11434=CARTESIAN_POINT ( 'NONE',  ( 10.37757302488624056, 48.77500000273120406, -31.93888565452638417 ) ) ;
#11438=DIRECTION ( 'NONE',  ( 0.000000000000000000, 0.000000000000000000, 1.000000000000000000 ) ) ;
#11440=CARTESIAN_POINT ( 'NONE',  ( -10.04305231718579172, 65.60000000000000853, -30.90933677959248982 ) ) ;
#11441=CARTESIAN_POINT ( 'NONE',  ( 6.486482029760649416E-15, 11.62500000273118950, 35.31076352940723240 ) ) ;
#11452=CARTESIAN_POINT ( 'NONE',  ( 20.75514604977249178, 53.82500000273119412, 28.56700777964553950 ) ) ;
#11454=CARTESIAN_POINT ( 'NONE',  ( -33.58253175000000113, 31.37500000273117706, 0.000000000000000000 ) ) ;
#11458=DIRECTION ( 'NONE',  ( 0.000000000000000000, 0.000000000000000000, 1.000000000000000000 ) ) ;
#11480=CARTESIAN_POINT ( 'NONE',  ( -15.83883214465799405, 52.00000000000004263, 29.08710441171866279 ) ) ;
#11481=CARTESIAN_POINT ( 'NONE',  ( -20.75514604977248823, 28.82500000273116569, -28.56700777964554305 ) ) ;
#11482=CARTESIAN_POINT ( 'NONE',  ( -26.29305231718579350, 56.30000000546238681, -19.10302069950537884 ) ) ;
#11484=CARTESIAN_POINT ( 'NONE',  ( 10.04305231718579705, 60.60000000000000142, 30.90933677959248982 ) ) ;
#11486=CARTESIAN_POINT ( 'NONE',  ( 10.04305231718578817, 47.90000000546239534, -30.90933677959249337 ) ) ;
#11489=CARTESIAN_POINT ( 'NONE',  ( -2.162160676586881955E-15, 74.62500000273116996, -35.31076352940723240 ) ) ;
#11492=ORIENTED_EDGE ( 'NONE', *, *, #32206, .T. ) ;
#11494=CARTESIAN_POINT ( 'NONE',  ( 20.08610463437158344, 9.200000005462387165, 27.64615127144129403 ) ) ;
#11503=CARTESIAN_POINT ( 'NONE',  ( -2.092463501923844636E-15, 35.49999999999998579, -34.17252228774368916 ) ) ;
#11511=CARTESIAN_POINT ( 'NONE',  ( 10.37757302488624767, 65.97500000273119269, 31.93888565452638417 ) ) ;
#11516=CARTESIAN_POINT ( 'NONE',  ( 27.16883889988623935, 48.32500000273119412, -19.73931689729374384 ) ) ;
#11517=CARTESIAN_POINT ( 'NONE',  ( 20.75514604977248467, 12.67500000273118488, -28.56700777964554305 ) ) ;
#11518=CARTESIAN_POINT ( 'NONE',  ( 33.58253175000000113, 60.37500000273120548, -4.112674001490185761E-15 ) ) ;
#11522=CARTESIAN_POINT ( 'NONE',  ( -20.08610463437157989, 66.20000000546238539, -27.64615127144129758 ) ) ;
#11528=CARTESIAN_POINT ( 'NONE',  ( -33.58253175000000113, 41.37500000273118417, 0.000000000000000000 ) ) ;
#11530=CARTESIAN_POINT ( 'NONE',  ( -32.50000000000000000, 32.50000000546236834, 0.000000000000000000 ) ) ;
#11532=CARTESIAN_POINT ( 'NONE',  ( -33.58253175000000113, 17.22500000273118559, 10.91162601494193929 ) ) ;
#11550=CARTESIAN_POINT ( 'NONE',  ( 10.04305231718578817, 11.40000000000000746, -30.90933677959249337 ) ) ;
#11556=CARTESIAN_POINT ( 'NONE',  ( -2.162160676586881955E-15, 66.62500000273118417, -35.31076352940723240 ) ) ;
#11557=CARTESIAN_POINT ( 'NONE',  ( -10.37757302488623701, 31.77500000273118630, 31.93888565452638417 ) ) ;
#11558=CARTESIAN_POINT ( 'NONE',  ( 20.75514604977248467, 16.67500000273117777, -28.56700777964554305 ) ) ;
#11564=CARTESIAN_POINT ( 'NONE',  ( 32.50000000000000711, 48.89999999999999858, 10.55989012756945122 ) ) ;
#11571=CARTESIAN_POINT ( 'NONE',  ( -27.16883889988624290, 67.17500000273118133, -19.73931689729374028 ) ) ;
#11577=CARTESIAN_POINT ( 'NONE',  ( 10.37757302488624767, 37.72500000273119980, 31.93888565452638417 ) ) ;
#11599=CARTESIAN_POINT ( 'NONE',  ( 33.58253175000000823, 50.27500000273118985, 10.91162601494192863 ) ) ;
#11605=CARTESIAN_POINT ( 'NONE',  ( -32.50000000000000000, 67.99999999999998579, 0.000000000000000000 ) ) ;
#11606=CARTESIAN_POINT ( 'NONE',  ( 27.16883889988623935, 6.325000002731187898, -19.73931689729374384 ) ) ;
#11616=CARTESIAN_POINT ( 'NONE',  ( -10.37757302488624411, 58.72500000273119269, -31.93888565452638417 ) ) ;
#11617=CARTESIAN_POINT ( 'NONE',  ( 27.16883889988623935, 30.57500000273117990, -19.73931689729374384 ) ) ;
#11630=CARTESIAN_POINT ( 'NONE',  ( -27.16883889988623935, 55.32500000273120122, 19.73931689729374739 ) ) ;
#11646=CARTESIAN_POINT ( 'NONE',  ( 27.16883889988624290, 25.92500000273119554, 19.73931689729373673 ) ) ;
#11651=CARTESIAN_POINT ( 'NONE',  ( -20.08610463437157989, 48.20000000546237828, -27.64615127144129758 ) ) ;
#11657=CARTESIAN_POINT ( 'NONE',  ( -2.162160676586881955E-15, 76.62500000273118417, -35.31076352940723240 ) ) ;
#11662=CARTESIAN_POINT ( 'NONE',  ( 6.277390505771533514E-15, 9.000000005462378994, 34.17252228774368916 ) ) ;
#11672=CARTESIAN_POINT ( 'NONE',  ( 20.08610463437157279, 35.29999999999999716, -27.64615127144129758 ) ) ;
#11680=ORIENTED_EDGE ( 'NONE', *, *, #21696, .T. ) ;
#11684=CARTESIAN_POINT ( 'NONE',  ( 10.37757302488624056, 48.52500000273117564, -31.93888565452638417 ) ) ;
#11685=CARTESIAN_POINT ( 'NONE',  ( 6.486482029760649416E-15, 7.875000002731177950, 35.31076352940723240 ) ) ;
#11686=CARTESIAN_POINT ( 'NONE',  ( -2.162160676586882350E-15, 62.87500000273120548, -35.31076352940722529 ) ) ;
#11690=CARTESIAN_POINT ( 'NONE',  ( 26.29305231718579350, 69.30000000546236549, 19.10302069950537529 ) ) ;
#11696=CARTESIAN_POINT ( 'NONE',  ( 6.486482029760649416E-15, 43.87500000273118417, 35.31076352940723240 ) ) ;
#11698=CARTESIAN_POINT ( 'NONE',  ( -32.50000000000000000, 30.50000000546236478, 0.000000000000000000 ) ) ;
#11715=CARTESIAN_POINT ( 'NONE',  ( -26.29305231718579350, 55.80000000000000426, -19.10302069950537884 ) ) ;
#11717=CARTESIAN_POINT ( 'NONE',  ( 6.277390505771533514E-15, 6.499999999999998224, 34.17252228774368916 ) ) ;
#11722=CARTESIAN_POINT ( 'NONE',  ( -20.75514604977248112, 65.42500000273118133, 28.56700777964554661 ) ) ;
#11723=CARTESIAN_POINT ( 'NONE',  ( -27.16883889988624290, 29.17500000273119554, -19.73931689729374028 ) ) ;
#11725=CARTESIAN_POINT ( 'NONE',  ( 6.486482029760649416E-15, 13.87500000273117529, 35.31076352940723240 ) ) ;
#11732=CARTESIAN_POINT ( 'NONE',  ( -20.08610463437157989, 49.70000000000000284, -27.64615127144129758 ) ) ;
#11738=CARTESIAN_POINT ( 'NONE',  ( -10.37757302488624411, 60.97500000273119269, -31.93888565452638417 ) ) ;
#11742=VERTEX_POINT ( 'NONE', #22610 ) ;
#11743=CARTESIAN_POINT ( 'NONE',  ( 27.16883889988623935, 30.32500000273117990, -19.73931689729374384 ) ) ;
#11765=CARTESIAN_POINT ( 'NONE',  ( -33.58253175000000113, 49.27500000273118985, -10.91162601494193218 ) ) ;
#11770=STYLED_ITEM ( 'NONE', ( #10657 ), #32129 ) ;
#11774=CARTESIAN_POINT ( 'NONE',  ( 32.50000000000000711, 64.89999999999997726, 10.55989012756945122 ) ) ;
#11779=CARTESIAN_POINT ( 'NONE',  ( 20.75514604977248467, 76.67500000273116711, -28.56700777964554305 ) ) ;
#11784=CARTESIAN_POINT ( 'NONE',  ( 20.75514604977248467, 58.42500000273119554, -28.56700777964554305 ) ) ;
#11785=CARTESIAN_POINT ( 'NONE',  ( -20.75514604977248823, 29.07500000273119056, -28.56700777964554305 ) ) ;
#11790=CARTESIAN_POINT ( 'NONE',  ( -20.75514604977248112, 1.425000002731191984, 28.56700777964554661 ) ) ;
#11794=AXIS2_PLACEMENT_3D ( 'NONE', #3405, #19691, #11458 ) ;
#11801=CARTESIAN_POINT ( 'NONE',  ( 33.58253175000000113, 58.12500000273116996, -4.112674001490185761E-15 ) ) ;
#11818=CARTESIAN_POINT ( 'NONE',  ( 33.58253175000000823, 20.02500000273118275, 10.91162601494192863 ) ) ;
#11820=CARTESIAN_POINT ( 'NONE',  ( 1.093617666956751375E-13, 61.50000000000000711, -32.50000000000000711 ) ) ;
#11822=CARTESIAN_POINT ( 'NONE',  ( 32.50000000000000711, 45.40000000546237402, 10.55989012756945122 ) ) ;
#11827=CARTESIAN_POINT ( 'NONE',  ( 27.16883889988624290, 77.92500000273118133, 19.73931689729373673 ) ) ;
#11832=CARTESIAN_POINT ( 'NONE',  ( 20.08610463437157279, 13.80000000546235839, -27.64615127144129758 ) ) ;
#11841=CARTESIAN_POINT ( 'NONE',  ( -2.092463501923844636E-15, 33.50000000000001421, -34.17252228774368916 ) ) ;
#11853=CARTESIAN_POINT ( 'NONE',  ( -20.75514604977248112, 47.42500000273118843, 28.56700777964554661 ) ) ;
#11854=CARTESIAN_POINT ( 'NONE',  ( 6.486482029760649416E-15, 3.875000002731187720, 35.31076352940723240 ) ) ;
#11855=CARTESIAN_POINT ( 'NONE',  ( 27.16883889988623935, 54.57500000273117280, -19.73931689729374384 ) ) ;
#11860=CARTESIAN_POINT ( 'NONE',  ( -26.29305231718579350, 66.30000000546236549, -19.10302069950537884 ) ) ;
#11867=CARTESIAN_POINT ( 'NONE',  ( 27.16883889988623935, 40.57500000273118701, -19.73931689729374384 ) ) ;
#11870=CARTESIAN_POINT ( 'NONE',  ( 26.29305231718579350, 31.30000000546239036, 19.10302069950537529 ) ) ;
#11889=FACE_OUTER_BOUND ( 'NONE', #33394, .T. ) ;
#11892=CARTESIAN_POINT ( 'NONE',  ( 6.277390505771533514E-15, 2.500000000000008882, 34.17252228774368916 ) ) ;
#11897=CARTESIAN_POINT ( 'NONE',  ( -33.58253175000000113, 65.02500000273118985, -10.91162601494193218 ) ) ;
#11898=CARTESIAN_POINT ( 'NONE',  ( 33.58253175000000113, 26.37500000273117351, -4.112674001490185761E-15 ) ) ;
#11899=CARTESIAN_POINT ( 'NONE',  ( 27.16883889988623935, 16.57500000273119767, -19.73931689729374384 ) ) ;
#11904=CARTESIAN_POINT ( 'NONE',  ( 32.50000000000000000, 45.10000000000000853, -10.55989012756945833 ) ) ;
#11909=CARTESIAN_POINT ( 'NONE',  ( -10.37757302488623701, 59.77500000273121117, 31.93888565452638417 ) ) ;
#11915=CARTESIAN_POINT ( 'NONE',  ( 10.37757302488624767, 27.72500000273118914, 31.93888565452638417 ) ) ;
#11938=CARTESIAN_POINT ( 'NONE',  ( 33.58253175000000113, 44.47500000273119269, -10.91162601494193751 ) ) ;
#11943=CARTESIAN_POINT ( 'NONE',  ( 26.29305231718578995, 69.20000000000000284, -19.10302069950538240 ) ) ;
#11952=CARTESIAN_POINT ( 'NONE',  ( -33.58253175000000113, 51.22500000273119269, 10.91162601494193929 ) ) ;
#11953=CARTESIAN_POINT ( 'NONE',  ( 27.16883889988624290, 24.17500000273119198, 19.73931689729373673 ) ) ;
#11967=CARTESIAN_POINT ( 'NONE',  ( 27.16883889988624290, 53.92500000273118843, 19.73931689729373673 ) ) ;
#11979=DIRECTION ( 'NONE',  ( 0.000000000000000000, 1.000000000000000000, 0.000000000000000000 ) ) ;
#11983=CARTESIAN_POINT ( 'NONE',  ( 20.75514604977248467, 24.42500000273119554, -28.56700777964554305 ) ) ;
#11987=CARTESIAN_POINT ( 'NONE',  ( 32.50000000000000000, 39.50000000546237544, -3.980102097228898626E-15 ) ) ;
#11993=CARTESIAN_POINT ( 'NONE',  ( 20.75514604977249178, 65.82500000273115859, 28.56700777964553950 ) ) ;
#11999=CARTESIAN_POINT ( 'NONE',  ( -32.50000000000000000, 8.600000005462376862, 10.55989012756946366 ) ) ;
#12009=CARTESIAN_POINT ( 'NONE',  ( -26.29305231718578995, 38.19999999999999574, 19.10302069950538595 ) ) ;
#12022=CARTESIAN_POINT ( 'NONE',  ( -33.58253175000000113, 43.02500000273118275, -10.91162601494193218 ) ) ;
#12023=CARTESIAN_POINT ( 'NONE',  ( 33.58253175000000823, 4.275000002731189852, 10.91162601494192863 ) ) ;
#12024=CARTESIAN_POINT ( 'NONE',  ( -33.58253175000000113, 55.27500000273121117, -10.91162601494193041 ) ) ;
#12028=CARTESIAN_POINT ( 'NONE',  ( -2.092463501923844636E-15, 58.00000000546235412, -34.17252228774368916 ) ) ;
#12033=CARTESIAN_POINT ( 'NONE',  ( 20.75514604977248467, 40.67500000273116711, -28.56700777964554305 ) ) ;
#12036=CARTESIAN_POINT ( 'NONE',  ( -2.092463501923844636E-15, 30.00000000546236478, -34.17252228774368916 ) ) ;
#12047=CARTESIAN_POINT ( 'NONE',  ( -33.58253175000000113, 65.22500000273117848, 10.91162601494193929 ) ) ;
#12057=CARTESIAN_POINT ( 'NONE',  ( 20.08610463437158344, 4.699999999999995737, 27.64615127144129403 ) ) ;
#12062=CARTESIAN_POINT ( 'NONE',  ( 20.75514604977248467, 62.42500000273118133, -28.56700777964554305 ) ) ;
#12063=CARTESIAN_POINT ( 'NONE',  ( -10.37757302488624411, 24.97500000273118914, -31.93888565452638417 ) ) ;
#12064=CARTESIAN_POINT ( 'NONE',  ( -33.58253175000000113, 11.27500000273118630, -10.91162601494193218 ) ) ;
#12067=EDGE_CURVE ( 'NONE', #679, #4618, #17292, .T. ) ;
#12070=CARTESIAN_POINT ( 'NONE',  ( 32.50000000000000000, 45.00000000000000000, -3.980102097228898626E-15 ) ) ;
#12076=CARTESIAN_POINT ( 'NONE',  ( -33.58253175000000113, 59.37500000273119838, 0.000000000000000000 ) ) ;
#12081=CARTESIAN_POINT ( 'NONE',  ( -20.75514604977248112, 27.42500000273118488, 28.56700777964554661 ) ) ;
#12103=CARTESIAN_POINT ( 'NONE',  ( -20.75514604977248823, 43.07500000273118701, -28.56700777964554305 ) ) ;
#12108=CARTESIAN_POINT ( 'NONE',  ( -20.08610463437156923, 68.30000000000001137, 27.64615127144130113 ) ) ;
#12118=CARTESIAN_POINT ( 'NONE',  ( 10.37757302488624056, 52.52500000273117564, -31.93888565452638417 ) ) ;
#12119=CARTESIAN_POINT ( 'NONE',  ( 20.75514604977249178, 20.07500000273118346, 28.56700777964553950 ) ) ;
#12124=LINE ( 'NONE', #2168, #7963 ) ;
#12142=CARTESIAN_POINT ( 'NONE',  ( -10.37757302488623701, 59.77500000273121117, 31.93888565452638417 ) ) ;
#12145=CARTESIAN_POINT ( 'NONE',  ( 1.076200423132605543E-16, 52.00000000000000711, -46.18802153517007980 ) ) ;
#12146=LINE ( 'NONE', #14564, #28923 ) ;
#12150=CARTESIAN_POINT ( 'NONE',  ( 10.37757302488624767, 19.72500000273118204, 31.93888565452638417 ) ) ;
#12155=CARTESIAN_POINT ( 'NONE',  ( -32.50000000000000000, 44.40000000546238823, -10.55989012756945478 ) ) ;
#12156=ADVANCED_FACE ( 'NONE', ( #11889 ), #33153, .F. ) ;
#12163=CARTESIAN_POINT ( 'NONE',  ( 10.37757302488624767, 69.72500000273117848, 31.93888565452638417 ) ) ;
#12169=CARTESIAN_POINT ( 'NONE',  ( 33.58253175000000113, 12.22500000273118381, -10.91162601494193751 ) ) ;
#12181=CARTESIAN_POINT ( 'NONE',  ( 32.50000000000000000, 34.99999999999999289, -3.980102097228898626E-15 ) ) ;
#12185=CARTESIAN_POINT ( 'NONE',  ( -10.64935084019668743, 66.99999999999997158, 30.92824909085704377 ) ) ;
#12195=CARTESIAN_POINT ( 'NONE',  ( -33.58253175000000113, 41.12500000273118417, 0.000000000000000000 ) ) ;
#12196=CARTESIAN_POINT ( 'NONE',  ( -33.58253175000000113, 3.475000002731185589, 10.91162601494193929 ) ) ;
#12197=CARTESIAN_POINT ( 'NONE',  ( 20.75514604977249178, 56.07500000273117990, 28.56700777964553950 ) ) ;
#12200=CARTESIAN_POINT ( 'NONE',  ( -10.04305231718578462, 62.90000000546238113, 30.90933677959249337 ) ) ;
#12207=CARTESIAN_POINT ( 'NONE',  ( -20.75514604977248823, 43.07500000273118701, -28.56700777964554305 ) ) ;
#12211=CARTESIAN_POINT ( 'NONE',  ( 26.29305231718578995, 29.70000000546237118, -19.10302069950538240 ) ) ;
#12212=ORIENTED_EDGE ( 'NONE', *, *, #30528, .T. ) ;
#12220=CARTESIAN_POINT ( 'NONE',  ( -2.162160676586882350E-15, 64.62500000273121259, -35.31076352940722529 ) ) ;
#12230=CARTESIAN_POINT ( 'NONE',  ( 10.04305231718578817, 3.400000000000000355, -30.90933677959249337 ) ) ;
#12235=CARTESIAN_POINT ( 'NONE',  ( 33.58253175000000113, 58.22500000273116427, -10.91162601494193751 ) ) ;
#12236=CARTESIAN_POINT ( 'NONE',  ( 20.75514604977249178, 22.07500000273117990, 28.56700777964553950 ) ) ;
#12237=CARTESIAN_POINT ( 'NONE',  ( 33.58253175000000113, 10.37500000273118594, -4.112674001490185761E-15 ) ) ;
#12241=CARTESIAN_POINT ( 'NONE',  ( 6.486482029760649416E-15, 1.625000002731185944, 35.31076352940723240 ) ) ;
#12243=CARTESIAN_POINT ( 'NONE',  ( 26.29305231718579350, 40.79999999999999005, 19.10302069950537529 ) ) ;
#12249=CARTESIAN_POINT ( 'NONE',  ( -20.75514604977248112, 57.67500000273118133, 28.56700777964554661 ) ) ;
#12254=CARTESIAN_POINT ( 'NONE',  ( 6.486482029760649416E-15, 27.62500000273118062, 35.31076352940723240 ) ) ;
#12276=CARTESIAN_POINT ( 'NONE',  ( -27.16883889988624290, 78.92500000273118133, -19.73931689729374028 ) ) ;
#12277=CARTESIAN_POINT ( 'NONE',  ( 6.486482029760649416E-15, 43.87500000273118417, 35.31076352940723240 ) ) ;
#12282=CARTESIAN_POINT ( 'NONE',  ( 10.04305231718578817, 63.39999999999999858, -30.90933677959249337 ) ) ;
#12288=DIRECTION ( 'NONE',  ( 0.000000000000000000, 1.000000000000000000, 0.000000000000000000 ) ) ;
#12294=CARTESIAN_POINT ( 'NONE',  ( 27.16883889988624290, 49.92500000273118843, 19.73931689729373673 ) ) ;
#12295=CARTESIAN_POINT ( 'NONE',  ( -2.162160676586881955E-15, 20.87500000273119127, -35.31076352940723240 ) ) ;
#12321=CARTESIAN_POINT ( 'NONE',  ( -27.16883889988624290, 59.17500000273119554, -19.73931689729374028 ) ) ;
#12325=PLANE ( 'NONE',  #26750 ) ;
#12329=CARTESIAN_POINT ( 'NONE',  ( -27.16883889988623935, 21.32500000273117280, 19.73931689729374739 ) ) ;
#12331=CARTESIAN_POINT ( 'NONE',  ( -40.00000000000000711, 66.99999999999998579, 23.09401076758504345 ) ) ;
#12334=CARTESIAN_POINT ( 'NONE',  ( -10.04305231718578462, 44.90000000546238823, 30.90933677959249337 ) ) ;
#12339=CARTESIAN_POINT ( 'NONE',  ( -27.16883889988623935, 71.32500000273118701, 19.73931689729374739 ) ) ;
#12346=CARTESIAN_POINT ( 'NONE',  ( 20.75514604977249178, 13.82500000273117813, 28.56700777964553950 ) ) ;
#12355=CARTESIAN_POINT ( 'NONE',  ( 20.08610463437157279, 27.29999999999997939, -27.64615127144129758 ) ) ;
#12360=CARTESIAN_POINT ( 'NONE',  ( 26.29305231718579350, 62.80000000000001137, 19.10302069950537529 ) ) ;
#12369=CARTESIAN_POINT ( 'NONE',  ( -20.75514604977248112, 41.42500000273118133, 28.56700777964554661 ) ) ;
#12370=CARTESIAN_POINT ( 'NONE',  ( -33.58253175000000113, 7.475000002731190030, 10.91162601494193929 ) ) ;
#12371=CARTESIAN_POINT ( 'NONE',  ( -33.58253175000000113, 57.27500000273120406, -10.91162601494193041 ) ) ;
#12375=CARTESIAN_POINT ( 'NONE',  ( 32.50000000000000000, 59.50000000546238965, -3.980102097228898626E-15 ) ) ;
#12383=CARTESIAN_POINT ( 'NONE',  ( -20.75514604977248823, 35.07500000273120833, -28.56700777964554305 ) ) ;
#12387=CARTESIAN_POINT ( 'NONE',  ( 10.04305231718579705, 25.10000000546237686, 30.90933677959248982 ) ) ;
#12407=CARTESIAN_POINT ( 'NONE',  ( 10.04305231718579705, 4.599999999999992539, 30.90933677959248982 ) ) ;
#12412=CARTESIAN_POINT ( 'NONE',  ( 10.37757302488624056, 62.52500000273118985, -31.93888565452638417 ) ) ;
#12413=CARTESIAN_POINT ( 'NONE',  ( -33.58253175000000113, 21.27500000273117209, -10.91162601494193218 ) ) ;
#12414=CARTESIAN_POINT ( 'NONE',  ( 6.486482029760649416E-15, 11.87500000273118062, 35.31076352940723240 ) ) ;
#12419=CARTESIAN_POINT ( 'NONE',  ( -32.50000000000000000, 78.40000000546233139, -10.55989012756945478 ) ) ;
#12421=CARTESIAN_POINT ( 'NONE',  ( 6.277390505771533514E-15, 40.50000000000000711, 34.17252228774368916 ) ) ;
#12426=CARTESIAN_POINT ( 'NONE',  ( -2.162160676586881955E-15, 58.87500000273117706, -35.31076352940723240 ) ) ;
#12432=CARTESIAN_POINT ( 'NONE',  ( 27.16883889988624290, 31.92500000273119909, 19.73931689729373673 ) ) ;
#12453=CARTESIAN_POINT ( 'NONE',  ( 27.16883889988623935, 78.32500000273120122, -19.73931689729374384 ) ) ;
#12454=CARTESIAN_POINT ( 'NONE',  ( 27.16883889988623935, 42.57500000273119412, -19.73931689729374384 ) ) ;
#12459=CARTESIAN_POINT ( 'NONE',  ( -26.29305231718579350, 61.80000000000000426, -19.10302069950537884 ) ) ;
#12469=CARTESIAN_POINT ( 'NONE',  ( -27.16883889988624290, 48.92500000273118843, -19.73931689729374028 ) ) ;
#12470=CARTESIAN_POINT ( 'NONE',  ( 10.37757302488624767, 21.97500000273118559, 31.93888565452638417 ) ) ;
#12471=ORIENTED_EDGE ( 'NONE', *, *, #30528, .F. ) ;
#12474=DIRECTION ( 'NONE',  ( 0.000000000000000000, 1.000000000000000000, 0.000000000000000000 ) ) ;
#12483=CARTESIAN_POINT ( 'NONE',  ( -20.52662985655310379, 67.00000000000000000, -26.66963712870534664 ) ) ;
#12494=CARTESIAN_POINT ( 'NONE',  ( -10.37757302488624411, 64.97500000273119269, -31.93888565452638417 ) ) ;
#12500=CARTESIAN_POINT ( 'NONE',  ( 10.04305231718578817, 63.90000000546238113, -30.90933677959249337 ) ) ;
#12501=CARTESIAN_POINT ( 'NONE',  ( -20.08610463437157989, 77.70000000000003126, -27.64615127144129758 ) ) ;
#12502=CARTESIAN_POINT ( 'NONE',  ( -27.16883889988624290, 22.92500000273119198, -19.73931689729374028 ) ) ;
#12504=CARTESIAN_POINT ( 'NONE',  ( 10.04305231718578817, 55.90000000546240244, -30.90933677959249337 ) ) ;
#12508=CARTESIAN_POINT ( 'NONE',  ( -26.29305231718578995, 38.70000000546237828, 19.10302069950538595 ) ) ;
#12514=CARTESIAN_POINT ( 'NONE',  ( 27.16883889988624290, 69.92500000273120975, 19.73931689729373673 ) ) ;
#12520=CARTESIAN_POINT ( 'NONE',  ( -27.16883889988623935, 11.32500000273119234, 19.73931689729374739 ) ) ;
#12530=CARTESIAN_POINT ( 'NONE',  ( 32.50000000000000711, 28.89999999999998792, 10.55989012756945122 ) ) ;
#12543=CARTESIAN_POINT ( 'NONE',  ( 33.58253175000000113, 40.22500000273119269, -10.91162601494193751 ) ) ;
#12544=CARTESIAN_POINT ( 'NONE',  ( -5.147494310547430452, 64.05125428700922896, -32.49999999999999289 ) ) ;
#12545=CARTESIAN_POINT ( 'NONE',  ( 20.75514604977249178, 54.07500000273118701, 28.56700777964553950 ) ) ;
#12549=CARTESIAN_POINT ( 'NONE',  ( 20.08610463437157279, 57.80000000546236549, -27.64615127144129758 ) ) ;
#12556=CARTESIAN_POINT ( 'NONE',  ( -33.58253175000000113, 35.47500000273118559, 10.91162601494193929 ) ) ;
#12560=CARTESIAN_POINT ( 'NONE',  ( -10.04305231718579172, 24.10000000546237686, -30.90933677959248982 ) ) ;
#12577=CARTESIAN_POINT ( 'NONE',  ( 31.04172217648528687, 52.00000000000000711, 12.81397374188273908 ) ) ;
#12578=CARTESIAN_POINT ( 'NONE',  ( 6.486482029760649416E-15, 73.87500000273119838, 35.31076352940723240 ) ) ;
#12583=CARTESIAN_POINT ( 'NONE',  ( 33.58253175000000823, 62.02500000273116143, 10.91162601494192863 ) ) ;
#12584=CARTESIAN_POINT ( 'NONE',  ( 33.58253175000000113, 22.47500000273119625, -10.91162601494193751 ) ) ;
#12585=CARTESIAN_POINT ( 'NONE',  ( 27.16883889988624290, 12.17500000273118133, 19.73931689729373673 ) ) ;
#12589=CARTESIAN_POINT ( 'NONE',  ( -27.16883889988623935, 3.325000002731184789, 19.73931689729374739 ) ) ;
#12591=CARTESIAN_POINT ( 'NONE',  ( -32.50000000000000000, 40.09999999999998721, 10.55989012756946366 ) ) ;
#12597=CARTESIAN_POINT ( 'NONE',  ( -33.58253175000000113, 55.47500000273119980, 10.91162601494193929 ) ) ;
#12602=EDGE_LOOP ( 'NONE', ( #27155, #2083, #12681, #9855, #2517, #28469 ) ) ;
#12603=CARTESIAN_POINT ( 'NONE',  ( -33.58253175000000113, 21.02500000273117919, -10.91162601494193218 ) ) ;
#12615=CARTESIAN_POINT ( 'NONE',  ( 26.29305231718578995, 65.70000000546237118, -19.10302069950538240 ) ) ;
#12616=CARTESIAN_POINT ( 'NONE',  ( 10.04305231718578817, 55.39999999999999147, -30.90933677959249337 ) ) ;
#12617=CARTESIAN_POINT ( 'NONE',  ( -32.50000000000000000, 52.00000000000000711, 0.000000000000000000 ) ) ;
#12622=CARTESIAN_POINT ( 'NONE',  ( 10.37757302488624767, 77.72500000273117848, 31.93888565452638417 ) ) ;
#12623=CARTESIAN_POINT ( 'NONE',  ( -2.162160676586881955E-15, 42.87500000273119127, -35.31076352940723240 ) ) ;
#12628=CARTESIAN_POINT ( 'NONE',  ( -10.04305231718579172, 61.60000000000000142, -30.90933677959248982 ) ) ;
#12632=CARTESIAN_POINT ( 'NONE',  ( -2.162160676586881955E-15, 72.87500000273115575, -35.31076352940723240 ) ) ;
#12637=CARTESIAN_POINT ( 'NONE',  ( 10.37757302488624767, 47.72500000273117848, 31.93888565452638417 ) ) ;
#12641=CARTESIAN_POINT ( 'NONE',  ( -10.04305231718578462, 2.900000005462380237, 30.90933677959249337 ) ) ;
#12649=LINE ( 'NONE', #13844, #20973 ) ;
#12661=CARTESIAN_POINT ( 'NONE',  ( -27.16883889988624290, 61.17500000273119554, -19.73931689729374028 ) ) ;
#12668=CARTESIAN_POINT ( 'NONE',  ( 26.29305231718579350, 78.79999999999999716, 19.10302069950537529 ) ) ;
#12669=CARTESIAN_POINT ( 'NONE',  ( -10.37757302488623701, 13.52500000273119873, 31.93888565452638417 ) ) ;
#12674=CARTESIAN_POINT ( 'NONE',  ( -10.04305231718578462, 40.90000000546238823, 30.90933677959249337 ) ) ;
#12681=ORIENTED_EDGE ( 'NONE', *, *, #21130, .F. ) ;
#12682=CARTESIAN_POINT ( 'NONE',  ( 33.58253175000000823, 70.02500000273121827, 10.91162601494192863 ) ) ;
#12689=CARTESIAN_POINT ( 'NONE',  ( -33.58253175000000113, 9.225000002731190918, 10.91162601494193929 ) ) ;
#12697=CARTESIAN_POINT ( 'NONE',  ( -20.08610463437157989, 52.20000000546236407, -27.64615127144129758 ) ) ;
#12699=CARTESIAN_POINT ( 'NONE',  ( -32.50000000000000000, 32.00000000000001421, 0.000000000000000000 ) ) ;
#12712=CARTESIAN_POINT ( 'NONE',  ( -20.75514604977248823, 40.82500000273120122, -28.56700777964554305 ) ) ;
#12713=CARTESIAN_POINT ( 'NONE',  ( -1.778240108872766143E-15, 64.00000000546238255, -32.49999999999999289 ) ) ;
#12716=DIRECTION ( 'NONE',  ( 0.8660254037844387076, 0.000000000000000000, -0.4999999999999998890 ) ) ;
#12718=CARTESIAN_POINT ( 'NONE',  ( -2.092463501923844636E-15, 64.00000000546236834, -34.17252228774368916 ) ) ;
#12726=CARTESIAN_POINT ( 'NONE',  ( -10.37757302488624411, 34.97500000273119980, -31.93888565452638417 ) ) ;
#12730=CARTESIAN_POINT ( 'NONE',  ( -2.092463501923844636E-15, 24.00000000546238610, -34.17252228774368916 ) ) ;
#12741=CARTESIAN_POINT ( 'NONE',  ( 20.75514604977248467, 58.42500000273119554, -28.56700777964554305 ) ) ;
#12751=CARTESIAN_POINT ( 'NONE',  ( 25.33181144634140836, 52.00000000000002842, 22.15645287102023175 ) ) ;
#12753=CARTESIAN_POINT ( 'NONE',  ( 20.75514604977249178, 72.07500000273120122, 28.56700777964553950 ) ) ;
#12758=CARTESIAN_POINT ( 'NONE',  ( 20.75514604977248467, 58.42500000273119554, -28.56700777964554305 ) ) ;
#12759=CARTESIAN_POINT ( 'NONE',  ( -33.58253175000000113, 19.47500000273117493, 10.91162601494193929 ) ) ;
#12760=CARTESIAN_POINT ( 'NONE',  ( 27.16883889988624290, 10.17500000273117955, 19.73931689729373673 ) ) ;
#12764=CARTESIAN_POINT ( 'NONE',  ( -10.37757302488623701, 3.525000002731190740, 31.93888565452638417 ) ) ;
#12766=CARTESIAN_POINT ( 'NONE',  ( -32.50000000000000000, 44.10000000000000142, 10.55989012756946366 ) ) ;
#12771=CARTESIAN_POINT ( 'NONE',  ( -20.75514604977248112, 51.67500000273117422, 28.56700777964554661 ) ) ;
#12772=CARTESIAN_POINT ( 'NONE',  ( 32.50000000000000000, 59.50000000546238965, -3.980102097228898626E-15 ) ) ;
#12775=ORIENTED_EDGE ( 'NONE', *, *, #32213, .T. ) ;
#12776=CARTESIAN_POINT ( 'NONE',  ( -27.16883889988624290, 26.92500000273119554, -19.73931689729374028 ) ) ;
#12779=ORIENTED_EDGE ( 'NONE', *, *, #22119, .F. ) ;
#12791=CARTESIAN_POINT ( 'NONE',  ( -26.29305231718579350, 15.79999999999999538, -19.10302069950537884 ) ) ;
#12798=CARTESIAN_POINT ( 'NONE',  ( -20.75514604977248112, 35.67500000273118843, 28.56700777964554661 ) ) ;
#12800=EDGE_CURVE ( 'NONE', #2261, #25651, #633, .T. ) ;
#12804=CARTESIAN_POINT ( 'NONE',  ( 20.08610463437157279, 59.30000000000001847, -27.64615127144129758 ) ) ;
#12808=CARTESIAN_POINT ( 'NONE',  ( -2.162160676586881955E-15, 70.87500000273118417, -35.31076352940723240 ) ) ;
#12813=CARTESIAN_POINT ( 'NONE',  ( -27.16883889988624290, 42.92500000273118133, -19.73931689729374028 ) ) ;
#12817=CARTESIAN_POINT ( 'NONE',  ( 26.29305231718578995, 3.700000005462375618, -19.10302069950538240 ) ) ;
#12838=CARTESIAN_POINT ( 'NONE',  ( 33.58253175000000823, 62.27500000273118275, 10.91162601494192863 ) ) ;
#12844=CARTESIAN_POINT ( 'NONE',  ( -32.50000000000000000, 80.00000000000000000, 0.000000000000000000 ) ) ;
#12845=CARTESIAN_POINT ( 'NONE',  ( 10.37757302488624056, 18.52500000273120406, -31.93888565452638417 ) ) ;
#12850=CARTESIAN_POINT ( 'NONE',  ( -32.50000000000000000, 36.50000000546236834, 0.000000000000000000 ) ) ;
#12855=CARTESIAN_POINT ( 'NONE',  ( -10.37757302488623701, 59.52500000273118275, 31.93888565452638417 ) ) ;
#12860=CARTESIAN_POINT ( 'NONE',  ( 33.58253175000000823, 14.02500000273117209, 10.91162601494192863 ) ) ;
#12871=CARTESIAN_POINT ( 'NONE',  ( 6.277390505771533514E-15, 28.50000000000000000, 34.17252228774368916 ) ) ;
#12875=CARTESIAN_POINT ( 'NONE',  ( -31.95463953835047377, 66.99999999999998579, -10.27070314127411521 ) ) ;
#12882=CARTESIAN_POINT ( 'NONE',  ( 18.68038058909793619, 66.99999999999997158, -27.25458793344660080 ) ) ;
#12883=CARTESIAN_POINT ( 'NONE',  ( 20.75514604977249178, 33.82500000273117990, 28.56700777964553950 ) ) ;
#12884=LINE ( 'NONE', #23360, #21547 ) ;
#12888=CARTESIAN_POINT ( 'NONE',  ( -32.50000000000000000, 56.60000000546236976, 10.55989012756946366 ) ) ;
#12889=VECTOR ( 'NONE', #27106, 1000.000000000000000 ) ;
#12896=CARTESIAN_POINT ( 'NONE',  ( -20.75514604977248112, 37.67500000273118133, 28.56700777964554661 ) ) ;
#12900=CARTESIAN_POINT ( 'NONE',  ( 32.50000000000000711, 21.40000000546237757, 10.55989012756945122 ) ) ;
#12905=VECTOR ( 'NONE', #6413, 1000.000000000000000 ) ;
#12911=CARTESIAN_POINT ( 'NONE',  ( 33.58253175000000113, 58.22500000273117138, -10.91162601494193574 ) ) ;
#12919=LINE ( 'NONE', #18592, #26993 ) ;
#12920=CARTESIAN_POINT ( 'NONE',  ( 20.75514604977248467, 76.67500000273116711, -28.56700777964554305 ) ) ;
#12925=CARTESIAN_POINT ( 'NONE',  ( -33.58253175000000113, 53.22500000273118559, 10.91162601494193929 ) ) ;
#12926=CARTESIAN_POINT ( 'NONE',  ( -2.162160676586881955E-15, 18.87500000273119483, -35.31076352940723240 ) ) ;
#12927=CARTESIAN_POINT ( 'NONE',  ( -10.37757302488624411, 2.975000002731182036, -31.93888565452638417 ) ) ;
#12932=CARTESIAN_POINT ( 'NONE',  ( 32.50000000000000000, 77.50000000546238255, -3.980102097228898626E-15 ) ) ;
#12933=CARTESIAN_POINT ( 'NONE',  ( 23.28634348215027572, 51.99999999999997868, -23.32808161240107125 ) ) ;
#12940=CARTESIAN_POINT ( 'NONE',  ( -20.75514604977248823, 53.07500000273118701, -28.56700777964554305 ) ) ;
#12945=CARTESIAN_POINT ( 'NONE',  ( 27.16883889988623935, 26.32500000273117635, -19.73931689729374384 ) ) ;
#12961=CARTESIAN_POINT ( 'NONE',  ( -10.04305231718579172, 19.59999999999999076, -30.90933677959248982 ) ) ;
#12968=CARTESIAN_POINT ( 'NONE',  ( 10.37757302488624767, 33.97500000273119269, 31.93888565452638417 ) ) ;
#12974=CARTESIAN_POINT ( 'NONE',  ( 10.04305231718579705, 58.60000000000000142, 30.90933677959248982 ) ) ;
#12979=CARTESIAN_POINT ( 'NONE',  ( -33.58253175000000113, 71.37500000273121259, 0.000000000000000000 ) ) ;
#12985=CARTESIAN_POINT ( 'NONE',  ( -33.58253175000000113, 43.22500000273118559, 10.91162601494193929 ) ) ;
#12991=CARTESIAN_POINT ( 'NONE',  ( 26.29305231718579350, 3.300000005462377928, 19.10302069950537529 ) ) ;
#13009=CARTESIAN_POINT ( 'NONE',  ( -33.58253175000000113, 53.37500000273119838, 0.000000000000000000 ) ) ;
#13017=CARTESIAN_POINT ( 'NONE',  ( 27.16883889988623935, 18.32500000273119767, -19.73931689729374384 ) ) ;
#13022=CARTESIAN_POINT ( 'NONE',  ( 10.04305231718578817, 37.90000000546238113, -30.90933677959249337 ) ) ;
#13027=CARTESIAN_POINT ( 'NONE',  ( -27.16883889988624290, 60.92500000273119554, -19.73931689729374028 ) ) ;
#13034=CARTESIAN_POINT ( 'NONE',  ( 20.75514604977249178, 5.825000002731183457, 28.56700777964553950 ) ) ;
#13043=CARTESIAN_POINT ( 'NONE',  ( 10.04305231718579705, 28.60000000000000142, 30.90933677959248982 ) ) ;
#13054=CARTESIAN_POINT ( 'NONE',  ( 33.58253175000000823, 32.02500000273118275, 10.91162601494192863 ) ) ;
#13055=CARTESIAN_POINT ( 'NONE',  ( -32.50000000000000000, 64.50000000546239676, 0.000000000000000000 ) ) ;
#13059=CARTESIAN_POINT ( 'NONE',  ( 20.08610463437158344, 55.20000000546238539, 27.64615127144129403 ) ) ;
#13065=CARTESIAN_POINT ( 'NONE',  ( 33.58253175000000823, 34.27500000273116854, 10.91162601494192863 ) ) ;
#13069=CARTESIAN_POINT ( 'NONE',  ( -32.50000000000000000, 20.50000000546238610, 0.000000000000000000 ) ) ;
#13081=CARTESIAN_POINT ( 'NONE',  ( 10.37757302488624767, 63.72500000273119269, 31.93888565452638417 ) ) ;
#13086=CARTESIAN_POINT ( 'NONE',  ( -20.08610463437156923, 66.80000000546236549, 27.64615127144130113 ) ) ;
#13091=CARTESIAN_POINT ( 'NONE',  ( -20.75514604977248112, 75.67500000273118133, 28.56700777964554661 ) ) ;
#13096=CARTESIAN_POINT ( 'NONE',  ( 10.37757302488624056, 56.52500000273118275, -31.93888565452638417 ) ) ;
#13097=CARTESIAN_POINT ( 'NONE',  ( 10.37757302488624767, 17.97500000273118204, 31.93888565452638417 ) ) ;
#13098=CARTESIAN_POINT ( 'NONE',  ( 27.16883889988624290, 2.175000002731186655, 19.73931689729373673 ) ) ;
#13102=CARTESIAN_POINT ( 'NONE',  ( 32.50000000000000000, 73.60000000546240528, -10.55989012756945833 ) ) ;
#13103=CARTESIAN_POINT ( 'NONE',  ( 9.358181289160048877, 51.99999999999999289, -31.32043657353322885 ) ) ;
#13108=VERTEX_POINT ( 'NONE', #25878 ) ;
#13109=CARTESIAN_POINT ( 'NONE',  ( 33.58253175000000113, 56.37500000273119838, -4.112674001490185761E-15 ) ) ;
#13114=CARTESIAN_POINT ( 'NONE',  ( -33.58253175000000113, 27.12500000273120193, 0.000000000000000000 ) ) ;
#13117=CARTESIAN_POINT ( 'NONE',  ( -32.50000000000000000, 58.10000000000000142, 10.55989012756946366 ) ) ;
#13126=CARTESIAN_POINT ( 'NONE',  ( -10.04305231718579172, 59.60000000000000142, -30.90933677959248982 ) ) ;
#13127=CARTESIAN_POINT ( 'NONE',  ( -20.08610463437157989, 13.70000000000000462, -27.64615127144129758 ) ) ;
#13133=CARTESIAN_POINT ( 'NONE',  ( 33.58253175000000113, 70.22500000273120691, -10.91162601494193751 ) ) ;
#13134=CARTESIAN_POINT ( 'NONE',  ( -20.75514604977248823, 35.07500000273120833, -28.56700777964554305 ) ) ;
#13141=CARTESIAN_POINT ( 'NONE',  ( -2.092463501923844636E-15, 55.49999999999999289, -34.17252228774368916 ) ) ;
#13146=CARTESIAN_POINT ( 'NONE',  ( -20.75514604977248112, 73.67500000273120975, 28.56700777964554661 ) ) ;
#13150=ORIENTED_EDGE ( 'NONE', *, *, #18466, .T. ) ;
#13151=CARTESIAN_POINT ( 'NONE',  ( -27.16883889988624290, 40.92500000273118133, -19.73931689729374028 ) ) ;
#13152=EDGE_LOOP ( 'NONE', ( #13150, #12775, #19991, #8207, #24047, #10287 ) ) ;
#13155=CARTESIAN_POINT ( 'NONE',  ( -26.29305231718578995, 6.700000005462378283, 19.10302069950538595 ) ) ;
#13156=LINE ( 'NONE', #31514, #32608 ) ;
#13173=CARTESIAN_POINT ( 'NONE',  ( 33.58253175000000823, 56.27500000273116854, 10.91162601494192863 ) ) ;
#13180=CARTESIAN_POINT ( 'NONE',  ( -26.29305231718579350, 77.80000000000002558, -19.10302069950537884 ) ) ;
#13181=CARTESIAN_POINT ( 'NONE',  ( -27.16883889988623935, 17.32500000273119767, 19.73931689729374739 ) ) ;
#13186=CARTESIAN_POINT ( 'NONE',  ( 32.50000000000000000, 35.60000000546236976, -10.55989012756945833 ) ) ;
#13192=CARTESIAN_POINT ( 'NONE',  ( -10.37757302488624411, 64.72500000273119269, -31.93888565452638417 ) ) ;
#13193=EDGE_LOOP ( 'NONE', ( #20141, #18485, #21188, #13275 ) ) ;
#13196=CARTESIAN_POINT ( 'NONE',  ( 27.16883889988623935, 4.325000002731186122, -19.73931689729374384 ) ) ;
#13205=CARTESIAN_POINT ( 'NONE',  ( 32.50000000000000000, 21.10000000000000142, -10.55989012756945833 ) ) ;
#13218=CARTESIAN_POINT ( 'NONE',  ( -2.162160676586881955E-15, 34.62500000273119127, -35.31076352940723240 ) ) ;
#13221=ADVANCED_FACE ( 'NONE', ( #28286 ), #20823, .T. ) ;
#13224=CARTESIAN_POINT ( 'NONE',  ( 32.50000000000000000, 53.60000000546238397, -10.55989012756945833 ) ) ;
#13232=CARTESIAN_POINT ( 'NONE',  ( -10.37757302488624411, 28.97500000273119269, -31.93888565452638417 ) ) ;
#13236=CARTESIAN_POINT ( 'NONE',  ( -10.04305231718579172, 18.10000000546237331, -30.90933677959248982 ) ) ;
#13248=CARTESIAN_POINT ( 'NONE',  ( -20.75514604977248823, 60.82500000273120122, -28.56700777964554305 ) ) ;
#13258=CARTESIAN_POINT ( 'NONE',  ( 10.37757302488624056, 74.77500000273117564, -31.93888565452638417 ) ) ;
#13262=ADVANCED_FACE ( 'NONE', ( #31571 ), #15469, .T. ) ;
#13263=CARTESIAN_POINT ( 'NONE',  ( -10.37757302488624411, 54.72500000273118559, -31.93888565452638417 ) ) ;
#13264=CARTESIAN_POINT ( 'NONE',  ( -20.75514604977248823, 17.07500000273119056, -28.56700777964554305 ) ) ;
#13265=CARTESIAN_POINT ( 'NONE',  ( 27.16883889988624290, 6.175000002731190207, 19.73931689729373673 ) ) ;
#13269=CARTESIAN_POINT ( 'NONE',  ( 10.04305231718578817, 75.90000000546235981, -30.90933677959249337 ) ) ;
#13270=CARTESIAN_POINT ( 'NONE',  ( 28.37133278852445528, 51.99999999999997868, -17.03823453610128524 ) ) ;
#13275=ORIENTED_EDGE ( 'NONE', *, *, #22119, .T. ) ;
#13276=CARTESIAN_POINT ( 'NONE',  ( 27.16883889988623935, 44.57500000273119412, -19.73931689729374384 ) ) ;
#13281=CARTESIAN_POINT ( 'NONE',  ( -33.58253175000000113, 27.22500000273119269, 10.91162601494193929 ) ) ;
#13285=CARTESIAN_POINT ( 'NONE',  ( -26.29305231718579350, 57.80000000000000426, -19.10302069950537884 ) ) ;
#13298=CARTESIAN_POINT ( 'NONE',  ( -32.50000000000000000, 59.99999999999998579, 0.000000000000000000 ) ) ;
#13299=CARTESIAN_POINT ( 'NONE',  ( -26.29305231718578995, 16.19999999999997797, 19.10302069950538595 ) ) ;
#13305=CARTESIAN_POINT ( 'NONE',  ( 10.37757302488624767, 73.72500000273117848, 31.93888565452638417 ) ) ;
#13306=CARTESIAN_POINT ( 'NONE',  ( 33.58253175000000823, 38.27500000273118985, 10.91162601494192863 ) ) ;
#13314=CARTESIAN_POINT ( 'NONE',  ( 32.50000000000000000, 57.00000000000000711, -3.980102097228898626E-15 ) ) ;
#13320=CARTESIAN_POINT ( 'NONE',  ( 33.58253175000000823, 74.27500000273117564, 10.91162601494192863 ) ) ;
#13321=CARTESIAN_POINT ( 'NONE',  ( -5.147494310547377161, 61.55125428154684641, -32.50000000000002132 ) ) ;
#13325=CARTESIAN_POINT ( 'NONE',  ( 33.58253175000000113, 40.22500000273119269, -10.91162601494193751 ) ) ;
#13329=CARTESIAN_POINT ( 'NONE',  ( -32.50000000000000000, 60.60000000546239107, 10.55989012756946366 ) ) ;
#13330=CARTESIAN_POINT ( 'NONE',  ( 32.50000000000000711, 3.400000005462381569, 10.55989012756945122 ) ) ;
#13349=CARTESIAN_POINT ( 'NONE',  ( 33.58253175000000113, 58.37500000273119838, -4.112674001490185761E-15 ) ) ;
#13355=CARTESIAN_POINT ( 'NONE',  ( 20.08610463437157279, 73.29999999999996874, -27.64615127144129758 ) ) ;
#13356=CARTESIAN_POINT ( 'NONE',  ( 10.37757302488624767, 15.72500000273117848, 31.93888565452638417 ) ) ;
#13361=CARTESIAN_POINT ( 'NONE',  ( 6.277390505771533514E-15, 37.00000000546237544, 34.17252228774368916 ) ) ;
#13368=CARTESIAN_POINT ( 'NONE',  ( 20.75514604977248467, 62.42500000273118133, -28.56700777964554305 ) ) ;
#13369=EDGE_CURVE ( 'NONE', #21053, #1690, #2866, .T. ) ;
#13373=CARTESIAN_POINT ( 'NONE',  ( -20.75514604977248823, 2.825000002731177240, -28.56700777964554305 ) ) ;
#13382=CARTESIAN_POINT ( 'NONE',  ( -32.50000000000000000, 20.10000000000000497, 10.55989012756946366 ) ) ;
#13395=CARTESIAN_POINT ( 'NONE',  ( -25.94559702212997365, 52.00000000000000000, 20.21712673764820778 ) ) ;
#13396=PRODUCT_DEFINITION_CONTEXT ( 'detailed design', #27843, 'design' ) ;
#13397=CARTESIAN_POINT ( 'NONE',  ( 10.37757302488624767, 37.72500000273119980, 31.93888565452638417 ) ) ;
#13398=CARTESIAN_POINT ( 'NONE',  ( 32.50000000000000000, 57.00000000000000711, -3.980102097228898626E-15 ) ) ;
#13399=CARTESIAN_POINT ( 'NONE',  ( 33.58253175000000113, 52.37500000273119838, -4.112674001490185761E-15 ) ) ;
#13402=CARTESIAN_POINT ( 'NONE',  ( -32.50000000000000000, 52.40000000546239534, -10.55989012756945478 ) ) ;
#13409=CARTESIAN_POINT ( 'NONE',  ( 33.58253175000000113, 26.47500000273118559, -10.91162601494193751 ) ) ;
#13413=CARTESIAN_POINT ( 'NONE',  ( 6.277390505771533514E-15, 15.00000000546237722, 34.17252228774368916 ) ) ;
#13423=CARTESIAN_POINT ( 'NONE',  ( -33.58253175000000113, 59.22500000273119980, 10.91162601494193929 ) ) ;
#13428=CARTESIAN_POINT ( 'NONE',  ( -32.50000000000000000, 66.50000000546239676, 0.000000000000000000 ) ) ;
#13433=CARTESIAN_POINT ( 'NONE',  ( -33.58253175000000113, 67.37500000273121259, 0.000000000000000000 ) ) ;
#13439=CARTESIAN_POINT ( 'NONE',  ( -10.37757302488623701, 51.52500000273117564, 31.93888565452638417 ) ) ;
#13440=CARTESIAN_POINT ( 'NONE',  ( 6.486482029760649416E-15, 17.87500000273119838, 35.31076352940723240 ) ) ;
#13441=CARTESIAN_POINT ( 'NONE',  ( -2.162160676586881955E-15, 2.875000002731189941, -35.31076352940723240 ) ) ;
#13445=CARTESIAN_POINT ( 'NONE',  ( 26.29305231718579350, 75.30000000546236549, 19.10302069950537529 ) ) ;
#13446=CARTESIAN_POINT ( 'NONE',  ( 32.17340636219253724, 52.00000000000002842, -8.405285767817208153 ) ) ;
#13452=CARTESIAN_POINT ( 'NONE',  ( 33.58253175000000113, 50.47500000273117848, -10.91162601494193751 ) ) ;
#13458=CARTESIAN_POINT ( 'NONE',  ( -2.162160676586881955E-15, 14.62500000273118239, -35.31076352940723240 ) ) ;
#13461=EDGE_CURVE ( 'NONE', #7658, #22688, #12884, .T. ) ;
#13477=CARTESIAN_POINT ( 'NONE',  ( 26.29305231718578995, 15.20000000000000462, -19.10302069950538240 ) ) ;
#13483=CARTESIAN_POINT ( 'NONE',  ( 10.37757302488624056, 74.52500000273120406, -31.93888565452638417 ) ) ;
#13484=CARTESIAN_POINT ( 'NONE',  ( -27.16883889988624290, 35.17500000273120264, -19.73931689729374028 ) ) ;
#13489=CARTESIAN_POINT ( 'NONE',  ( 10.04305231718578817, 51.39999999999998437, -30.90933677959249337 ) ) ;
#13490=LINE ( 'NONE', #29423, #23212 ) ;
#13494=CARTESIAN_POINT ( 'NONE',  ( 10.37757302488624056, 66.77500000273118985, -31.93888565452638417 ) ) ;
#13501=CARTESIAN_POINT ( 'NONE',  ( 27.16883889988623935, 40.32500000273118701, -19.73931689729374384 ) ) ;
#13504=( BOUNDED_CURVE ( )  B_SPLINE_CURVE ( 2, ( #26870, #26370, #21396, #6097, #23629, #13329, #2859, #31842, #29595, #21564, #29098, #32009, #8504 ),
 .UNSPECIFIED., .F., .T. ) 
 B_SPLINE_CURVE_WITH_KNOTS ( ( 3, 2, 2, 2, 2, 2, 3 ),
 ( 0.2243589743589743668, 0.2256410256410256443, 0.2282051282051281993, 0.2307692307692307820, 0.2333333333333333370, 0.2358974358974358920, 0.2371794871794871973 ),
 .UNSPECIFIED. ) 
 CURVE ( )  GEOMETRIC_REPRESENTATION_ITEM ( )  RATIONAL_B_SPLINE_CURVE ( ( 0.9755282581475768211, 0.9755282581475768211, 1.000000000000000000, 0.9510565162951535312, 1.000000000000000000, 0.9510565162951535312, 1.000000000000000000, 0.9510565162951535312, 1.000000000000000000, 0.9510565162951535312, 1.000000000000000000, 0.9755282581475764880, 0.9755282581475768211 ) ) 
 REPRESENTATION_ITEM ( '' )  );
#13507=CARTESIAN_POINT ( 'NONE',  ( 20.08610463437157279, 59.30000000000001847, -27.64615127144129758 ) ) ;
#13525=CARTESIAN_POINT ( 'NONE',  ( -33.58253175000000113, 57.37500000273119838, 0.000000000000000000 ) ) ;
#13530=ADVANCED_FACE ( 'NONE', ( #10144 ), #23695, .F. ) ;
#13532=CARTESIAN_POINT ( 'NONE',  ( -32.50000000000000000, 74.00000000000000000, 0.000000000000000000 ) ) ;
#13533=CARTESIAN_POINT ( 'NONE',  ( 33.58253175000000113, 8.225000002731182036, -10.91162601494193751 ) ) ;
#13541=CARTESIAN_POINT ( 'NONE',  ( -10.37757302488623701, 65.52500000273118985, 31.93888565452638417 ) ) ;
#13545=CARTESIAN_POINT ( 'NONE',  ( 27.16883889988624290, 7.925000002731205306, 19.73931689729373673 ) ) ;
#13556=EDGE_CURVE ( 'NONE', #24301, #679, #1736, .T. ) ;
#13558=CARTESIAN_POINT ( 'NONE',  ( -26.29305231718578995, 26.19999999999998863, 19.10302069950538595 ) ) ;
#13562=CARTESIAN_POINT ( 'NONE',  ( -33.02351622650638063, 66.99999999999997158, 4.441931073548307296 ) ) ;
#13570=CARTESIAN_POINT ( 'NONE',  ( 3.724851327375194643, 52.00000000000000000, 33.24794091741933499 ) ) ;
#13571=CARTESIAN_POINT ( 'NONE',  ( 6.486482029760649416E-15, 31.62500000273119483, 35.31076352940723240 ) ) ;
#13577=CARTESIAN_POINT ( 'NONE',  ( -32.50000000000000000, 56.40000000546238113, -10.55989012756945478 ) ) ;
#13579=SURFACE_SIDE_STYLE ('',( #342 ) ) ;
#13587=CARTESIAN_POINT ( 'NONE',  ( 20.08610463437157279, 19.80000000546237260, -27.64615127144129758 ) ) ;
#13596=CARTESIAN_POINT ( 'NONE',  ( -27.16883889988624290, 56.92500000273119554, -19.73931689729374028 ) ) ;
#13606=CARTESIAN_POINT ( 'NONE',  ( -33.58253175000000113, 69.47500000273116427, 10.91162601494193929 ) ) ;
#13611=CARTESIAN_POINT ( 'NONE',  ( -27.16883889988624290, 50.92500000273118843, -19.73931689729374028 ) ) ;
#13612=CARTESIAN_POINT ( 'NONE',  ( -33.58253175000000113, 13.37500000273118772, 0.000000000000000000 ) ) ;
#13613=CARTESIAN_POINT ( 'NONE',  ( 27.16883889988624290, 4.175000002731188431, 19.73931689729373673 ) ) ;
#13617=CARTESIAN_POINT ( 'NONE',  ( 10.04305231718579705, 73.10000000546239107, 30.90933677959248982 ) ) ;
#13624=CARTESIAN_POINT ( 'NONE',  ( -2.162160676586881955E-15, 44.87500000273119127, -35.31076352940723240 ) ) ;
#13630=CARTESIAN_POINT ( 'NONE',  ( -20.75514604977248112, 15.42500000273118843, 28.56700777964554661 ) ) ;
#13644=CARTESIAN_POINT ( 'NONE',  ( -26.29305231718578995, 12.20000000000000284, 19.10302069950538595 ) ) ;
#13650=CARTESIAN_POINT ( 'NONE',  ( 27.16883889988623935, 74.32500000273118701, -19.73931689729374384 ) ) ;
#13651=CARTESIAN_POINT ( 'NONE',  ( 20.75514604977249178, 32.07500000273117990, 28.56700777964553950 ) ) ;
#13657=CARTESIAN_POINT ( 'NONE',  ( 6.277390505771533514E-15, 56.49999999999998579, 34.17252228774368916 ) ) ;
#13660=EDGE_CURVE ( 'NONE', #20850, #22505, #843, .T. ) ;
#13663=CARTESIAN_POINT ( 'NONE',  ( -20.75514604977248823, 65.07500000273118701, -28.56700777964554305 ) ) ;
#13668=CARTESIAN_POINT ( 'NONE',  ( -2.162160676586881955E-15, 34.62500000273119127, -35.31076352940723240 ) ) ;
#13673=CARTESIAN_POINT ( 'NONE',  ( 5.779280353836490358E-15, 58.49999999999999289, 32.49999999999999289 ) ) ;
#13684=CARTESIAN_POINT ( 'NONE',  ( -1.778240108872766143E-15, 54.00000000546237544, -32.49999999999999289 ) ) ;
#13689=CARTESIAN_POINT ( 'NONE',  ( 33.58253175000000823, 54.27500000273118275, 10.91162601494192863 ) ) ;
#13695=CARTESIAN_POINT ( 'NONE',  ( -26.29305231718579350, 75.80000000000002558, -19.10302069950537884 ) ) ;
#13696=CARTESIAN_POINT ( 'NONE',  ( 10.37757302488624056, 10.52500000273119696, -31.93888565452638417 ) ) ;
#13704=CARTESIAN_POINT ( 'NONE',  ( -33.58253175000000113, 57.22500000273117848, 10.91162601494193929 ) ) ;
#13708=CARTESIAN_POINT ( 'NONE',  ( -10.37757302488624411, 2.725000002731181592, -31.93888565452638417 ) ) ;
#13719=CARTESIAN_POINT ( 'NONE',  ( -20.08610463437156923, 22.29999999999999716, 27.64615127144130113 ) ) ;
#13730=CARTESIAN_POINT ( 'NONE',  ( -33.58253175000000113, 29.12500000273120193, 0.000000000000000000 ) ) ;
#13732=CARTESIAN_POINT ( 'NONE',  ( 26.29305231718578995, 61.70000000546237118, -19.10302069950538240 ) ) ;
#13733=CARTESIAN_POINT ( 'NONE',  ( 32.50000000000000711, 60.89999999999999147, 10.55989012756945122 ) ) ;
#13735=CARTESIAN_POINT ( 'NONE',  ( 20.08610463437157279, 49.80000000546238681, -27.64615127144129758 ) ) ;
#13739=CARTESIAN_POINT ( 'NONE',  ( 33.58253175000000113, 74.12500000273118417, -4.112674001490185761E-15 ) ) ;
#13744=CARTESIAN_POINT ( 'NONE',  ( -32.50000000000000000, 16.50000000546238255, 0.000000000000000000 ) ) ;
#13752=DIRECTION ( 'NONE',  ( 0.000000000000000000, 1.000000000000000000, 0.000000000000000000 ) ) ;
#13763=CARTESIAN_POINT ( 'NONE',  ( 6.486482029760649416E-15, 69.87500000273121259, 35.31076352940723240 ) ) ;
#13768=CARTESIAN_POINT ( 'NONE',  ( 10.37757302488624056, 44.52500000273119696, -31.93888565452638417 ) ) ;
#13769=CARTESIAN_POINT ( 'NONE',  ( 27.16883889988623935, 12.57500000273119234, -19.73931689729374384 ) ) ;
#13770=CARTESIAN_POINT ( 'NONE',  ( 20.75514604977249178, 64.07500000273120122, 28.56700777964553950 ) ) ;
#13774=CARTESIAN_POINT ( 'NONE',  ( 6.277390505771533514E-15, 73.00000000546239676, 34.17252228774368916 ) ) ;
#13782=EDGE_LOOP ( 'NONE', ( #29371, #30134, #29565, #9937 ) ) ;
#13783=CARTESIAN_POINT ( 'NONE',  ( 33.58253175000000113, 48.37500000273119127, -4.112674001490185761E-15 ) ) ;
#13789=CARTESIAN_POINT ( 'NONE',  ( -27.16883889988624290, 14.92500000273118488, -19.73931689729374028 ) ) ;
#13790=EDGE_CURVE ( 'NONE', #18447, #9615, #3072, .T. ) ;
#13792=VERTEX_POINT ( 'NONE', #19055 ) ;
#13806=CARTESIAN_POINT ( 'NONE',  ( 32.50000000000000000, 9.100000000000004974, -10.55989012756945833 ) ) ;
#13812=CARTESIAN_POINT ( 'NONE',  ( -27.16883889988624290, 74.92500000273120975, -19.73931689729374028 ) ) ;
#13814=CARTESIAN_POINT ( 'NONE',  ( 6.486482029760649416E-15, 29.87500000273119838, 35.31076352940723240 ) ) ;
#13815=CARTESIAN_POINT ( 'NONE',  ( 33.58253175000000113, 16.37500000273119127, -4.112674001490185761E-15 ) ) ;
#13821=CARTESIAN_POINT ( 'NONE',  ( 32.50000000000000000, 53.00000000000000711, -3.980102097228898626E-15 ) ) ;
#13826=CARTESIAN_POINT ( 'NONE',  ( -33.58253175000000113, 69.37500000273121259, 0.000000000000000000 ) ) ;
#13831=CARTESIAN_POINT ( 'NONE',  ( -33.58253175000000113, 37.22500000273119980, 10.91162601494193929 ) ) ;
#13835=CARTESIAN_POINT ( 'NONE',  ( 20.75514604977248467, 66.67500000273119554, -28.56700777964554305 ) ) ;
#13844=CARTESIAN_POINT ( 'NONE',  ( -40.00000000000000711, 52.00000000000000711, -23.09401076758504345 ) ) ;
#13854=CARTESIAN_POINT ( 'NONE',  ( -10.37757302488624411, 46.97500000273117848, -31.93888565452638417 ) ) ;
#13861=CARTESIAN_POINT ( 'NONE',  ( -20.08610463437157989, 75.69999999999998863, -27.64615127144129758 ) ) ;
#13862=CARTESIAN_POINT ( 'NONE',  ( 10.37757302488624056, 8.525000002731195181, -31.93888565452638417 ) ) ;
#13866=CARTESIAN_POINT ( 'NONE',  ( -32.50000000000000000, 65.89999999999999147, -10.55989012756945300 ) ) ;
#13871=CARTESIAN_POINT ( 'NONE',  ( 27.16883889988623935, 56.32500000273120122, -19.73931689729374384 ) ) ;
#13887=CARTESIAN_POINT ( 'NONE',  ( -10.04305231718578462, 22.39999999999998792, 30.90933677959249337 ) ) ;
#13896=CARTESIAN_POINT ( 'NONE',  ( 31.92269207768545058, 66.99999999999998579, -6.710300343870453155 ) ) ;
#13898=CARTESIAN_POINT ( 'NONE',  ( 6.486482029760649416E-15, 27.62500000273118062, 35.31076352940723240 ) ) ;
#13904=CARTESIAN_POINT ( 'NONE',  ( 32.50000000000000000, 47.60000000546239818, -10.55989012756945833 ) ) ;
#13908=CARTESIAN_POINT ( 'NONE',  ( -20.75514604977248823, 76.82500000273120122, -28.56700777964554305 ) ) ;
#13911=ORIENTED_EDGE ( 'NONE', *, *, #21409, .F. ) ;
#13913=CARTESIAN_POINT ( 'NONE',  ( 32.50000000000000000, 17.50000000546238255, -3.980102097228898626E-15 ) ) ;
#13931=CARTESIAN_POINT ( 'NONE',  ( -33.58253175000000113, 67.27500000273117564, -10.91162601494193218 ) ) ;
#13936=CARTESIAN_POINT ( 'NONE',  ( -33.58253175000000113, 47.22500000273117138, 10.91162601494193929 ) ) ;
#13937=CARTESIAN_POINT ( 'NONE',  ( -27.16883889988624290, 11.17500000273118133, -19.73931689729374028 ) ) ;
#13938=CARTESIAN_POINT ( 'NONE',  ( 33.58253175000000113, 62.37500000273120548, -4.112674001490185761E-15 ) ) ;
#13942=CARTESIAN_POINT ( 'NONE',  ( 32.50000000000000711, 67.40000000546237402, 10.55989012756945122 ) ) ;
#13949=CARTESIAN_POINT ( 'NONE',  ( -27.16883889988623935, 47.57500000273119412, 19.73931689729374739 ) ) ;
#13954=CARTESIAN_POINT ( 'NONE',  ( 27.16883889988624290, 19.92500000273118843, 19.73931689729373673 ) ) ;
#13969=CARTESIAN_POINT ( 'NONE',  ( -26.29305231718579350, 7.800000000000014921, -19.10302069950537884 ) ) ;
#13975=CARTESIAN_POINT ( 'NONE',  ( 33.58253175000000113, 66.12500000273118417, -4.112674001490185761E-15 ) ) ;
#13976=CARTESIAN_POINT ( 'NONE',  ( 20.75514604977249178, 30.07500000273118701, 28.56700777964553950 ) ) ;
#13977=CARTESIAN_POINT ( 'NONE',  ( 33.58253175000000823, 18.27500000273118275, 10.91162601494192863 ) ) ;
#13985=CARTESIAN_POINT ( 'NONE',  ( -2.092463501923844636E-15, 47.49999999999997868, -34.17252228774368916 ) ) ;
#13991=CARTESIAN_POINT ( 'NONE',  ( -27.16883889988624290, 69.17500000273118133, -19.73931689729374028 ) ) ;
#13997=CARTESIAN_POINT ( 'NONE',  ( 33.58253175000000113, 38.22500000273119269, -10.91162601494193751 ) ) ;
#14013=CARTESIAN_POINT ( 'NONE',  ( -1.778240108872766143E-15, 54.00000000546237544, -32.49999999999999289 ) ) ;
#14017=CARTESIAN_POINT ( 'NONE',  ( 33.58253175000000823, 46.27500000273120406, 10.91162601494192863 ) ) ;
#14023=CARTESIAN_POINT ( 'NONE',  ( -32.50000000000000000, 76.00000000000000000, 0.000000000000000000 ) ) ;
#14025=CARTESIAN_POINT ( 'NONE',  ( -20.75514604977248112, 11.42500000273117955, 28.56700777964554661 ) ) ;
#14029=EDGE_CURVE ( 'NONE', #13792, #17050, #24856, .T. ) ;
#14030=CARTESIAN_POINT ( 'NONE',  ( -1.778240108872766143E-15, 65.50000000000000000, -32.49999999999999289 ) ) ;
#14035=CARTESIAN_POINT ( 'NONE',  ( -20.75514604977248823, 56.82500000273117990, -28.56700777964554305 ) ) ;
#14036=CARTESIAN_POINT ( 'NONE',  ( -33.58253175000000113, 27.47500000273118204, 10.91162601494193929 ) ) ;
#14040=CARTESIAN_POINT ( 'NONE',  ( 10.37757302488624767, 1.725000002731180704, 31.93888565452638417 ) ) ;
#14062=CARTESIAN_POINT ( 'NONE',  ( 32.52223864317537050, 66.99999999999998579, -1.355835680407735611 ) ) ;
#14063=CARTESIAN_POINT ( 'NONE',  ( 6.410174973103799800, 51.99999999999999289, 32.88179426022558260 ) ) ;
#14065=CARTESIAN_POINT ( 'NONE',  ( 33.58253175000000113, 26.12500000273119838, -4.112674001490185761E-15 ) ) ;
#14068=CARTESIAN_POINT ( 'NONE',  ( 32.50000000000000000, 61.09999999999998721, -10.55989012756945833 ) ) ;
#14070=CARTESIAN_POINT ( 'NONE',  ( 10.04305231718578817, 49.90000000546239534, -30.90933677959249337 ) ) ;
#14076=CARTESIAN_POINT ( 'NONE',  ( -20.75514604977248112, 75.42500000273120975, 28.56700777964554661 ) ) ;
#14081=CARTESIAN_POINT ( 'NONE',  ( 6.277390505771533514E-15, 11.00000000546237544, 34.17252228774368916 ) ) ;
#14087=( BOUNDED_CURVE ( )  B_SPLINE_CURVE ( 2, ( #18539, #8216, #18709, #29146, #4974, #23167, #5651, #23346, #26588, #12697, #33807, #33629, #20610 ),
 .UNSPECIFIED., .F., .T. ) 
 B_SPLINE_CURVE_WITH_KNOTS ( ( 3, 2, 2, 2, 2, 2, 3 ),
 ( 0.3269230769230769273, 0.3282051282051282048, 0.3307692307692307598, 0.3333333333333333148, 0.3358974358974358698, 0.3384615384615384803, 0.3397435898119063880 ),
 .UNSPECIFIED. ) 
 CURVE ( )  GEOMETRIC_REPRESENTATION_ITEM ( )  RATIONAL_B_SPLINE_CURVE ( ( 0.9755282581475768211, 0.9755282581475768211, 1.000000000000000000, 0.9510565162951535312, 1.000000000000000000, 0.9510565162951535312, 1.000000000000000000, 0.9510565162951535312, 1.000000000000000000, 0.9510565162951535312, 1.000000000000000000, 0.9755282568435517110, 0.9755282581475768211 ) ) 
 REPRESENTATION_ITEM ( '' )  );
#14090=CARTESIAN_POINT ( 'NONE',  ( -26.29305231718579350, 62.30000000546238681, -19.10302069950537884 ) ) ;
#14092=SURFACE_STYLE_FILL_AREA ( #27293 ) ;
#14093=CARTESIAN_POINT ( 'NONE',  ( 20.08610463437158344, 36.70000000000000995, 27.64615127144129403 ) ) ;
#14101=CARTESIAN_POINT ( 'NONE',  ( 27.16883889988623935, 66.57500000273118701, -19.73931689729374384 ) ) ;
#14106=CARTESIAN_POINT ( 'NONE',  ( 10.37757302488624767, 45.72500000273120691, 31.93888565452638417 ) ) ;
#14107=CARTESIAN_POINT ( 'NONE',  ( 33.58253175000000823, 8.275000002731191628, 10.91162601494192863 ) ) ;
#14108=CARTESIAN_POINT ( 'NONE',  ( -10.37757302488624411, 60.97500000273119269, -31.93888565452638417 ) ) ;
#14112=CARTESIAN_POINT ( 'NONE',  ( -32.50000000000000000, 70.40000000546237402, -10.55989012756945478 ) ) ;
#14119=CARTESIAN_POINT ( 'NONE',  ( 10.37757302488624767, 43.97500000273117848, 31.93888565452638417 ) ) ;
#14122=CARTESIAN_POINT ( 'NONE',  ( 26.29305231718578995, 31.70000000546237118, -19.10302069950538240 ) ) ;
#14124=CARTESIAN_POINT ( 'NONE',  ( -20.75514604977248823, 20.82500000273119412, -28.56700777964554305 ) ) ;
#14140=CARTESIAN_POINT ( 'NONE',  ( -26.29305231718579350, 11.80000000000001847, -19.10302069950537884 ) ) ;
#14146=CARTESIAN_POINT ( 'NONE',  ( -27.16883889988624290, 68.92500000273120975, -19.73931689729374028 ) ) ;
#14147=CARTESIAN_POINT ( 'NONE',  ( -20.75514604977248112, 27.67500000273118133, 28.56700777964554661 ) ) ;
#14148=CARTESIAN_POINT ( 'NONE',  ( -27.16883889988623935, 15.57500000273119589, 19.73931689729374739 ) ) ;
#14153=CARTESIAN_POINT ( 'NONE',  ( 26.29305231718578995, 45.20000000000000284, -19.10302069950538240 ) ) ;
#14159=CARTESIAN_POINT ( 'NONE',  ( 33.58253175000000113, 64.37500000273121259, -4.112674001490185761E-15 ) ) ;
#14164=CARTESIAN_POINT ( 'NONE',  ( 20.75514604977248467, 38.42500000273118133, -28.56700777964554305 ) ) ;
#14169=CARTESIAN_POINT ( 'NONE',  ( -20.08610463437156923, 0.8000000054623763734, 27.64615127144130113 ) ) ;
#14184=CARTESIAN_POINT ( 'NONE',  ( -33.58253175000000113, 51.47500000273118559, 10.91162601494193929 ) ) ;
#14188=CYLINDRICAL_SURFACE ( 'NONE', #10320, 32.50000000000000000 ) ;
#14191=CARTESIAN_POINT ( 'NONE',  ( -26.29305231718578995, 64.20000000000001705, 19.10302069950538595 ) ) ;
#14192=CARTESIAN_POINT ( 'NONE',  ( 10.37757302488624056, 6.525000002731193405, -31.93888565452638417 ) ) ;
#14195=CARTESIAN_POINT ( 'NONE',  ( -5.485892052525789174E-07, 66.99999999999998579, 32.49999999999999289 ) ) ;
#14203=CARTESIAN_POINT ( 'NONE',  ( 33.58253175000000113, 54.22500000273117848, -10.91162601494193751 ) ) ;
#14204=CARTESIAN_POINT ( 'NONE',  ( -10.37757302488623701, 29.77500000273118630, 31.93888565452638417 ) ) ;
#14218=CARTESIAN_POINT ( 'NONE',  ( -10.37757302488623701, 55.52500000273118275, 31.93888565452638417 ) ) ;
#14233=CARTESIAN_POINT ( 'NONE',  ( 27.16883889988624290, 29.92500000273119909, 19.73931689729373673 ) ) ;
#14236=CARTESIAN_POINT ( 'NONE',  ( 5.147494310547434893, 60.55125428154683220, 32.49999999999999289 ) ) ;
#14238=CARTESIAN_POINT ( 'NONE',  ( 32.50000000000000711, 49.40000000546236691, 10.55989012756945122 ) ) ;
#14242=CARTESIAN_POINT ( 'NONE',  ( -10.37757302488624411, 72.72500000273117848, -31.93888565452638417 ) ) ;
#14244=DIRECTION ( 'NONE',  ( 0.000000000000000000, 0.000000000000000000, 1.000000000000000000 ) ) ;
#14247=CARTESIAN_POINT ( 'NONE',  ( 32.50000000000000711, 11.40000000546237580, 10.55989012756945122 ) ) ;
#14256=CARTESIAN_POINT ( 'NONE',  ( -10.04305231718579172, 35.60000000000000853, -30.90933677959248982 ) ) ;
#14265=EDGE_CURVE ( 'NONE', #26368, #19609, #18349, .T. ) ;
#14266=CARTESIAN_POINT ( 'NONE',  ( 6.486482029760649416E-15, 59.87500000273117706, 35.31076352940723240 ) ) ;
#14271=CARTESIAN_POINT ( 'NONE',  ( -20.75514604977248823, 48.82500000273117280, -28.56700777964554305 ) ) ;
#14272=CARTESIAN_POINT ( 'NONE',  ( -2.162160676586881955E-15, 8.875000002731189497, -35.31076352940723240 ) ) ;
#14273=CARTESIAN_POINT ( 'NONE',  ( -27.16883889988623935, 59.57500000273117990, 19.73931689729374739 ) ) ;
#14277=CARTESIAN_POINT ( 'NONE',  ( 32.50000000000000711, 65.40000000546237402, 10.55989012756945122 ) ) ;
#14283=CARTESIAN_POINT ( 'NONE',  ( -20.75514604977248112, 39.67500000273118133, 28.56700777964554661 ) ) ;
#14286=CARTESIAN_POINT ( 'NONE',  ( 6.277390505771533514E-15, 31.00000000546236834, 34.17252228774368916 ) ) ;
#14305=CARTESIAN_POINT ( 'NONE',  ( -20.08610463437157989, 7.699999999999988631, -27.64615127144129758 ) ) ;
#14311=CARTESIAN_POINT ( 'NONE',  ( 20.75514604977249178, 67.82500000273120122, 28.56700777964553950 ) ) ;
#14312=CARTESIAN_POINT ( 'NONE',  ( -10.37757302488624411, 32.97500000273119269, -31.93888565452638417 ) ) ;
#14313=CARTESIAN_POINT ( 'NONE',  ( -20.75514604977248823, 15.07500000273116747, -28.56700777964554305 ) ) ;
#14318=CARTESIAN_POINT ( 'NONE',  ( 20.08610463437157279, 47.29999999999999005, -27.64615127144129758 ) ) ;
#14324=CARTESIAN_POINT ( 'NONE',  ( 20.75514604977248467, 58.67500000273118843, -28.56700777964554305 ) ) ;
#14329=CARTESIAN_POINT ( 'NONE',  ( 27.16883889988623935, 28.32500000273117990, -19.73931689729374384 ) ) ;
#14351=CARTESIAN_POINT ( 'NONE',  ( 27.16883889988624290, 52.17500000273118843, 19.73931689729373673 ) ) ;
#14357=CARTESIAN_POINT ( 'NONE',  ( -10.04305231718579172, 69.59999999999998010, -30.90933677959248982 ) ) ;
#14367=CARTESIAN_POINT ( 'NONE',  ( -33.58253175000000113, 57.02500000273118275, -10.91162601494193218 ) ) ;
#14368=CARTESIAN_POINT ( 'NONE',  ( 33.58253175000000823, 26.27500000273119340, 10.91162601494192863 ) ) ;
#14381=CARTESIAN_POINT ( 'NONE',  ( -33.58253175000000113, 57.12500000273116996, 0.000000000000000000 ) ) ;
#14400=CARTESIAN_POINT ( 'NONE',  ( -27.16883889988623935, 29.32500000273117990, 19.73931689729374739 ) ) ;
#14402=CARTESIAN_POINT ( 'NONE',  ( 10.04305231718579705, 55.10000000546237686, 30.90933677959248982 ) ) ;
#14407=CARTESIAN_POINT ( 'NONE',  ( 20.08610463437157279, 47.80000000546239391, -27.64615127144129758 ) ) ;
#14412=CARTESIAN_POINT ( 'NONE',  ( -20.75514604977248112, 73.42500000273118133, 28.56700777964554661 ) ) ;
#14417=CARTESIAN_POINT ( 'NONE',  ( -2.092463501923844636E-15, 10.00000000546237722, -34.17252228774368916 ) ) ;
#14424=CARTESIAN_POINT ( 'NONE',  ( -5.147494310547430452, 62.05125428700922185, -32.49999999999999289 ) ) ;
#14426=CARTESIAN_POINT ( 'NONE',  ( -10.04305231718578462, 34.39999999999999858, 30.90933677959249337 ) ) ;
#14434=EDGE_LOOP ( 'NONE', ( #10859, #5769, #30515, #1214 ) ) ;
#14438=CARTESIAN_POINT ( 'NONE',  ( 20.75514604977248467, 48.42500000273119554, -28.56700777964554305 ) ) ;
#14439=CARTESIAN_POINT ( 'NONE',  ( -27.16883889988623935, 1.575000002731183457, 19.73931689729374739 ) ) ;
#14440=CARTESIAN_POINT ( 'NONE',  ( -33.58253175000000113, 59.27500000273119696, -10.91162601494193041 ) ) ;
#14444=CARTESIAN_POINT ( 'NONE',  ( 20.08610463437158344, 67.20000000546235697, 27.64615127144129403 ) ) ;
#14447=CARTESIAN_POINT ( 'NONE',  ( -32.50000000000000000, 54.10000000000000853, 10.55989012756946366 ) ) ;
#14451=CARTESIAN_POINT ( 'NONE',  ( -33.58253175000000113, 43.27500000273117564, -10.91162601494193218 ) ) ;
#14453=CARTESIAN_POINT ( 'NONE',  ( 20.08610463437158344, 31.20000000546238894, 27.64615127144129403 ) ) ;
#14463=CARTESIAN_POINT ( 'NONE',  ( 6.486482029760648627E-15, 65.62500000273116996, 35.31076352940722529 ) ) ;
#14472=CARTESIAN_POINT ( 'NONE',  ( -26.29305231718578995, 2.199999999999993516, 19.10302069950538595 ) ) ;
#14477=CARTESIAN_POINT ( 'NONE',  ( -33.58253175000000113, 65.12500000273118417, 0.000000000000000000 ) ) ;
#14478=CARTESIAN_POINT ( 'NONE',  ( 10.37757302488624767, 25.97500000273118914, 31.93888565452638417 ) ) ;
#14479=VECTOR ( 'NONE', #11979, 1000.000000000000000 ) ;
#14480=CARTESIAN_POINT ( 'NONE',  ( -33.58253175000000113, 17.47500000273117848, 10.91162601494193929 ) ) ;
#14486=CARTESIAN_POINT ( 'NONE',  ( 6.277390505771533514E-15, 48.50000000000000711, 34.17252228774368916 ) ) ;
#14491=CARTESIAN_POINT ( 'NONE',  ( -33.58253175000000113, 63.27500000273118985, -10.91162601494193218 ) ) ;
#14497=CARTESIAN_POINT ( 'NONE',  ( 10.37757302488624056, 32.52500000273118985, -31.93888565452638417 ) ) ;
#14518=CARTESIAN_POINT ( 'NONE',  ( 33.58253175000000113, 52.47500000273117138, -10.91162601494193751 ) ) ;
#14524=CARTESIAN_POINT ( 'NONE',  ( 10.04305231718579705, 68.59999999999998010, 30.90933677959248982 ) ) ;
#14534=CARTESIAN_POINT ( 'NONE',  ( -27.16883889988623935, 47.32500000273119412, 19.73931689729374739 ) ) ;
#14535=CARTESIAN_POINT ( 'NONE',  ( 10.37757302488624056, 20.77500000273117919, -31.93888565452638417 ) ) ;
#14552=CARTESIAN_POINT ( 'NONE',  ( 33.58253175000000823, 56.02500000273118275, 10.91162601494192685 ) ) ;
#14563=CARTESIAN_POINT ( 'NONE',  ( 0.000000000000000000, 52.00000000000000711, 32.50000000000000000 ) ) ;
#14564=CARTESIAN_POINT ( 'NONE',  ( -40.00000000000000711, 66.99999999999998579, -23.09401076758504345 ) ) ;
#14567=CARTESIAN_POINT ( 'NONE',  ( -33.58253175000000113, 19.02500000273118630, -10.91162601494193218 ) ) ;
#14569=CARTESIAN_POINT ( 'NONE',  ( 32.50000000000000000, 55.60000000546237686, -10.55989012756945833 ) ) ;
#14572=CARTESIAN_POINT ( 'NONE',  ( 26.29305231718579350, 41.30000000546237260, 19.10302069950537529 ) ) ;
#14577=CARTESIAN_POINT ( 'NONE',  ( 33.58253175000000113, 66.12500000273118417, -4.112674001490185761E-15 ) ) ;
#14583=CARTESIAN_POINT ( 'NONE',  ( 10.04305231718578817, 9.900000005462358033, -30.90933677959249337 ) ) ;
#14594=PRESENTATION_STYLE_ASSIGNMENT (( #1020 ) ) ;
#14595=EDGE_CURVE ( 'NONE', #927, #30177, #19213, .T. ) ;
#14596=CARTESIAN_POINT ( 'NONE',  ( 32.50000000000000000, 33.10000000000000853, -10.55989012756945833 ) ) ;
#14600=CARTESIAN_POINT ( 'NONE',  ( -15.01861347032170180, 66.99999999999998579, 29.12398716250626407 ) ) ;
#14609=CARTESIAN_POINT ( 'NONE',  ( -10.37757302488624411, 38.72500000273119980, -31.93888565452638417 ) ) ;
#14610=CARTESIAN_POINT ( 'NONE',  ( 33.58253175000000113, 6.475000002731178483, -10.91162601494193751 ) ) ;
#14611=CARTESIAN_POINT ( 'NONE',  ( -33.58253175000000113, 57.47500000273118559, 10.91162601494193929 ) ) ;
#14615=CARTESIAN_POINT ( 'NONE',  ( -20.08610463437157989, 70.20000000546237118, -27.64615127144129758 ) ) ;
#14620=CARTESIAN_POINT ( 'NONE',  ( -27.16883889988623935, 39.57500000273118701, 19.73931689729374739 ) ) ;
#14622=ORIENTED_EDGE ( 'NONE', *, *, #11354, .T. ) ;
#14623=CARTESIAN_POINT ( 'NONE',  ( -32.50000000000000000, 30.60000000546238041, 10.55989012756946366 ) ) ;
#14638=LINE ( 'NONE', #1234, #33747 ) ;
#14645=CARTESIAN_POINT ( 'NONE',  ( -32.50000000000000000, 4.000000000000003553, 0.000000000000000000 ) ) ;
#14650=CARTESIAN_POINT ( 'NONE',  ( -33.58253175000000113, 59.12500000273116996, 0.000000000000000000 ) ) ;
#14651=CARTESIAN_POINT ( 'NONE',  ( 27.16883889988624290, 22.17500000273119198, 19.73931689729373673 ) ) ;
#14652=CARTESIAN_POINT ( 'NONE',  ( 10.37757302488624767, 11.97500000273120335, 31.93888565452638417 ) ) ;
#14657=CARTESIAN_POINT ( 'NONE',  ( 10.04305231718578817, 45.40000000000001279, -30.90933677959249337 ) ) ;
#14661=CARTESIAN_POINT ( 'NONE',  ( -10.37757302488624411, 58.97500000273119269, -31.93888565452638417 ) ) ;
#14666=CARTESIAN_POINT ( 'NONE',  ( 20.75514604977248467, 28.42500000273118133, -28.56700777964554305 ) ) ;
#14690=CARTESIAN_POINT ( 'NONE',  ( 27.16883889988623935, 40.57500000273118701, -19.73931689729374384 ) ) ;
#14696=CARTESIAN_POINT ( 'NONE',  ( -2.092463501923844636E-15, 67.50000000000000000, -34.17252228774368916 ) ) ;
#14701=CARTESIAN_POINT ( 'NONE',  ( 10.37757302488624056, 78.77500000273117564, -31.93888565452638417 ) ) ;
#14706=CARTESIAN_POINT ( 'NONE',  ( 20.75514604977249178, 51.82500000273120122, 28.56700777964553950 ) ) ;
#14707=CARTESIAN_POINT ( 'NONE',  ( 33.58253175000000823, 20.27500000273117564, 10.91162601494192863 ) ) ;
#14721=CARTESIAN_POINT ( 'NONE',  ( -10.37757302488624411, 52.72500000273121401, -31.93888565452638417 ) ) ;
#14735=CARTESIAN_POINT ( 'NONE',  ( -32.15037667113026743, 52.00000000000000000, 5.379467130815013043 ) ) ;
#14736=CARTESIAN_POINT ( 'NONE',  ( 10.37757302488624056, 20.52500000273117919, -31.93888565452638417 ) ) ;
#14738=CARTESIAN_POINT ( 'NONE',  ( 20.08610463437157279, 53.29999999999999716, -27.64615127144129758 ) ) ;
#14741=CARTESIAN_POINT ( 'NONE',  ( -26.29305231718578995, 44.70000000546238539, 19.10302069950538595 ) ) ;
#14747=CARTESIAN_POINT ( 'NONE',  ( 20.75514604977248467, 66.42500000273120975, -28.56700777964554305 ) ) ;
#14753=CARTESIAN_POINT ( 'NONE',  ( -33.58253175000000113, 13.12500000273118772, 0.000000000000000000 ) ) ;
#14763=CARTESIAN_POINT ( 'NONE',  ( -32.50000000000000000, 36.10000000000000142, 10.55989012756946366 ) ) ;
#14767=CARTESIAN_POINT ( 'NONE',  ( -6.725304478055195823, 66.99999999999998579, 31.94333337441920762 ) ) ;
#14776=CARTESIAN_POINT ( 'NONE',  ( -20.75514604977248823, 42.82500000273119412, -28.56700777964554305 ) ) ;
#14777=CARTESIAN_POINT ( 'NONE',  ( 20.75514604977248467, 2.675000002731181770, -28.56700777964554305 ) ) ;
#14778=CARTESIAN_POINT ( 'NONE',  ( -33.58253175000000113, 55.47500000273120691, 10.91162601494193929 ) ) ;
#14781=CARTESIAN_POINT ( 'NONE',  ( -20.08610463437156923, 58.80000000546239391, 27.64615127144130113 ) ) ;
#14785=CARTESIAN_POINT ( 'NONE',  ( -20.08610463437157989, 53.69999999999998863, -27.64615127144129758 ) ) ;
#14788=CARTESIAN_POINT ( 'NONE',  ( 33.58253175000000823, 38.27500000273118985, 10.91162601494192863 ) ) ;
#14792=CARTESIAN_POINT ( 'NONE',  ( -10.04305231718578462, 30.90000000546237757, 30.90933677959249337 ) ) ;
#14812=CARTESIAN_POINT ( 'NONE',  ( -27.16883889988624290, 79.17500000273118133, -19.73931689729374028 ) ) ;
#14818=CARTESIAN_POINT ( 'NONE',  ( -27.16883889988624290, 58.92500000273119554, -19.73931689729374028 ) ) ;
#14819=CARTESIAN_POINT ( 'NONE',  ( 10.37757302488624056, 24.77500000273118275, -31.93888565452638417 ) ) ;
#14820=CARTESIAN_POINT ( 'NONE',  ( -33.58253175000000113, 9.275000002731177418, -10.91162601494193218 ) ) ;
#14825=CARTESIAN_POINT ( 'NONE',  ( -32.50000000000000000, 78.50000000546238255, 0.000000000000000000 ) ) ;
#14827=CARTESIAN_POINT ( 'NONE',  ( -26.29305231718579350, 41.79999999999999005, -19.10302069950537884 ) ) ;
#14833=CARTESIAN_POINT ( 'NONE',  ( -10.37757302488623701, 57.77500000273121117, 31.93888565452638417 ) ) ;
#14838=CARTESIAN_POINT ( 'NONE',  ( 20.75514604977248467, 30.42500000273117777, -28.56700777964554305 ) ) ;
#14851=CARTESIAN_POINT ( 'NONE',  ( -1.778240108872766143E-15, 55.49999999999999289, -32.49999999999999289 ) ) ;
#14852=CARTESIAN_POINT ( 'NONE',  ( -20.08610463437156923, 52.30000000000000426, 27.64615127144130113 ) ) ;
#14858=CARTESIAN_POINT ( 'NONE',  ( 10.37757302488624056, 44.77500000273119696, -31.93888565452638417 ) ) ;
#14863=CARTESIAN_POINT ( 'NONE',  ( -32.50000000000000000, 63.89999999999998437, -10.55989012756945478 ) ) ;
#14869=CARTESIAN_POINT ( 'NONE',  ( -10.37757302488624411, 76.97500000273120691, -31.93888565452638417 ) ) ;
#14874=CARTESIAN_POINT ( 'NONE',  ( 27.16883889988623935, 52.32500000273120122, -19.73931689729374384 ) ) ;
#14875=CARTESIAN_POINT ( 'NONE',  ( 10.37757302488624056, 22.77500000273117919, -31.93888565452638417 ) ) ;
#14877=ORIENTED_EDGE ( 'NONE', *, *, #3297, .F. ) ;
#14890=CARTESIAN_POINT ( 'NONE',  ( 5.779280353836490358E-15, 66.49999999999998579, 32.49999999999999289 ) ) ;
#14899=CARTESIAN_POINT ( 'NONE',  ( 10.37757302488624056, 60.77500000273118275, -31.93888565452638417 ) ) ;
#14903=DIRECTION ( 'NONE',  ( -0.8660254037844387076, 0.000000000000000000, -0.4999999999999998335 ) ) ;
#14905=CARTESIAN_POINT ( 'NONE',  ( 10.04305231718579705, 63.10000000546238397, 30.90933677959248982 ) ) ;
#14907=CARTESIAN_POINT ( 'NONE',  ( 10.37757302488624056, 22.52500000273117919, -31.93888565452638417 ) ) ;
#14912=CARTESIAN_POINT ( 'NONE',  ( -32.50000000000000000, 40.40000000546239534, -10.55989012756945478 ) ) ;
#14917=CARTESIAN_POINT ( 'NONE',  ( 20.75514604977248467, 68.42500000273120975, -28.56700777964554305 ) ) ;
#14924=CARTESIAN_POINT ( 'NONE',  ( -20.75514604977248112, 13.42500000273119198, 28.56700777964554661 ) ) ;
#14935=CARTESIAN_POINT ( 'NONE',  ( -10.04305231718579172, 31.60000000000000142, -30.90933677959248982 ) ) ;
#14949=CARTESIAN_POINT ( 'NONE',  ( 33.58253175000000113, 38.22500000273119269, -10.91162601494193751 ) ) ;
#14950=CARTESIAN_POINT ( 'NONE',  ( -10.37757302488623701, 3.775000002731190740, 31.93888565452638417 ) ) ;
#14951=CARTESIAN_POINT ( 'NONE',  ( 27.16883889988623935, 58.57500000273117990, -19.73931689729374384 ) ) ;
#14956=CARTESIAN_POINT ( 'NONE',  ( 32.50000000000000711, 59.40000000546237402, 10.55989012756945122 ) ) ;
#14962=CARTESIAN_POINT ( 'NONE',  ( -33.58253175000000113, 35.37500000273117706, 0.000000000000000000 ) ) ;
#14966=CARTESIAN_POINT ( 'NONE',  ( 10.04305231718579705, 23.10000000546237686, 30.90933677959248982 ) ) ;
#14983=CARTESIAN_POINT ( 'NONE',  ( -26.29305231718579350, 3.799999999999998046, -19.10302069950537884 ) ) ;
#14989=CARTESIAN_POINT ( 'NONE',  ( -33.58253175000000113, 63.22500000273119269, 10.91162601494193929 ) ) ;
#14990=CARTESIAN_POINT ( 'NONE',  ( -10.37757302488623701, 23.77500000273117919, 31.93888565452638417 ) ) ;
#14991=CARTESIAN_POINT ( 'NONE',  ( 20.75514604977249178, 12.07500000273119234, 28.56700777964553950 ) ) ;
#14996=CARTESIAN_POINT ( 'NONE',  ( 27.16883889988623935, 2.325000002731183901, -19.73931689729374384 ) ) ;
#14998=CARTESIAN_POINT ( 'NONE',  ( -26.29305231718578995, 42.20000000000000284, 19.10302069950538595 ) ) ;
#15004=CARTESIAN_POINT ( 'NONE',  ( -33.58253175000000113, 57.47500000273119269, 10.91162601494193929 ) ) ;
#15009=CARTESIAN_POINT ( 'NONE',  ( 10.37757302488624767, 29.72500000273119269, 31.93888565452638417 ) ) ;
#15034=CARTESIAN_POINT ( 'NONE',  ( 20.75514604977248467, 44.67500000273118843, -28.56700777964554305 ) ) ;
#15040=CARTESIAN_POINT ( 'NONE',  ( 32.50000000000000000, 63.10000000000001563, -10.55989012756945833 ) ) ;
#15050=CARTESIAN_POINT ( 'NONE',  ( 6.486482029760649416E-15, 51.62500000273120548, 35.31076352940723240 ) ) ;
#15051=CARTESIAN_POINT ( 'NONE',  ( 33.58253175000000113, 22.37500000273119483, -4.112674001490185761E-15 ) ) ;
#15073=CARTESIAN_POINT ( 'NONE',  ( -10.37757302488623701, 63.77500000273118985, 31.93888565452638417 ) ) ;
#15080=CARTESIAN_POINT ( 'NONE',  ( 20.75514604977249178, 23.82500000273118701, 28.56700777964553950 ) ) ;
#15082=CARTESIAN_POINT ( 'NONE',  ( 26.29305231718578995, 55.70000000546236407, -19.10302069950538240 ) ) ;
#15085=CARTESIAN_POINT ( 'NONE',  ( -10.04305231718578462, 38.90000000546238113, 30.90933677959249337 ) ) ;
#15090=ORIENTED_EDGE ( 'NONE', *, *, #14265, .T. ) ;
#15091=CARTESIAN_POINT ( 'NONE',  ( 27.16883889988624290, 67.92500000273120975, 19.73931689729373673 ) ) ;
#15100=CARTESIAN_POINT ( 'NONE',  ( 27.16883889988623935, 10.32500000273119056, -19.73931689729374384 ) ) ;
#15110=CARTESIAN_POINT ( 'NONE',  ( -32.50000000000000000, 31.90000000000001279, -10.55989012756945478 ) ) ;
#15118=VERTEX_POINT ( 'NONE', #2536 ) ;
#15124=CARTESIAN_POINT ( 'NONE',  ( -10.37757302488624411, 40.72500000273119980, -31.93888565452638417 ) ) ;
#15125=CARTESIAN_POINT ( 'NONE',  ( -27.16883889988624290, 3.175000002731187543, -19.73931689729374028 ) ) ;
#15126=CARTESIAN_POINT ( 'NONE',  ( -27.16883889988624290, 55.17500000273119554, -19.73931689729374028 ) ) ;
#15131=CARTESIAN_POINT ( 'NONE',  ( 6.277390505771533514E-15, 59.00000000546238255, 34.17252228774368916 ) ) ;
#15133=CARTESIAN_POINT ( 'NONE',  ( 20.08610463437157279, 57.80000000546236549, -27.64615127144129758 ) ) ;
#15138=CARTESIAN_POINT ( 'NONE',  ( 20.75514604977248467, 36.67500000273118843, -28.56700777964554305 ) ) ;
#15142=CARTESIAN_POINT ( 'NONE',  ( -32.50000000000000000, 26.50000000546236123, 0.000000000000000000 ) ) ;
#15160=CARTESIAN_POINT ( 'NONE',  ( -26.29305231718579350, 5.799999999999999822, -19.10302069950537884 ) ) ;
#15161=ORIENTED_EDGE ( 'NONE', *, *, #30747, .T. ) ;
#15165=CARTESIAN_POINT ( 'NONE',  ( 27.16883889988623935, 58.32500000273120833, -19.73931689729374384 ) ) ;
#15166=CARTESIAN_POINT ( 'NONE',  ( -33.58253175000000113, 23.27500000273116854, -10.91162601494193218 ) ) ;
#15167=CARTESIAN_POINT ( 'NONE',  ( 20.75514604977248467, 12.67500000273118488, -28.56700777964554305 ) ) ;
#15172=CARTESIAN_POINT ( 'NONE',  ( -10.37757302488624411, 2.725000002731181592, -31.93888565452638417 ) ) ;
#15174=CARTESIAN_POINT ( 'NONE',  ( 26.29305231718578995, 39.19999999999999574, -19.10302069950538240 ) ) ;
#15179=CARTESIAN_POINT ( 'NONE',  ( -27.16883889988624290, 53.17500000273118843, -19.73931689729374028 ) ) ;
#15180=CARTESIAN_POINT ( 'NONE',  ( 32.50000000000000000, 59.60000000546236976, -10.55989012756945833 ) ) ;
#15185=CARTESIAN_POINT ( 'NONE',  ( -10.37757302488623701, 21.52500000273117919, 31.93888565452638417 ) ) ;
#15191=AXIS2_PLACEMENT_3D ( 'NONE', #21970, #16825, #6679 ) ;
#15205=CARTESIAN_POINT ( 'NONE',  ( 6.486482029760649416E-15, 41.87500000273119127, 35.31076352940723240 ) ) ;
#15210=CARTESIAN_POINT ( 'NONE',  ( 32.50000000000000711, 60.89999999999999147, 10.55989012756945122 ) ) ;
#15215=CARTESIAN_POINT ( 'NONE',  ( 20.75514604977248467, 74.67500000273118133, -28.56700777964554305 ) ) ;
#15220=CARTESIAN_POINT ( 'NONE',  ( 20.75514604977248467, 48.42500000273119554, -28.56700777964554305 ) ) ;
#15224=CARTESIAN_POINT ( 'NONE',  ( -20.08610463437157989, 10.20000000546238539, -27.64615127144129758 ) ) ;
#15244=CARTESIAN_POINT ( 'NONE',  ( -10.37757302488623701, 61.77500000273118985, 31.93888565452638417 ) ) ;
#15251=CARTESIAN_POINT ( 'NONE',  ( 32.50000000000000000, 79.10000000000000853, -10.55989012756945833 ) ) ;
#15252=CARTESIAN_POINT ( 'NONE',  ( 27.16883889988624290, 17.92500000273118843, 19.73931689729373673 ) ) ;
#15257=CARTESIAN_POINT ( 'NONE',  ( 20.08610463437158344, 43.20000000546235697, 27.64615127144129403 ) ) ;
#15263=CARTESIAN_POINT ( 'NONE',  ( -27.16883889988624290, 68.92500000273120975, -19.73931689729374028 ) ) ;
#15269=ORIENTED_EDGE ( 'NONE', *, *, #6933, .F. ) ;
#15270=CARTESIAN_POINT ( 'NONE',  ( 6.486482029760649416E-15, 9.625000002731178839, 35.31076352940723240 ) ) ;
#15280=CARTESIAN_POINT ( 'NONE',  ( -10.04305231718578462, 26.39999999999999147, 30.90933677959249337 ) ) ;
#15284=CARTESIAN_POINT ( 'NONE',  ( -2.708425130540669024, 66.99999999999998579, 32.46185396738155049 ) ) ;
#15293=CARTESIAN_POINT ( 'NONE',  ( -27.16883889988623935, 41.32500000273119412, 19.73931689729374739 ) ) ;
#15294=CARTESIAN_POINT ( 'NONE',  ( -32.50000000000000000, 64.60000000546239107, 10.55989012756946366 ) ) ;
#15295=CARTESIAN_POINT ( 'NONE',  ( 20.75514604977249178, 58.07500000273117990, 28.56700777964553950 ) ) ;
#15299=CARTESIAN_POINT ( 'NONE',  ( 20.08610463437158344, 63.20000000546237118, 27.64615127144129403 ) ) ;
#15307=CARTESIAN_POINT ( 'NONE',  ( -20.75514604977248823, 33.07500000273117990, -28.56700777964554305 ) ) ;
#15311=CARTESIAN_POINT ( 'NONE',  ( -32.50000000000000000, 24.50000000546238965, 0.000000000000000000 ) ) ;
#15324=CARTESIAN_POINT ( 'NONE',  ( -27.16883889988623935, 59.32500000273120833, 19.73931689729374739 ) ) ;
#15334=CARTESIAN_POINT ( 'NONE',  ( -27.16883889988623935, 75.57500000273118701, 19.73931689729374739 ) ) ;
#15335=ORIENTED_EDGE ( 'NONE', *, *, #3903, .F. ) ;
#15339=CARTESIAN_POINT ( 'NONE',  ( 10.37757302488624767, 59.72500000273119269, 31.93888565452638417 ) ) ;
#15340=CARTESIAN_POINT ( 'NONE',  ( 33.58253175000000823, 16.27500000273118630, 10.91162601494192863 ) ) ;
#15341=CARTESIAN_POINT ( 'NONE',  ( -10.37757302488623701, 7.775000002731194293, 31.93888565452638417 ) ) ;
#15346=CARTESIAN_POINT ( 'NONE',  ( 20.75514604977249178, 3.825000002731188786, 28.56700777964553950 ) ) ;
#15348=CARTESIAN_POINT ( 'NONE',  ( 10.04305231718579705, 42.60000000000001563, 30.90933677959248982 ) ) ;
#15354=CARTESIAN_POINT ( 'NONE',  ( -20.75514604977248112, 55.67500000273118843, 28.56700777964554661 ) ) ;
#15355=CARTESIAN_POINT ( 'NONE',  ( 26.29305231718578995, 59.70000000546237118, -19.10302069950538240 ) ) ;
#15359=CARTESIAN_POINT ( 'NONE',  ( 6.486482029760649416E-15, 21.62500000273119483, 35.31076352940723240 ) ) ;
#15363=CARTESIAN_POINT ( 'NONE',  ( -26.29305231718578995, 58.20000000000001705, 19.10302069950538595 ) ) ;
#15373=CARTESIAN_POINT ( 'NONE',  ( 32.50000000000000000, 17.00000000000000000, -3.980102097228898626E-15 ) ) ;
#15380=CARTESIAN_POINT ( 'NONE',  ( -33.58253175000000113, 41.47500000273117138, 10.91162601494193929 ) ) ;
#15385=CARTESIAN_POINT ( 'NONE',  ( -20.08610463437157989, 61.69999999999999574, -27.64615127144129758 ) ) ;
#15389=CARTESIAN_POINT ( 'NONE',  ( 6.486482029760649416E-15, 73.87500000273119838, 35.31076352940723240 ) ) ;
#15394=CARTESIAN_POINT ( 'NONE',  ( 10.37757302488624056, 44.52500000273119696, -31.93888565452638417 ) ) ;
#15396=ORIENTED_EDGE ( 'NONE', *, *, #20791, .T. ) ;
#15399=CARTESIAN_POINT ( 'NONE',  ( 10.04305231718578817, 1.900000005462379349, -30.90933677959249337 ) ) ;
#15419=CARTESIAN_POINT ( 'NONE',  ( 27.16883889988624290, 60.17500000273119554, 19.73931689729373673 ) ) ;
#15426=CARTESIAN_POINT ( 'NONE',  ( -2.162160676586881955E-15, 12.62500000273118772, -35.31076352940723240 ) ) ;
#15431=CARTESIAN_POINT ( 'NONE',  ( -2.092463501923844636E-15, 34.00000000546236123, -34.17252228774368916 ) ) ;
#15437=CARTESIAN_POINT ( 'NONE',  ( -10.37757302488624411, 62.72500000273119269, -31.93888565452638417 ) ) ;
#15443=CARTESIAN_POINT ( 'NONE',  ( 10.37757302488624767, 13.72500000273117671, 31.93888565452638417 ) ) ;
#15454=CARTESIAN_POINT ( 'NONE',  ( 6.277390505771533514E-15, 30.49999999999999645, 34.17252228774368916 ) ) ;
#15467=CARTESIAN_POINT ( 'NONE',  ( 29.12397828776036235, 66.99999999999997158, -15.02363756889424273 ) ) ;
#15468=CARTESIAN_POINT ( 'NONE',  ( 10.37757302488624056, 36.52500000273118985, -31.93888565452638417 ) ) ;
#15469=PLANE ( 'NONE',  #20990 ) ;
#15474=CARTESIAN_POINT ( 'NONE',  ( -10.04305231718579172, 58.10000000546237686, -30.90933677959248982 ) ) ;
#15481=CARTESIAN_POINT ( 'NONE',  ( 10.37757302488624056, 34.77500000273118985, -31.93888565452638417 ) ) ;
#15485=CARTESIAN_POINT ( 'NONE',  ( 26.29305231718579350, 25.30000000546238326, 19.10302069950537529 ) ) ;
#15495=CARTESIAN_POINT ( 'NONE',  ( -27.16883889988623935, 61.32500000273120833, 19.73931689729374739 ) ) ;
#15500=VECTOR ( 'NONE', #17315, 1000.000000000000000 ) ;
#15508=CARTESIAN_POINT ( 'NONE',  ( -20.75514604977248823, 77.07500000273117280, -28.56700777964554305 ) ) ;
#15514=CARTESIAN_POINT ( 'NONE',  ( 27.16883889988624290, 55.92500000273119554, 19.73931689729373673 ) ) ;
#15515=CARTESIAN_POINT ( 'NONE',  ( -27.16883889988624290, 19.17500000273118843, -19.73931689729374028 ) ) ;
#15516=CARTESIAN_POINT ( 'NONE',  ( -20.75514604977248823, 7.075000002731188786, -28.56700777964554305 ) ) ;
#15520=CARTESIAN_POINT ( 'NONE',  ( -20.75514604977248112, 3.425000002731186655, 28.56700777964554661 ) ) ;
#15527=CARTESIAN_POINT ( 'NONE',  ( -33.58253175000000113, 55.37500000273119838, 0.000000000000000000 ) ) ;
#15528=CARTESIAN_POINT ( 'NONE',  ( 10.04305231718579705, 59.10000000546237686, 30.90933677959248982 ) ) ;
#15532=CARTESIAN_POINT ( 'NONE',  ( 6.486482029760649416E-15, 25.62500000273118772, 35.31076352940723240 ) ) ;
#15536=CARTESIAN_POINT ( 'NONE',  ( -10.04305231718579172, 57.60000000000000142, -30.90933677959248982 ) ) ;
#15547=CARTESIAN_POINT ( 'NONE',  ( 6.277390505771533514E-15, 18.49999999999999645, 34.17252228774368916 ) ) ;
#15554=CARTESIAN_POINT ( 'NONE',  ( 20.75514604977248467, 36.67500000273118843, -28.56700777964554305 ) ) ;
#15561=EDGE_CURVE ( 'NONE', #32793, #29266, #31126, .T. ) ;
#15562=CARTESIAN_POINT ( 'NONE',  ( -26.29305231718578995, 60.20000000000001705, 19.10302069950538595 ) ) ;
#15567=CARTESIAN_POINT ( 'NONE',  ( 33.58253175000000113, 76.47500000273117848, -10.91162601494193751 ) ) ;
#15572=CARTESIAN_POINT ( 'NONE',  ( 33.58253175000000113, 46.22500000273119269, -10.91162601494193751 ) ) ;
#15576=CARTESIAN_POINT ( 'NONE',  ( -10.04305231718579172, 4.100000005462373309, -30.90933677959248982 ) ) ;
#15595=CARTESIAN_POINT ( 'NONE',  ( 33.58253175000000113, 58.47500000273118559, -10.91162601494193751 ) ) ;
#15601=CARTESIAN_POINT ( 'NONE',  ( 6.277390505771533514E-15, 78.49999999999998579, 34.17252228774368916 ) ) ;
#15602=CARTESIAN_POINT ( 'NONE',  ( -33.58253175000000113, 13.02500000273118985, -10.91162601494193218 ) ) ;
#15608=CARTESIAN_POINT ( 'NONE',  ( 20.08610463437157279, 35.80000000546235128, -27.64615127144129758 ) ) ;
#15615=CARTESIAN_POINT ( 'NONE',  ( -33.58253175000000113, 65.12500000273118417, 0.000000000000000000 ) ) ;
#15620=CARTESIAN_POINT ( 'NONE',  ( 27.16883889988623935, 6.325000002731187898, -19.73931689729374384 ) ) ;
#15631=CARTESIAN_POINT ( 'NONE',  ( 20.08610463437157279, 29.30000000000000782, -27.64615127144129758 ) ) ;
#15635=CARTESIAN_POINT ( 'NONE',  ( -32.61426705943295445, 67.00000000000001421, -7.648559219945903820 ) ) ;
#15641=CARTESIAN_POINT ( 'NONE',  ( 12.18942006770534547, 66.99999999999997158, -30.86762708970427127 ) ) ;
#15643=CARTESIAN_POINT ( 'NONE',  ( -2.162160676586881955E-15, 36.62500000273119127, -35.31076352940723240 ) ) ;
#15648=CARTESIAN_POINT ( 'NONE',  ( 10.04305231718579705, 53.10000000546237686, 30.90933677959248982 ) ) ;
#15656=CARTESIAN_POINT ( 'NONE',  ( 10.37757302488624056, 36.77500000273118985, -31.93888565452638417 ) ) ;
#15660=CARTESIAN_POINT ( 'NONE',  ( 20.08610463437157279, 23.80000000546235839, -27.64615127144129758 ) ) ;
#15671=EDGE_CURVE ( 'NONE', #24911, #25651, #22805, .T. ) ;
#15672=CARTESIAN_POINT ( 'NONE',  ( 20.75514604977248467, 62.42500000273118133, -28.56700777964554305 ) ) ;
#15682=CARTESIAN_POINT ( 'NONE',  ( -27.16883889988624290, 75.17500000273118133, -19.73931689729374028 ) ) ;
#15687=CARTESIAN_POINT ( 'NONE',  ( -33.58253175000000113, 55.12500000273119838, 0.000000000000000000 ) ) ;
#15688=CARTESIAN_POINT ( 'NONE',  ( -10.37757302488623701, 15.77500000273117386, 31.93888565452638417 ) ) ;
#15689=CARTESIAN_POINT ( 'NONE',  ( -33.58253175000000113, 3.375000002731193049, 0.000000000000000000 ) ) ;
#15693=CARTESIAN_POINT ( 'NONE',  ( -20.08610463437156923, 74.80000000546239391, 27.64615127144130113 ) ) ;
#15698=CARTESIAN_POINT ( 'NONE',  ( 10.37757302488624056, 54.77500000273121117, -31.93888565452638417 ) ) ;
#15703=CARTESIAN_POINT ( 'NONE',  ( -33.58253175000000113, 25.12500000273119838, 0.000000000000000000 ) ) ;
#15710=LINE ( 'NONE', #18789, #32200 ) ;
#15719=CARTESIAN_POINT ( 'NONE',  ( -32.50000000000000000, 13.89999999999999858, -10.55989012756945478 ) ) ;
#15725=CARTESIAN_POINT ( 'NONE',  ( 20.75514604977249178, 71.82500000273118701, 28.56700777964553950 ) ) ;
#15726=CARTESIAN_POINT ( 'NONE',  ( -20.75514604977248823, 39.07500000273119412, -28.56700777964554305 ) ) ;
#15732=CARTESIAN_POINT ( 'NONE',  ( 6.277390505771533514E-15, 52.50000000000000000, 34.17252228774368916 ) ) ;
#15736=CARTESIAN_POINT ( 'NONE',  ( 27.16883889988624290, 74.17500000273118133, 19.73931689729373673 ) ) ;
#15740=EDGE_LOOP ( 'NONE', ( #21438, #16406, #8330, #11325 ) ) ;
#15742=CARTESIAN_POINT ( 'NONE',  ( -33.58253175000000113, 41.12500000273118417, 0.000000000000000000 ) ) ;
#15746=CARTESIAN_POINT ( 'NONE',  ( -20.08610463437156923, 4.800000005462381480, 27.64615127144130113 ) ) ;
#15766=CARTESIAN_POINT ( 'NONE',  ( -2.162160676586881955E-15, 52.87500000273119838, -35.31076352940723240 ) ) ;
#15773=CARTESIAN_POINT ( 'NONE',  ( 10.37757302488624056, 14.52500000273120051, -31.93888565452638417 ) ) ;
#15778=CARTESIAN_POINT ( 'NONE',  ( 20.08610463437158344, 33.20000000546238539, 27.64615127144129403 ) ) ;
#15783=CARTESIAN_POINT ( 'NONE',  ( 20.75514604977249178, 59.82500000273117280, 28.56700777964553950 ) ) ;
#15788=CARTESIAN_POINT ( 'NONE',  ( 20.75514604977248467, 4.425000002731183990, -28.56700777964554305 ) ) ;
#15797=CARTESIAN_POINT ( 'NONE',  ( 20.08610463437157279, 21.29999999999999716, -27.64615127144129758 ) ) ;
#15808=CARTESIAN_POINT ( 'NONE',  ( 20.30017892146906533, 66.99999999999995737, -26.02681000244154674 ) ) ;
#15810=CARTESIAN_POINT ( 'NONE',  ( 27.16883889988623935, 34.32500000273118701, -19.73931689729374384 ) ) ;
#15811=CARTESIAN_POINT ( 'NONE',  ( -20.08610463437157989, 64.20000000546238539, -27.64615127144129758 ) ) ;
#15815=CARTESIAN_POINT ( 'NONE',  ( 10.04305231718578817, 55.90000000546240244, -30.90933677959249337 ) ) ;
#15823=CARTESIAN_POINT ( 'NONE',  ( 10.37757302488624056, 30.77500000273118630, -31.93888565452638417 ) ) ;
#15827=CARTESIAN_POINT ( 'NONE',  ( 26.29305231718579350, 19.30000000546237970, 19.10302069950537529 ) ) ;
#15836=CARTESIAN_POINT ( 'NONE',  ( -33.58253175000000113, 61.22500000273119269, 10.91162601494193929 ) ) ;
#15841=CARTESIAN_POINT ( 'NONE',  ( 40.00000000000000000, 66.99999999999998579, -23.09401076758505766 ) ) ;
#15846=CARTESIAN_POINT ( 'NONE',  ( 10.37757302488624767, 75.97500000273120691, 31.93888565452638417 ) ) ;
#15851=CARTESIAN_POINT ( 'NONE',  ( 27.16883889988623935, 54.32500000273120122, -19.73931689729374384 ) ) ;
#15852=CARTESIAN_POINT ( 'NONE',  ( -20.75514604977248112, 17.67500000273117422, 28.56700777964554661 ) ) ;
#15853=CARTESIAN_POINT ( 'NONE',  ( -33.58253175000000113, 79.12500000273118417, 0.000000000000000000 ) ) ;
#15857=CARTESIAN_POINT ( 'NONE',  ( 6.277390505771533514E-15, 71.00000000546235412, 34.17252228774368916 ) ) ;
#15858=CARTESIAN_POINT ( 'NONE',  ( 33.25271216035365285, 52.00000000000002132, 3.649504031948850979 ) ) ;
#15864=CARTESIAN_POINT ( 'NONE',  ( -20.75514604977248823, 55.07500000273117990, -28.56700777964554305 ) ) ;
#15869=CARTESIAN_POINT ( 'NONE',  ( 33.58253175000000113, 24.22500000273119625, -10.91162601494193751 ) ) ;
#15875=DIRECTION ( 'NONE',  ( 0.000000000000000000, 1.000000000000000000, 0.000000000000000000 ) ) ;
#15885=CARTESIAN_POINT ( 'NONE',  ( -26.29305231718578995, 18.20000000000000639, 19.10302069950538595 ) ) ;
#15891=CARTESIAN_POINT ( 'NONE',  ( -33.58253175000000113, 75.02500000273117564, -10.91162601494193218 ) ) ;
#15892=CARTESIAN_POINT ( 'NONE',  ( 6.486482029760649416E-15, 37.87500000273117706, 35.31076352940723240 ) ) ;
#15899=CARTESIAN_POINT ( 'NONE',  ( -2.092463501923844636E-15, 53.50000000000000000, -34.17252228774368916 ) ) ;
#15904=CARTESIAN_POINT ( 'NONE',  ( 27.16883889988623935, 74.57500000273118701, -19.73931689729374384 ) ) ;
#15905=CARTESIAN_POINT ( 'NONE',  ( -26.29305231718578995, 62.20000000000001705, 19.10302069950538595 ) ) ;
#15910=CARTESIAN_POINT ( 'NONE',  ( 20.75514604977248467, 40.42500000273117422, -28.56700777964554305 ) ) ;
#15915=CARTESIAN_POINT ( 'NONE',  ( -32.50000000000000000, 4.600000005462372421, 10.55989012756946366 ) ) ;
#15922=DIRECTION ( 'NONE',  ( 0.000000000000000000, 1.000000000000000000, 0.000000000000000000 ) ) ;
#15934=CARTESIAN_POINT ( 'NONE',  ( -2.162160676586881955E-15, 54.87500000273119127, -35.31076352940723240 ) ) ;
#15940=CARTESIAN_POINT ( 'NONE',  ( 26.29305231718578995, 71.20000000000000284, -19.10302069950538240 ) ) ;
#15941=CARTESIAN_POINT ( 'NONE',  ( 20.75514604977249178, 13.82500000273117813, 28.56700777964553950 ) ) ;
#15945=CARTESIAN_POINT ( 'NONE',  ( 20.08610463437158344, 35.20000000546237828, 27.64615127144129403 ) ) ;
#15951=CARTESIAN_POINT ( 'NONE',  ( 10.37757302488624767, 59.72500000273119269, 31.93888565452638417 ) ) ;
#15955=CARTESIAN_POINT ( 'NONE',  ( -10.37757302488623701, 3.525000002731190740, 31.93888565452638417 ) ) ;
#15965=CARTESIAN_POINT ( 'NONE',  ( 32.50000000000000711, 20.90000000000000924, 10.55989012756945122 ) ) ;
#15975=CARTESIAN_POINT ( 'NONE',  ( -10.35455269120598132, 66.99999999999998579, -31.92933819309194732 ) ) ;
#15976=CARTESIAN_POINT ( 'NONE',  ( -23.31009017153187202, 52.00000000000001421, 23.30172593756756427 ) ) ;
#15977=CARTESIAN_POINT ( 'NONE',  ( 6.486482029760649416E-15, 37.62500000273118417, 35.31076352940723240 ) ) ;
#15979=CARTESIAN_POINT ( 'NONE',  ( -10.04305231718578462, 64.90000000546237402, 30.90933677959249337 ) ) ;
#15984=CARTESIAN_POINT ( 'NONE',  ( -20.08610463437156923, 54.80000000546237260, 27.64615127144130113 ) ) ;
#15985=EDGE_CURVE ( 'NONE', #30034, #32793, #29694, .T. ) ;
#15991=CARTESIAN_POINT ( 'NONE',  ( -10.37757302488623701, 27.77500000273118275, 31.93888565452638417 ) ) ;
#15995=CARTESIAN_POINT ( 'NONE',  ( 32.50000000000000711, 15.40000000546236514, 10.55989012756945122 ) ) ;
#16006=CARTESIAN_POINT ( 'NONE',  ( -33.58253175000000113, 59.02500000273120406, -10.91162601494193041 ) ) ;
#16010=( BOUNDED_CURVE ( )  B_SPLINE_CURVE ( 2, ( #22450, #9580, #12500, #20058, #9230, #30161, #1848, #30503, #27774, #7003, #14905, #22968, #6665 ),
 .UNSPECIFIED., .F., .T. ) 
 B_SPLINE_CURVE_WITH_KNOTS ( ( 3, 2, 2, 2, 2, 2, 3 ),
 ( 0.1858974358974359031, 0.1871794871794871806, 0.1897435897435897356, 0.1923076923076923184, 0.1948717948717948734, 0.1974358974358974284, 0.1987179487179487336 ),
 .UNSPECIFIED. ) 
 CURVE ( )  GEOMETRIC_REPRESENTATION_ITEM ( )  RATIONAL_B_SPLINE_CURVE ( ( 0.9755282581475768211, 0.9755282581475768211, 1.000000000000000000, 0.9510565162951535312, 1.000000000000000000, 0.9510565162951535312, 1.000000000000000000, 0.9510565162951535312, 1.000000000000000000, 0.9510565162951535312, 1.000000000000000000, 0.9755282581475764880, 0.9755282581475768211 ) ) 
 REPRESENTATION_ITEM ( '' )  );
#16017=CARTESIAN_POINT ( 'NONE',  ( -27.16883889988623935, 71.57500000273118701, 19.73931689729374739 ) ) ;
#16021=CARTESIAN_POINT ( 'NONE',  ( 10.37757302488624056, 54.52500000273118275, -31.93888565452638417 ) ) ;
#16022=CARTESIAN_POINT ( 'NONE',  ( -20.75514604977248112, 19.67500000273119909, 28.56700777964554661 ) ) ;
#16023=CARTESIAN_POINT ( 'NONE',  ( 33.58253175000000113, 4.375000002731193938, -4.112674001490185761E-15 ) ) ;
#16027=CARTESIAN_POINT ( 'NONE',  ( -20.08610463437157989, 74.20000000546238539, -27.64615127144129758 ) ) ;
#16028=CARTESIAN_POINT ( 'NONE',  ( 2.708425130540434544, 52.00000000000002842, -32.46185396738157891 ) ) ;
#16034=CARTESIAN_POINT ( 'NONE',  ( 10.37757302488624056, 50.77500000273120406, -31.93888565452638417 ) ) ;
#16039=CARTESIAN_POINT ( 'NONE',  ( -10.37757302488624411, 18.72500000273118204, -31.93888565452638417 ) ) ;
#16052=CARTESIAN_POINT ( 'NONE',  ( -1.778240108872766143E-15, 63.50000000000000000, -32.49999999999999289 ) ) ;
#16056=CARTESIAN_POINT ( 'NONE',  ( -20.08610463437156923, 18.30000000000000782, 27.64615127144130113 ) ) ;
#16062=CARTESIAN_POINT ( 'NONE',  ( -10.37757302488624411, 72.72500000273117848, -31.93888565452638417 ) ) ;
#16063=CARTESIAN_POINT ( 'NONE',  ( -27.16883889988623935, 37.57500000273118701, 19.73931689729374739 ) ) ;
#16068=AXIS2_PLACEMENT_3D ( 'NONE', #20446, #30896, #17875 ) ;
#16069=CARTESIAN_POINT ( 'NONE',  ( 32.50000000000000000, 55.00000000000000711, -3.980102097228898626E-15 ) ) ;
#16075=CARTESIAN_POINT ( 'NONE',  ( 20.75514604977248467, 68.67500000273119554, -28.56700777964554305 ) ) ;
#16076=CARTESIAN_POINT ( 'NONE',  ( -10.04305231718578462, 62.39999999999999858, 30.90933677959249337 ) ) ;
#16080=ORIENTED_EDGE ( 'NONE', *, *, #15561, .T. ) ;
#16081=CARTESIAN_POINT ( 'NONE',  ( 10.37757302488624056, 42.52500000273119696, -31.93888565452638417 ) ) ;
#16085=CARTESIAN_POINT ( 'NONE',  ( 10.37757302488624056, 66.77500000273118985, -31.93888565452638417 ) ) ;
#16086=CARTESIAN_POINT ( 'NONE',  ( 20.08610463437158344, 5.200000005462368513, 27.64615127144129403 ) ) ;
#16087=DIRECTION ( 'NONE',  ( 0.000000000000000000, 1.000000000000000000, 0.000000000000000000 ) ) ;
#16103=DIRECTION ( 'NONE',  ( 0.000000000000000000, 0.000000000000000000, 1.000000000000000000 ) ) ;
#16107=CARTESIAN_POINT ( 'NONE',  ( 10.37757302488624767, 55.97500000273118559, 31.93888565452638417 ) ) ;
#16113=CARTESIAN_POINT ( 'NONE',  ( 32.50000000000000000, 75.09999999999999432, -10.55989012756945833 ) ) ;
#16114=CARTESIAN_POINT ( 'NONE',  ( 27.16883889988624290, 9.925000002731207971, 19.73931689729373673 ) ) ;
#16122=CARTESIAN_POINT ( 'NONE',  ( -20.75514604977248112, 63.42500000273118133, 28.56700777964554661 ) ) ;
#16126=CARTESIAN_POINT ( 'NONE',  ( 6.486482029760649416E-15, 7.625000002731185056, 35.31076352940723240 ) ) ;
#16136=CARTESIAN_POINT ( 'NONE',  ( -32.50000000000000000, 24.00000000000000711, 0.000000000000000000 ) ) ;
#16149=CARTESIAN_POINT ( 'NONE',  ( 10.35455269120621047, 52.00000000000001421, 31.92933819309184429 ) ) ;
#16150=CARTESIAN_POINT ( 'NONE',  ( -33.58253175000000113, 35.12500000273117706, 0.000000000000000000 ) ) ;
#16151=CARTESIAN_POINT ( 'NONE',  ( -5.147494310547322094, 56.05125428700920764, -32.50000000000003553 ) ) ;
#16155=CARTESIAN_POINT ( 'NONE',  ( 6.277390505771533514E-15, 57.00000000546238965, 34.17252228774368916 ) ) ;
#16160=CARTESIAN_POINT ( 'NONE',  ( -33.58253175000000113, 29.37500000273117351, 0.000000000000000000 ) ) ;
#16164=CARTESIAN_POINT ( 'NONE',  ( -32.50000000000000000, 18.50000000546238255, 0.000000000000000000 ) ) ;
#16174=CARTESIAN_POINT ( 'NONE',  ( 31.04172217648528687, 52.00000000000000711, 12.81397374188273908 ) ) ;
#16180=CARTESIAN_POINT ( 'NONE',  ( -5.485892052525789174E-07, 66.99999999999998579, 32.49999999999999289 ) ) ;
#16181=DIRECTION ( 'NONE',  ( 0.000000000000000000, 1.000000000000000000, 0.000000000000000000 ) ) ;
#16185=CARTESIAN_POINT ( 'NONE',  ( -33.58253175000000113, 71.37500000273121259, 0.000000000000000000 ) ) ;
#16190=CARTESIAN_POINT ( 'NONE',  ( 6.486482029760649416E-15, 51.62500000273120548, 35.31076352940723240 ) ) ;
#16191=CARTESIAN_POINT ( 'NONE',  ( 20.75514604977249178, 12.07500000273119234, 28.56700777964553950 ) ) ;
#16192=CARTESIAN_POINT ( 'NONE',  ( 20.75514604977248467, 4.675000002731191096, -28.56700777964554305 ) ) ;
#16196=CARTESIAN_POINT ( 'NONE',  ( 20.08610463437158344, 73.20000000546235697, 27.64615127144129403 ) ) ;
#16197=CARTESIAN_POINT ( 'NONE',  ( 24.23786831611837655, 51.99999999999999289, -22.37122307655969067 ) ) ;
#16203=CARTESIAN_POINT ( 'NONE',  ( -10.37757302488623701, 45.77500000273119696, 31.93888565452638417 ) ) ;
#16208=CARTESIAN_POINT ( 'NONE',  ( -33.58253175000000113, 19.12500000273119483, 0.000000000000000000 ) ) ;
#16225=CARTESIAN_POINT ( 'NONE',  ( 6.277390505771533514E-15, 8.499999999999992895, 34.17252228774368916 ) ) ;
#16231=CARTESIAN_POINT ( 'NONE',  ( -33.58253175000000113, 75.12500000273118417, 0.000000000000000000 ) ) ;
#16232=CARTESIAN_POINT ( 'NONE',  ( -20.75514604977248112, 37.67500000273118133, 28.56700777964554661 ) ) ;
#16237=CARTESIAN_POINT ( 'NONE',  ( -32.50000000000000000, 54.10000000000000853, 10.55989012756946366 ) ) ;
#16241=CARTESIAN_POINT ( 'NONE',  ( 27.16883889988623935, 68.57500000273118701, -19.73931689729374384 ) ) ;
#16247=CARTESIAN_POINT ( 'NONE',  ( 27.16883889988624290, 35.92500000273117422, 19.73931689729373673 ) ) ;
#16269=CARTESIAN_POINT ( 'NONE',  ( 27.16883889988624290, 54.17500000273118843, 19.73931689729373673 ) ) ;
#16276=CARTESIAN_POINT ( 'NONE',  ( 10.04305231718578817, 73.40000000000000568, -30.90933677959249337 ) ) ;
#16277=CARTESIAN_POINT ( 'NONE',  ( 33.58253175000000113, 12.22500000273118381, -10.91162601494193751 ) ) ;
#16285=CARTESIAN_POINT ( 'NONE',  ( -20.75514604977248112, 57.42500000273118843, 28.56700777964554661 ) ) ;
#16289=CARTESIAN_POINT ( 'NONE',  ( 20.75514604977248467, 2.425000002731189763, -28.56700777964554305 ) ) ;
#16298=AXIS2_PLACEMENT_3D ( 'NONE', #30014, #32752, #14244 ) ;
#16299=B_SPLINE_CURVE_WITH_KNOTS ( 'NONE', 3,
 ( #7728, #5327, #15975, #31066, #157, #23525, #28660, #31405, #23865, #10648, #332, #23182, #23358, #10818, #8066, #31738, #5156, #15641, #18723, #26092, #10478, #12882, #29159, #15808, #5666, #3098, #33645, #10142, #18045, #7561, #28489, #15467, #25920, #33819, #32069, #1162, #3424, #29998, #13896, #24363, #26768, #11154, #14062, #21955 ),
 .UNSPECIFIED., .F., .F.,
 ( 4, 2, 2, 2, 2, 2, 2, 2, 2, 2, 2, 2, 2, 2, 2, 2, 2, 2, 2, 2, 2, 4 ),
 ( 0.000000000000000000, 0.004064997385822684446, 0.008129994771645368892, 0.01219499215746805247, 0.01422749085037939600, 0.01625998954329073778, 0.02032498692911342136, 0.02235748562202476489, 0.02438998431493610147, 0.02845498170075878158, 0.03251997908658145475, 0.03455247777949279481, 0.03658497647240413486, 0.04064997385822680803, 0.04471497124404947426, 0.04877996862987214050, 0.05081246732278348055, 0.05284496601569481367, 0.05690996340151748684, 0.05894246209442883383, 0.06097496078734017388, 0.06503995817316285399 ),
 .UNSPECIFIED. ) ;
#16300=CARTESIAN_POINT ( 'NONE',  ( -10.04305231718579172, 25.59999999999999787, -30.90933677959248982 ) ) ;
#16314=CARTESIAN_POINT ( 'NONE',  ( 6.486482029760649416E-15, 29.62500000273120193, 35.31076352940723240 ) ) ;
#16319=CARTESIAN_POINT ( 'NONE',  ( 10.04305231718578817, 45.90000000546238823, -30.90933677959249337 ) ) ;
#16321=CARTESIAN_POINT ( 'NONE',  ( -10.04305231718578462, 58.90000000546240244, 30.90933677959249337 ) ) ;
#16329=CARTESIAN_POINT ( 'NONE',  ( 6.277390505771533514E-15, 17.00000000546237544, 34.17252228774368916 ) ) ;
#16336=CARTESIAN_POINT ( 'NONE',  ( 0.000000000000000000, 52.00000000000000711, 0.000000000000000000 ) ) ;
#16339=CARTESIAN_POINT ( 'NONE',  ( -33.58253175000000113, 53.22500000273118559, 10.91162601494193929 ) ) ;
#16347=CARTESIAN_POINT ( 'NONE',  ( -20.75514604977248823, 71.07500000273117280, -28.56700777964554305 ) ) ;
#16353=CARTESIAN_POINT ( 'NONE',  ( -20.75514604977248823, 44.82500000273117990, -28.56700777964554305 ) ) ;
#16354=CARTESIAN_POINT ( 'NONE',  ( 6.486482029760649416E-15, 11.87500000273118062, 35.31076352940723240 ) ) ;
#16355=CARTESIAN_POINT ( 'NONE',  ( 10.37757302488624767, 63.97500000273119269, 31.93888565452638417 ) ) ;
#16359=CARTESIAN_POINT ( 'NONE',  ( -2.092463501923844636E-15, 72.00000000546236834, -34.17252228774368916 ) ) ;
#16367=CARTESIAN_POINT ( 'NONE',  ( -33.58253175000000113, 47.37500000273119127, 0.000000000000000000 ) ) ;
#16373=CARTESIAN_POINT ( 'NONE',  ( -33.58253175000000113, 17.02500000273118985, -10.91162601494193218 ) ) ;
#16383=CARTESIAN_POINT ( 'NONE',  ( -5.147494310547430452, 63.55125428154684641, -32.49999999999999289 ) ) ;
#16387=CARTESIAN_POINT ( 'NONE',  ( -10.04305231718578462, 10.40000000000000568, 30.90933677959249337 ) ) ;
#16393=CARTESIAN_POINT ( 'NONE',  ( -20.75514604977248823, 70.82500000273117280, -28.56700777964554305 ) ) ;
#16394=CARTESIAN_POINT ( 'NONE',  ( -27.16883889988624290, 33.17500000273120264, -19.73931689729374028 ) ) ;
#16395=CARTESIAN_POINT ( 'NONE',  ( 33.58253175000000113, 18.37500000273119127, -4.112674001490185761E-15 ) ) ;
#16401=CARTESIAN_POINT ( 'NONE',  ( -10.04305231718579172, 55.59999999999999432, -30.90933677959248982 ) ) ;
#16406=ORIENTED_EDGE ( 'NONE', *, *, #30108, .F. ) ;
#16407=CARTESIAN_POINT ( 'NONE',  ( -20.75514604977248823, 67.07500000273118701, -28.56700777964554305 ) ) ;
#16414=CARTESIAN_POINT ( 'NONE',  ( -33.58253175000000113, 39.12500000273118417, 0.000000000000000000 ) ) ;
#16415=CYLINDRICAL_SURFACE ( 'NONE', #29658, 32.50000000000000000 ) ;
#16418=CARTESIAN_POINT ( 'NONE',  ( -10.37757302488624411, 66.97500000273119269, -31.93888565452638417 ) ) ;
#16435=CARTESIAN_POINT ( 'NONE',  ( 33.58253175000000823, 48.27500000273119696, 10.91162601494192863 ) ) ;
#16440=CARTESIAN_POINT ( 'NONE',  ( -10.04305231718578462, 70.40000000000000568, 30.90933677959249337 ) ) ;
#16441=CARTESIAN_POINT ( 'NONE',  ( -27.16883889988623935, 9.325000002731190563, 19.73931689729374739 ) ) ;
#16450=CARTESIAN_POINT ( 'NONE',  ( 6.486482029760649416E-15, 55.62500000273119838, 35.31076352940723240 ) ) ;
#16462=CARTESIAN_POINT ( 'NONE',  ( -26.29305231718579350, 21.80000000000000071, -19.10302069950537884 ) ) ;
#16472=CARTESIAN_POINT ( 'NONE',  ( 11.64495469945098627, 52.00000000000000000, 31.50463004621144947 ) ) ;
#16473=CARTESIAN_POINT ( 'NONE',  ( 27.16883889988623935, 28.32500000273117990, -19.73931689729374384 ) ) ;
#16474=CARTESIAN_POINT ( 'NONE',  ( -32.50000000000000000, 56.50000000546238965, 0.000000000000000000 ) ) ;
#16477=CARTESIAN_POINT ( 'NONE',  ( 32.50000000000000000, 45.50000000546238255, -3.980102097228898626E-15 ) ) ;
#16479=CARTESIAN_POINT ( 'NONE',  ( -5.147494310547423346, 58.94874572391554324, 32.50000000000000000 ) ) ;
#16482=CARTESIAN_POINT ( 'NONE',  ( -33.58253175000000113, 77.22500000273117848, 10.91162601494193929 ) ) ;
#16487=CARTESIAN_POINT ( 'NONE',  ( 26.29305231718579350, 15.30000000546237438, 19.10302069950537529 ) ) ;
#16496=FACE_OUTER_BOUND ( 'NONE', #8084, .T. ) ;
#16508=CARTESIAN_POINT ( 'NONE',  ( 33.58253175000000823, 68.27500000273120406, 10.91162601494192863 ) ) ;
#16512=CARTESIAN_POINT ( 'NONE',  ( 3.980102097228898626E-15, 52.00000000000000711, -32.50000000000000000 ) ) ;
#16513=CARTESIAN_POINT ( 'NONE',  ( 33.58253175000000113, 50.12500000273119127, -4.112674001490185761E-15 ) ) ;
#16514=CARTESIAN_POINT ( 'NONE',  ( -33.58253175000000113, 9.375000002731184168, 0.000000000000000000 ) ) ;
#16515=CARTESIAN_POINT ( 'NONE',  ( -2.162160676586882350E-15, 64.87500000273119838, -35.31076352940722529 ) ) ;
#16519=CARTESIAN_POINT ( 'NONE',  ( -2.092463501923844636E-15, 68.00000000546236834, -34.17252228774368916 ) ) ;
#16526=CARTESIAN_POINT ( 'NONE',  ( 33.58253175000000113, 48.47500000273118559, -10.91162601494193751 ) ) ;
#16533=CARTESIAN_POINT ( 'NONE',  ( -20.75514604977248823, 14.82500000273117635, -28.56700777964554305 ) ) ;
#16548=CARTESIAN_POINT ( 'NONE',  ( 32.50000000000000711, 10.89999999999998792, 10.55989012756945122 ) ) ;
#16555=CARTESIAN_POINT ( 'NONE',  ( -27.16883889988623935, 69.32500000273118701, 19.73931689729374739 ) ) ;
#16556=CARTESIAN_POINT ( 'NONE',  ( -10.37757302488623701, 27.77500000273118275, 31.93888565452638417 ) ) ;
#16557=CARTESIAN_POINT ( 'NONE',  ( -20.75514604977248823, 19.07500000273118701, -28.56700777964554305 ) ) ;
#16564=CARTESIAN_POINT ( 'NONE',  ( 10.04305231718578817, 47.39999999999998437, -30.90933677959249337 ) ) ;
#16569=CARTESIAN_POINT ( 'NONE',  ( 33.58253175000000113, 64.47500000273120691, -10.91162601494193751 ) ) ;
#16574=CARTESIAN_POINT ( 'NONE',  ( -20.75514604977248112, 37.42500000273118843, 28.56700777964554661 ) ) ;
#16579=CARTESIAN_POINT ( 'NONE',  ( 5.147494310547434893, 58.55125428154683220, 32.49999999999999289 ) ) ;
#16597=CARTESIAN_POINT ( 'NONE',  ( 33.58253175000000113, 50.37500000273119127, -4.112674001490185761E-15 ) ) ;
#16605=CARTESIAN_POINT ( 'NONE',  ( 20.08610463437158344, 74.70000000000000284, 27.64615127144129403 ) ) ;
#16606=CARTESIAN_POINT ( 'NONE',  ( 33.58253175000000113, 8.125000002731184168, -4.112674001490185761E-15 ) ) ;
#16608=DIRECTION ( 'NONE',  ( 0.000000000000000000, 0.000000000000000000, 1.000000000000000000 ) ) ;
#16610=CARTESIAN_POINT ( 'NONE',  ( -20.08610463437157989, 65.69999999999998863, -27.64615127144129758 ) ) ;
#16615=CARTESIAN_POINT ( 'NONE',  ( 20.75514604977248467, 54.42500000273117422, -28.56700777964554305 ) ) ;
#16639=EDGE_CURVE ( 'NONE', #1221, #21685, #16299, .T. ) ;
#16640=EDGE_CURVE ( 'NONE', #19648, #21685, #28871, .T. ) ;
#16643=CARTESIAN_POINT ( 'NONE',  ( 0.3462681986485906527, 52.00000000000000000, 33.37691080753738504 ) ) ;
#16644=CARTESIAN_POINT ( 'NONE',  ( -10.37757302488624411, 30.72500000273119269, -31.93888565452638417 ) ) ;
#16645=CARTESIAN_POINT ( 'NONE',  ( 5.779280353836490358E-15, 56.49999999999998579, 32.49999999999999289 ) ) ;
#16650=CARTESIAN_POINT ( 'NONE',  ( -32.50000000000000000, 50.60000000546236265, 10.55989012756946366 ) ) ;
#16654=CARTESIAN_POINT ( 'NONE',  ( 33.58253175000000113, 78.22500000273119269, -10.91162601494193751 ) ) ;
#16659=CARTESIAN_POINT ( 'NONE',  ( -32.50000000000000000, 12.50000000546237722, 0.000000000000000000 ) ) ;
#16666=CARTESIAN_POINT ( 'NONE',  ( -1.053607264507113999E-13, 63.00000000546238255, 32.50000000000000711 ) ) ;
#16676=CARTESIAN_POINT ( 'NONE',  ( -27.16883889988624290, 71.17500000273118133, -19.73931689729374028 ) ) ;
#16681=CARTESIAN_POINT ( 'NONE',  ( 27.16883889988623935, 44.32500000273119412, -19.73931689729374384 ) ) ;
#16682=CARTESIAN_POINT ( 'NONE',  ( 33.58253175000000113, 8.375000002731184168, -4.112674001490185761E-15 ) ) ;
#16683=CARTESIAN_POINT ( 'NONE',  ( -10.37757302488624411, 64.97500000273119269, -31.93888565452638417 ) ) ;
#16687=CARTESIAN_POINT ( 'NONE',  ( -10.04305231718579172, 70.10000000546239107, -30.90933677959248982 ) ) ;
#16694=CARTESIAN_POINT ( 'NONE',  ( -33.58253175000000113, 47.27500000273116143, -10.91162601494193218 ) ) ;
#16698=CARTESIAN_POINT ( 'NONE',  ( 26.29305231718579350, 29.30000000546238681, 19.10302069950537529 ) ) ;
#16700=CARTESIAN_POINT ( 'NONE',  ( -2.162160676586881955E-15, 20.62500000273119483, -35.31076352940723240 ) ) ;
#16701=ADVANCED_FACE ( 'NONE', ( #27096 ), #21625, .T. ) ;
#16718=CARTESIAN_POINT ( 'NONE',  ( -20.08610463437157989, 9.699999999999999289, -27.64615127144129758 ) ) ;
#16719=ORIENTED_EDGE ( 'NONE', *, *, #30107, .F. ) ;
#16724=CARTESIAN_POINT ( 'NONE',  ( -20.75514604977248112, 67.42500000273118133, 28.56700777964554661 ) ) ;
#16725=CARTESIAN_POINT ( 'NONE',  ( 10.37757302488624767, 29.97500000273119269, 31.93888565452638417 ) ) ;
#16726=CARTESIAN_POINT ( 'NONE',  ( -10.37757302488623701, 19.77500000273117564, 31.93888565452638417 ) ) ;
#16732=CARTESIAN_POINT ( 'NONE',  ( 20.08610463437157279, 49.29999999999998295, -27.64615127144129758 ) ) ;
#16737=CARTESIAN_POINT ( 'NONE',  ( 6.486482029760649416E-15, 67.87500000273116996, 35.31076352940723240 ) ) ;
#16742=CARTESIAN_POINT ( 'NONE',  ( -2.162160676586881955E-15, 36.62500000273119127, -35.31076352940723240 ) ) ;
#16762=CARTESIAN_POINT ( 'NONE',  ( 33.58253175000000823, 52.27500000273118985, 10.91162601494192863 ) ) ;
#16766=FACE_OUTER_BOUND ( 'NONE', #2650, .T. ) ;
#16768=CARTESIAN_POINT ( 'NONE',  ( 20.08610463437157279, 65.29999999999999716, -27.64615127144129758 ) ) ;
#16769=CARTESIAN_POINT ( 'NONE',  ( -20.75514604977248823, 6.825000002731195892, -28.56700777964554305 ) ) ;
#16779=CARTESIAN_POINT ( 'NONE',  ( 27.16883889988624290, 57.92500000273119554, 19.73931689729373673 ) ) ;
#16780=CARTESIAN_POINT ( 'NONE',  ( 33.58253175000000823, 30.27500000273118630, 10.91162601494192863 ) ) ;
#16811=CARTESIAN_POINT ( 'NONE',  ( -31.32135535759083567, 52.00000000000002132, 9.352374566761922026 ) ) ;
#16812=UNCERTAINTY_MEASURE_WITH_UNIT (LENGTH_MEASURE( 1.000000000000000082E-05 ), #6530, 'distance_accuracy_value', 'NONE');
#16813=CARTESIAN_POINT ( 'NONE',  ( 33.58253175000000113, 28.12500000273120193, -4.112674001490185761E-15 ) ) ;
#16818=CARTESIAN_POINT ( 'NONE',  ( -2.092463501923844636E-15, 46.00000000546238965, -34.17252228774368916 ) ) ;
#16822=CARTESIAN_POINT ( 'NONE',  ( 33.58253175000000823, 76.02500000273118985, 10.91162601494192863 ) ) ;
#16825=DIRECTION ( 'NONE',  ( 1.000000000000000000, -0.000000000000000000, 0.000000000000000000 ) ) ;
#16828=CARTESIAN_POINT ( 'NONE',  ( 10.04305231718578817, 11.90000000546235981, -30.90933677959249337 ) ) ;
#16838=CARTESIAN_POINT ( 'NONE',  ( -32.50000000000000000, 37.99999999999999289, 0.000000000000000000 ) ) ;
#16846=CARTESIAN_POINT ( 'NONE',  ( -27.16883889988623935, 63.57500000273117990, 19.73931689729374739 ) ) ;
#16851=CARTESIAN_POINT ( 'NONE',  ( -2.162160676586881955E-15, 46.62500000273119127, -35.31076352940723240 ) ) ;
#16852=CARTESIAN_POINT ( 'NONE',  ( -27.16883889988623935, 11.57500000273119234, 19.73931689729374739 ) ) ;
#16853=CARTESIAN_POINT ( 'NONE',  ( -27.16883889988624290, 63.17500000273117422, -19.73931689729374028 ) ) ;
#16857=CARTESIAN_POINT ( 'NONE',  ( 10.04305231718578817, 65.90000000546237402, -30.90933677959249337 ) ) ;
#16863=CARTESIAN_POINT ( 'NONE',  ( 33.58253175000000113, 42.47500000273119980, -10.91162601494193751 ) ) ;
#16865=CARTESIAN_POINT ( 'NONE',  ( -10.04305231718578462, 26.90000000546237402, 30.90933677959249337 ) ) ;
#16873=FACE_OUTER_BOUND ( 'NONE', #28153, .T. ) ;
#16882=CARTESIAN_POINT ( 'NONE',  ( 20.08610463437158344, 8.700000000000002842, 27.64615127144129403 ) ) ;
#16888=CARTESIAN_POINT ( 'NONE',  ( 10.37757302488624767, 67.72500000273116427, 31.93888565452638417 ) ) ;
#16889=CARTESIAN_POINT ( 'NONE',  ( -20.75514604977248823, 29.07500000273119056, -28.56700777964554305 ) ) ;
#16890=CARTESIAN_POINT ( 'NONE',  ( 20.75514604977249178, 14.07500000273119944, 28.56700777964553950 ) ) ;
#16897=CARTESIAN_POINT ( 'NONE',  ( -26.29305231718579350, 45.79999999999999005, -19.10302069950537884 ) ) ;
#16902=CARTESIAN_POINT ( 'NONE',  ( -27.16883889988624290, 61.17500000273119554, -19.73931689729374028 ) ) ;
#16907=CARTESIAN_POINT ( 'NONE',  ( -33.58253175000000113, 35.12500000273117706, 0.000000000000000000 ) ) ;
#16923=EDGE_CURVE ( 'NONE', #1690, #5766, #16010, .T. ) ;
#16925=CARTESIAN_POINT ( 'NONE',  ( 5.147494310547434893, 53.05125428700921475, 32.49999999999999289 ) ) ;
#16931=CARTESIAN_POINT ( 'NONE',  ( 33.58253175000000113, 48.47500000273118559, -10.91162601494193751 ) ) ;
#16938=CARTESIAN_POINT ( 'NONE',  ( 6.277390505771533514E-15, 68.50000000000002842, 34.17252228774368916 ) ) ;
#16947=ORIENTED_EDGE ( 'NONE', *, *, #13790, .T. ) ;
#16948=CARTESIAN_POINT ( 'NONE',  ( -33.58253175000000113, 53.22500000273118559, 10.91162601494193929 ) ) ;
#16949=CARTESIAN_POINT ( 'NONE',  ( 20.75514604977248467, 30.67500000273119909, -28.56700777964554305 ) ) ;
#16963=CARTESIAN_POINT ( 'NONE',  ( 20.75514604977248467, 52.42500000273118133, -28.56700777964554305 ) ) ;
#16978=CARTESIAN_POINT ( 'NONE',  ( -33.58253175000000113, 25.12500000273119838, 0.000000000000000000 ) ) ;
#16981=CARTESIAN_POINT ( 'NONE',  ( 20.08610463437157279, 61.30000000000001137, -27.64615127144129758 ) ) ;
#16983=CARTESIAN_POINT ( 'NONE',  ( -26.29305231718579350, 46.30000000546237260, -19.10302069950537884 ) ) ;
#16987=CARTESIAN_POINT ( 'NONE',  ( -20.75514604977248112, 77.42500000273119554, 28.56700777964554661 ) ) ;
#16989=CARTESIAN_POINT ( 'NONE',  ( 3.980102097228898626E-15, 52.00000000000000711, -32.50000000000000000 ) ) ;
#16992=CARTESIAN_POINT ( 'NONE',  ( -10.04305231718578462, 10.90000000546235981, 30.90933677959249337 ) ) ;
#17001=CARTESIAN_POINT ( 'NONE',  ( -32.50000000000000000, 62.40000000546236691, -10.55989012756945300 ) ) ;
#17004=CARTESIAN_POINT ( 'NONE',  ( 10.04305231718579705, 36.60000000000000853, 30.90933677959248982 ) ) ;
#17016=CARTESIAN_POINT ( 'NONE',  ( -2.162160676586881955E-15, 48.62500000273118417, -35.31076352940723240 ) ) ;
#17017=CARTESIAN_POINT ( 'NONE',  ( 6.486482029760649416E-15, 1.875000002731192383, 35.31076352940723240 ) ) ;
#17018=CARTESIAN_POINT ( 'NONE',  ( 10.37757302488624056, 60.77500000273118275, -31.93888565452638417 ) ) ;
#17023=CARTESIAN_POINT ( 'NONE',  ( 6.277390505771533514E-15, 69.00000000546239676, 34.17252228774368916 ) ) ;
#17029=CARTESIAN_POINT ( 'NONE',  ( -33.58253175000000113, 41.27500000273117564, -10.91162601494193218 ) ) ;
#17031=CARTESIAN_POINT ( 'NONE',  ( -26.29305231718579350, 32.30000000546238681, -19.10302069950537884 ) ) ;
#17035=ORIENTED_EDGE ( 'NONE', *, *, #11313, .T. ) ;
#17049=CARTESIAN_POINT ( 'NONE',  ( 32.50000000000000000, 3.099999999999989875, -10.55989012756945833 ) ) ;
#17050=VERTEX_POINT ( 'NONE', #31365 ) ;
#17055=CARTESIAN_POINT ( 'NONE',  ( 10.37757302488624056, 66.52500000273118985, -31.93888565452638417 ) ) ;
#17056=CARTESIAN_POINT ( 'NONE',  ( -2.162160676586881955E-15, 20.87500000273119127, -35.31076352940723240 ) ) ;
#17057=CARTESIAN_POINT ( 'NONE',  ( -10.37757302488624411, 18.97500000273118204, -31.93888565452638417 ) ) ;
#17063=CARTESIAN_POINT ( 'NONE',  ( 32.50000000000000000, 47.00000000000000000, -3.980102097228898626E-15 ) ) ;
#17064=AXIS2_PLACEMENT_3D ( 'NONE', #31684, #15922, #2702 ) ;
#17069=CARTESIAN_POINT ( 'NONE',  ( -33.58253175000000113, 63.37500000273120548, 0.000000000000000000 ) ) ;
#17074=CARTESIAN_POINT ( 'NONE',  ( -20.75514604977248823, 32.82500000273118701, -28.56700777964554305 ) ) ;
#17098=CARTESIAN_POINT ( 'NONE',  ( -20.75514604977248823, 49.07500000273117280, -28.56700777964554305 ) ) ;
#17104=CARTESIAN_POINT ( 'NONE',  ( -26.29305231718578995, 68.20000000000000284, 19.10302069950538595 ) ) ;
#17109=CARTESIAN_POINT ( 'NONE',  ( 10.37757302488624056, 76.77500000273117564, -31.93888565452638417 ) ) ;
#17115=CARTESIAN_POINT ( 'NONE',  ( -33.58253175000000113, 49.22500000273119269, 10.91162601494193929 ) ) ;
#17116=CARTESIAN_POINT ( 'NONE',  ( -10.37757302488624411, 20.97500000273118559, -31.93888565452638417 ) ) ;
#17132=CARTESIAN_POINT ( 'NONE',  ( -27.16883889988623935, 57.32500000273120833, 19.73931689729374739 ) ) ;
#17148=CARTESIAN_POINT ( 'NONE',  ( 33.58253175000000113, 20.22500000273117848, -10.91162601494193751 ) ) ;
#17150=CARTESIAN_POINT ( 'NONE',  ( 5.147494310547327423, 52.55125428154686062, 32.50000000000003553 ) ) ;
#17153=CARTESIAN_POINT ( 'NONE',  ( 26.29305231718578995, 39.70000000546237828, -19.10302069950538240 ) ) ;
#17161=CARTESIAN_POINT ( 'NONE',  ( 20.75514604977249178, 73.82500000273121543, 28.56700777964553950 ) ) ;
#17166=CARTESIAN_POINT ( 'NONE',  ( 32.50000000000000000, 13.50000000546237899, -3.980102097228898626E-15 ) ) ;
#17175=CARTESIAN_POINT ( 'NONE',  ( 32.50000000000000000, 37.09999999999999432, -10.55989012756945833 ) ) ;
#17188=CARTESIAN_POINT ( 'NONE',  ( -10.37757302488624411, 42.72500000273119980, -31.93888565452638417 ) ) ;
#17189=CARTESIAN_POINT ( 'NONE',  ( 10.37757302488624056, 6.775000002731193405, -31.93888565452638417 ) ) ;
#17190=CARTESIAN_POINT ( 'NONE',  ( -20.75514604977248823, 59.07500000273120122, -28.56700777964554305 ) ) ;
#17194=CARTESIAN_POINT ( 'NONE',  ( -32.50000000000000000, 64.40000000546238823, -10.55989012756945478 ) ) ;
#17200=CARTESIAN_POINT ( 'NONE',  ( -2.162160676586881955E-15, 40.87500000273119838, -35.31076352940723240 ) ) ;
#17202=CARTESIAN_POINT ( 'NONE',  ( -10.04305231718578462, 32.90000000546238113, 30.90933677959249337 ) ) ;
#17212=CARTESIAN_POINT ( 'NONE',  ( -31.04172217648553556, 66.99999999999998579, -12.81397374188210136 ) ) ;
#17222=CARTESIAN_POINT ( 'NONE',  ( -20.08610463437156923, 2.299999999999999822, 27.64615127144130113 ) ) ;
#17226=CARTESIAN_POINT ( 'NONE',  ( -33.58253175000000113, 67.12500000273118417, 0.000000000000000000 ) ) ;
#17227=CARTESIAN_POINT ( 'NONE',  ( -20.75514604977248112, 25.67500000273118488, 28.56700777964554661 ) ) ;
#17228=CARTESIAN_POINT ( 'NONE',  ( -33.58253175000000113, 7.375000002731183280, 0.000000000000000000 ) ) ;
#17233=CARTESIAN_POINT ( 'NONE',  ( 26.29305231718579350, 46.79999999999999716, 19.10302069950537529 ) ) ;
#17234=CARTESIAN_POINT ( 'NONE',  ( 5.779280353836490358E-15, 57.00000000546238965, 32.49999999999999289 ) ) ;
#17239=CARTESIAN_POINT ( 'NONE',  ( -33.58253175000000113, 59.27500000273119696, -10.91162601494193218 ) ) ;
#17244=CARTESIAN_POINT ( 'NONE',  ( 20.75514604977249178, 29.82500000273119767, 28.56700777964553950 ) ) ;
#17265=CARTESIAN_POINT ( 'NONE',  ( -20.75514604977248112, 43.67500000273119554, 28.56700777964554661 ) ) ;
#17269=VECTOR ( 'NONE', #12288, 1000.000000000000000 ) ;
#17271=CARTESIAN_POINT ( 'NONE',  ( -32.50000000000000000, 69.90000000000000568, -10.55989012756945478 ) ) ;
#17281=CARTESIAN_POINT ( 'NONE',  ( -20.75514604977248112, 51.42500000273118133, 28.56700777964554661 ) ) ;
#17282=CARTESIAN_POINT ( 'NONE',  ( 33.58253175000000113, 20.37500000273119483, -4.112674001490185761E-15 ) ) ;
#17292=( BOUNDED_CURVE ( )  B_SPLINE_CURVE ( 2, ( #24759, #17389, #17562, #1412, #1237, #30582, #22198, #7078, #11715, #22874, #33332, #32976, #27854 ),
 .UNSPECIFIED., .F., .T. ) 
 B_SPLINE_CURVE_WITH_KNOTS ( ( 3, 2, 2, 2, 2, 2, 3 ),
 ( 0.3012820512820512664, 0.3025641025641025439, 0.3051282051282051544, 0.3076923076923077094, 0.3102564102564102644, 0.3128205128205128194, 0.3141025641025640969 ),
 .UNSPECIFIED. ) 
 CURVE ( )  GEOMETRIC_REPRESENTATION_ITEM ( )  RATIONAL_B_SPLINE_CURVE ( ( 0.9755282581475768211, 0.9755282581475768211, 1.000000000000000000, 0.9510565162951535312, 1.000000000000000000, 0.9510565162951535312, 1.000000000000000000, 0.9510565162951535312, 1.000000000000000000, 0.9510565162951535312, 1.000000000000000000, 0.9755282581475768211, 0.9755282581475768211 ) ) 
 REPRESENTATION_ITEM ( '' )  );
#17295=CARTESIAN_POINT ( 'NONE',  ( 5.147494310547434893, 66.55125428154683220, 32.49999999999999289 ) ) ;
#17298=CARTESIAN_POINT ( 'NONE',  ( -27.16883889988624290, 54.92500000273118843, -19.73931689729374028 ) ) ;
#17314=CARTESIAN_POINT ( 'NONE',  ( 6.486482029760649416E-15, 23.62500000273119127, 35.31076352940723240 ) ) ;
#17315=DIRECTION ( 'NONE',  ( 0.000000000000000000, 1.000000000000000000, 0.000000000000000000 ) ) ;
#17319=CARTESIAN_POINT ( 'NONE',  ( 20.08610463437157279, 43.80000000546237970, -27.64615127144129758 ) ) ;
#17324=CARTESIAN_POINT ( 'NONE',  ( 10.37757302488624056, 70.52500000273118985, -31.93888565452638417 ) ) ;
#17326=CARTESIAN_POINT ( 'NONE',  ( 40.00000000000000000, 52.00000000000000711, 23.09401076758503990 ) ) ;
#17327=ORIENTED_EDGE ( 'NONE', *, *, #29070, .F. ) ;
#17331=CARTESIAN_POINT ( 'NONE',  ( 27.16883889988623935, 8.325000002731188786, -19.73931689729374384 ) ) ;
#17341=CARTESIAN_POINT ( 'NONE',  ( 32.50000000000000000, 38.99999999999999289, -3.980102097228898626E-15 ) ) ;
#17345=CARTESIAN_POINT ( 'NONE',  ( -5.393181536354430428, 66.99999999999997158, 32.17179393301731949 ) ) ;
#17354=CARTESIAN_POINT ( 'NONE',  ( 33.58253175000000113, 42.22500000273118559, -10.91162601494193751 ) ) ;
#17355=CARTESIAN_POINT ( 'NONE',  ( 20.75514604977249178, 2.075000002731186122, 28.56700777964553950 ) ) ;
#17356=CARTESIAN_POINT ( 'NONE',  ( -10.37757302488624411, 52.97500000273118559, -31.93888565452638417 ) ) ;
#17360=CARTESIAN_POINT ( 'NONE',  ( -20.08610463437156923, 60.80000000546239391, 27.64615127144130113 ) ) ;
#17363=CARTESIAN_POINT ( 'NONE',  ( -10.04305231718579172, 53.60000000000002274, -30.90933677959248982 ) ) ;
#17367=CARTESIAN_POINT ( 'NONE',  ( -27.16883889988624290, 39.17500000273120264, -19.73931689729374028 ) ) ;
#17371=CARTESIAN_POINT ( 'NONE',  ( 10.04305231718578817, 29.90000000546237757, -30.90933677959249337 ) ) ;
#17381=CARTESIAN_POINT ( 'NONE',  ( -33.58253175000000113, 65.12500000273118417, 0.000000000000000000 ) ) ;
#17389=CARTESIAN_POINT ( 'NONE',  ( -5.147494310547423346, 56.44874571845313938, 32.50000000000000000 ) ) ;
#17390=PLANE ( 'NONE',  #21598 ) ;
#17392=CARTESIAN_POINT ( 'NONE',  ( 33.58253175000000113, 78.37500000273118417, -4.112674001490185761E-15 ) ) ;
#17397=CARTESIAN_POINT ( 'NONE',  ( -10.37757302488623701, 59.52500000273118275, 31.93888565452638417 ) ) ;
#17398=CARTESIAN_POINT ( 'NONE',  ( -33.58253175000000113, 23.47500000273119269, 10.91162601494193929 ) ) ;
#17399=CARTESIAN_POINT ( 'NONE',  ( 20.75514604977249178, 8.075000002731185234, 28.56700777964553950 ) ) ;
#17403=CARTESIAN_POINT ( 'NONE',  ( 10.37757302488624767, 1.725000002731180704, 31.93888565452638417 ) ) ;
#17406=CARTESIAN_POINT ( 'NONE',  ( 6.277390505771533514E-15, 42.50000000000000000, 34.17252228774368916 ) ) ;
#17412=CARTESIAN_POINT ( 'NONE',  ( 10.37757302488624767, 57.97500000273118559, 31.93888565452638417 ) ) ;
#17417=AXIS2_PLACEMENT_3D ( 'NONE', #3492, #5737, #19120 ) ;
#17418=CARTESIAN_POINT ( 'NONE',  ( -2.162160676586881955E-15, 30.62500000273119838, -35.31076352940723240 ) ) ;
#17433=CARTESIAN_POINT ( 'NONE',  ( -2.165007332552593587E-13, 52.50000000000000711, 32.50000000000000000 ) ) ;
#17439=CARTESIAN_POINT ( 'NONE',  ( 10.37757302488624767, 45.97500000273117848, 31.93888565452638417 ) ) ;
#17446=CARTESIAN_POINT ( 'NONE',  ( 26.29305231718579350, 64.80000000000001137, 19.10302069950537529 ) ) ;
#17452=CARTESIAN_POINT ( 'NONE',  ( 33.58253175000000113, 78.37500000273118417, -4.112674001490185761E-15 ) ) ;
#17457=CARTESIAN_POINT ( 'NONE',  ( -20.75514604977248823, 50.82500000273116569, -28.56700777964554305 ) ) ;
#17458=CARTESIAN_POINT ( 'NONE',  ( -10.37757302488624411, 22.97500000273118559, -31.93888565452638417 ) ) ;
#17479=CARTESIAN_POINT ( 'NONE',  ( -33.58253175000000113, 59.37500000273119838, 0.000000000000000000 ) ) ;
#17487=CARTESIAN_POINT ( 'NONE',  ( 20.75514604977248467, 22.42500000273119909, -28.56700777964554305 ) ) ;
#17489=CARTESIAN_POINT ( 'NONE',  ( 5.147494310547434893, 55.05125428700922896, 32.49999999999999289 ) ) ;
#17492=CARTESIAN_POINT ( 'NONE',  ( 32.50000000000000000, 41.50000000546237544, -3.980102097228898626E-15 ) ) ;
#17497=CARTESIAN_POINT ( 'NONE',  ( 20.75514604977249178, 71.82500000273118701, 28.56700777964553950 ) ) ;
#17503=CARTESIAN_POINT ( 'NONE',  ( 20.75514604977248467, 14.42500000273119021, -28.56700777964554305 ) ) ;
#17513=CARTESIAN_POINT ( 'NONE',  ( 26.29305231718579350, 30.80000000000000782, 19.10302069950537529 ) ) ;
#17517=CARTESIAN_POINT ( 'NONE',  ( -16.81447360525995194, 66.99999999999995737, 28.18961368868553663 ) ) ;
#17526=CARTESIAN_POINT ( 'NONE',  ( 33.58253175000000823, 42.02500000273118985, 10.91162601494192863 ) ) ;
#17527=CARTESIAN_POINT ( 'NONE',  ( -20.75514604977248823, 5.075000002731193227, -28.56700777964554305 ) ) ;
#17528=CARTESIAN_POINT ( 'NONE',  ( 27.16883889988624290, 58.17500000273119554, 19.73931689729373673 ) ) ;
#17532=CARTESIAN_POINT ( 'NONE',  ( -10.04305231718579172, 62.10000000546238397, -30.90933677959248982 ) ) ;
#17539=CARTESIAN_POINT ( 'NONE',  ( 33.58253175000000113, 40.37500000273118417, -4.112674001490185761E-15 ) ) ;
#17543=CARTESIAN_POINT ( 'NONE',  ( 32.50000000000000711, 25.40000000546236691, 10.55989012756945122 ) ) ;
#17562=CARTESIAN_POINT ( 'NONE',  ( -10.04305231718578462, 56.39999999999999147, 30.90933677959249337 ) ) ;
#17563=CARTESIAN_POINT ( 'NONE',  ( 16.87750156402159618, 52.00000000000001421, 29.11635311643962964 ) ) ;
#17564=CARTESIAN_POINT ( 'NONE',  ( -33.58253175000000113, 79.27500000273118985, -10.91162601494193218 ) ) ;
#17565=VERTEX_POINT ( 'NONE', #1291 ) ;
#17569=CARTESIAN_POINT ( 'NONE',  ( 27.16883889988624290, 57.92500000273119554, 19.73931689729373673 ) ) ;
#17570=CARTESIAN_POINT ( 'NONE',  ( -33.58253175000000113, 23.37500000273119838, 0.000000000000000000 ) ) ;
#17571=CARTESIAN_POINT ( 'NONE',  ( 20.75514604977248467, 8.675000002731195536, -28.56700777964554305 ) ) ;
#17575=CARTESIAN_POINT ( 'NONE',  ( -33.58253175000000113, 5.125000002731180615, 0.000000000000000000 ) ) ;
#17577=CARTESIAN_POINT ( 'NONE',  ( 10.04305231718578817, 43.40000000000000568, -30.90933677959249337 ) ) ;
#17582=CARTESIAN_POINT ( 'NONE',  ( 27.16883889988623935, 60.57500000273117990, -19.73931689729374384 ) ) ;
#17587=CARTESIAN_POINT ( 'NONE',  ( 10.37757302488624056, 30.52500000273118630, -31.93888565452638417 ) ) ;
#17606=CARTESIAN_POINT ( 'NONE',  ( 20.75514604977249178, 46.07500000273117280, 28.56700777964553950 ) ) ;
#17611=CARTESIAN_POINT ( 'NONE',  ( 20.08610463437157279, 61.30000000000001847, -27.64615127144129758 ) ) ;
#17617=CARTESIAN_POINT ( 'NONE',  ( -27.16883889988624290, 79.17500000273118133, -19.73931689729374028 ) ) ;
#17622=CARTESIAN_POINT ( 'NONE',  ( 10.37757302488624767, 51.72500000273121401, 31.93888565452638417 ) ) ;
#17623=CARTESIAN_POINT ( 'NONE',  ( -20.75514604977248823, 25.07500000273120122, -28.56700777964554305 ) ) ;
#17648=CARTESIAN_POINT ( 'NONE',  ( -2.162160676586881955E-15, 64.87500000273119838, -35.31076352940723240 ) ) ;
#17652=CARTESIAN_POINT ( 'NONE',  ( 40.00000000000000000, 52.00000000000000711, -23.09401076758505766 ) ) ;
#17655=CARTESIAN_POINT ( 'NONE',  ( -20.75514604977248112, 21.42500000273120264, 28.56700777964554661 ) ) ;
#17660=CARTESIAN_POINT ( 'NONE',  ( 20.08610463437157279, 41.80000000546237260, -27.64615127144129758 ) ) ;
#17666=CARTESIAN_POINT ( 'NONE',  ( -10.37757302488623701, 69.52500000273118985, 31.93888565452638417 ) ) ;
#17673=CARTESIAN_POINT ( 'NONE',  ( 20.75514604977249178, 11.82500000273118346, 28.56700777964553950 ) ) ;
#17684=CARTESIAN_POINT ( 'NONE',  ( 20.08610463437158344, 30.69999999999999218, 27.64615127144129403 ) ) ;
#17693=ORIENTED_EDGE ( 'NONE', *, *, #33051, .F. ) ;
#17698=CARTESIAN_POINT ( 'NONE',  ( -33.58253175000000113, 39.02500000273118985, -10.91162601494193218 ) ) ;
#17699=CARTESIAN_POINT ( 'NONE',  ( -27.16883889988624290, 5.175000002731189319, -19.73931689729374028 ) ) ;
#17700=CARTESIAN_POINT ( 'NONE',  ( 20.75514604977248467, 54.67500000273119554, -28.56700777964554305 ) ) ;
#17705=CARTESIAN_POINT ( 'NONE',  ( 26.29305231718578995, 59.70000000546237118, -19.10302069950538240 ) ) ;
#17712=CARTESIAN_POINT ( 'NONE',  ( -2.162160676586881955E-15, 32.87500000273118417, -35.31076352940723240 ) ) ;
#17716=CARTESIAN_POINT ( 'NONE',  ( 32.50000000000000000, 25.50000000546236123, -3.980102097228898626E-15 ) ) ;
#17735=CARTESIAN_POINT ( 'NONE',  ( 26.29305231718579350, 2.799999999999997158, 19.10302069950537529 ) ) ;
#17740=CARTESIAN_POINT ( 'NONE',  ( 27.16883889988623935, 60.32500000273120833, -19.73931689729374384 ) ) ;
#17741=CARTESIAN_POINT ( 'NONE',  ( 20.75514604977248467, 22.67500000273119198, -28.56700777964554305 ) ) ;
#17742=CARTESIAN_POINT ( 'NONE',  ( 10.37757302488624056, 8.775000002731166759, -31.93888565452638417 ) ) ;
#17746=CARTESIAN_POINT ( 'NONE',  ( 6.277390505771533514E-15, 77.00000000546235412, 34.17252228774368916 ) ) ;
#17748=CARTESIAN_POINT ( 'NONE',  ( -10.04305231718578462, 42.40000000000000568, 30.90933677959249337 ) ) ;
#17753=ORIENTED_EDGE ( 'NONE', *, *, #4310, .F. ) ;
#17754=CARTESIAN_POINT ( 'NONE',  ( 33.58253175000000823, 56.27500000273116854, 10.91162601494192863 ) ) ;
#17759=CARTESIAN_POINT ( 'NONE',  ( -27.16883889988624290, 28.92500000273119554, -19.73931689729374028 ) ) ;
#17762=CARTESIAN_POINT ( 'NONE',  ( 5.779280353836490358E-15, 58.49999999999999289, 32.49999999999999289 ) ) ;
#17781=CARTESIAN_POINT ( 'NONE',  ( -27.16883889988624290, 43.17500000273118133, -19.73931689729374028 ) ) ;
#17786=CARTESIAN_POINT ( 'NONE',  ( 26.29305231718578995, 63.20000000000001705, -19.10302069950538240 ) ) ;
#17792=CARTESIAN_POINT ( 'NONE',  ( 27.16883889988623935, 70.57500000273118701, -19.73931689729374384 ) ) ;
#17797=CARTESIAN_POINT ( 'NONE',  ( -10.37757302488624411, 50.72500000273118559, -31.93888565452638417 ) ) ;
#17803=CARTESIAN_POINT ( 'NONE',  ( -2.092463501923844636E-15, 8.000000005462366559, -34.17252228774368916 ) ) ;
#17823=CARTESIAN_POINT ( 'NONE',  ( 20.75514604977249178, 62.07500000273118701, 28.56700777964553950 ) ) ;
#17830=CARTESIAN_POINT ( 'NONE',  ( -27.16883889988623935, 19.32500000273117280, 19.73931689729374739 ) ) ;
#17835=CARTESIAN_POINT ( 'NONE',  ( -20.08610463437156923, 44.80000000546235839, 27.64615127144130113 ) ) ;
#17843=CARTESIAN_POINT ( 'NONE',  ( 10.37757302488624767, 71.72500000273117848, 31.93888565452638417 ) ) ;
#17850=CARTESIAN_POINT ( 'NONE',  ( 33.58253175000000823, 12.02500000273117742, 10.91162601494192863 ) ) ;
#17861=CARTESIAN_POINT ( 'NONE',  ( -2.092463501923844636E-15, 27.50000000000000355, -34.17252228774368916 ) ) ;
#17874=CARTESIAN_POINT ( 'NONE',  ( 33.58253175000000113, 40.12500000273118417, -4.112674001490185761E-15 ) ) ;
#17875=DIRECTION ( 'NONE',  ( 0.000000000000000000, 0.000000000000000000, 1.000000000000000000 ) ) ;
#17876=CARTESIAN_POINT ( 'NONE',  ( -27.16883889988623935, 55.57500000273117280, 19.73931689729374739 ) ) ;
#17880=CARTESIAN_POINT ( 'NONE',  ( 20.08610463437157279, 59.80000000546235839, -27.64615127144129758 ) ) ;
#17889=CARTESIAN_POINT ( 'NONE',  ( -27.16883889988623935, 33.57500000273118701, 19.73931689729374739 ) ) ;
#17893=CARTESIAN_POINT ( 'NONE',  ( 6.277390505771533514E-15, 21.00000000546236478, 34.17252228774368916 ) ) ;
#17903=CARTESIAN_POINT ( 'NONE',  ( 33.58253175000000113, 62.22500000273119269, -10.91162601494193574 ) ) ;
#17914=CARTESIAN_POINT ( 'NONE',  ( 33.58253175000000823, 72.27500000273118985, 10.91162601494192863 ) ) ;
#17920=CARTESIAN_POINT ( 'NONE',  ( -20.75514604977248112, 63.42500000273118133, 28.56700777964554661 ) ) ;
#17921=CARTESIAN_POINT ( 'NONE',  ( -33.58253175000000113, 17.47500000273117848, 10.91162601494193929 ) ) ;
#17922=CARTESIAN_POINT ( 'NONE',  ( -2.162160676586881955E-15, 10.87500000273118417, -35.31076352940723240 ) ) ;
#17926=CARTESIAN_POINT ( 'NONE',  ( 20.75514604977249178, 1.825000002731179460, 28.56700777964553950 ) ) ;
#17928=CARTESIAN_POINT ( 'NONE',  ( -26.29305231718578995, 44.20000000000000284, 19.10302069950538595 ) ) ;
#17934=CARTESIAN_POINT ( 'NONE',  ( -2.162160676586881955E-15, 54.87500000273119127, -35.31076352940723240 ) ) ;
#17939=CARTESIAN_POINT ( 'NONE',  ( -27.16883889988624290, 22.92500000273119198, -19.73931689729374028 ) ) ;
#17954=CARTESIAN_POINT ( 'NONE',  ( -20.08610463437157989, 17.69999999999999218, -27.64615127144129758 ) ) ;
#17959=CARTESIAN_POINT ( 'NONE',  ( -27.16883889988624290, 76.92500000273120975, -19.73931689729374028 ) ) ;
#17960=CARTESIAN_POINT ( 'NONE',  ( -27.16883889988624290, 41.17500000273118133, -19.73931689729374028 ) ) ;
#17965=CARTESIAN_POINT ( 'NONE',  ( -32.50000000000000000, 61.99999999999998579, 0.000000000000000000 ) ) ;
#17969=CARTESIAN_POINT ( 'NONE',  ( 20.75514604977248467, 72.67500000273118133, -28.56700777964554305 ) ) ;
#17975=CARTESIAN_POINT ( 'NONE',  ( -33.58253175000000113, 43.12500000273118417, 0.000000000000000000 ) ) ;
#17979=CARTESIAN_POINT ( 'NONE',  ( 6.277390505771533514E-15, 7.000000005462369224, 34.17252228774368916 ) ) ;
#17997=AXIS2_PLACEMENT_3D ( 'NONE', #28450, #33781, #28789 ) ;
#18001=CARTESIAN_POINT ( 'NONE',  ( -10.37757302488624411, 60.97500000273119269, -31.93888565452638417 ) ) ;
#18005=CYLINDRICAL_SURFACE ( 'NONE', #17997, 32.50000000000000000 ) ;
#18007=CARTESIAN_POINT ( 'NONE',  ( 10.04305231718579705, 76.59999999999999432, 30.90933677959248982 ) ) ;
#18008=CARTESIAN_POINT ( 'NONE',  ( -27.16883889988624290, 12.92500000273118310, -19.73931689729374028 ) ) ;
#18012=CARTESIAN_POINT ( 'NONE',  ( 32.50000000000000711, 37.40000000546236691, 10.55989012756945122 ) ) ;
#18013=( BOUNDED_CURVE ( )  B_SPLINE_CURVE ( 2, ( #16666, #27123, #24711, #29856, #3949, #3616, #8925, #17001, #14090, #24547, #1018, #14424, #24878 ),
 .UNSPECIFIED., .F., .T. ) 
 B_SPLINE_CURVE_WITH_KNOTS ( ( 3, 2, 2, 2, 2, 2, 3 ),
 ( 0.1987179487179487336, 0.2000000000000000111, 0.2025641025641025661, 0.2051282051282051211, 0.2076923076923077038, 0.2102564102564102588, 0.2115384615384615363 ),
 .UNSPECIFIED. ) 
 CURVE ( )  GEOMETRIC_REPRESENTATION_ITEM ( )  RATIONAL_B_SPLINE_CURVE ( ( 0.9755282581475768211, 0.9755282581475770431, 1.000000000000000000, 0.9510565162951535312, 1.000000000000000000, 0.9510565162951535312, 1.000000000000000000, 0.9510565162951535312, 1.000000000000000000, 0.9510565162951535312, 1.000000000000000000, 0.9755282581475768211, 0.9755282581475768211 ) ) 
 REPRESENTATION_ITEM ( '' )  );
#18018=CARTESIAN_POINT ( 'NONE',  ( 27.16883889988623935, 66.32500000273118701, -19.73931689729374384 ) ) ;
#18024=CARTESIAN_POINT ( 'NONE',  ( 33.58253175000000113, 12.12500000273118772, -4.112674001490185761E-15 ) ) ;
#18034=CARTESIAN_POINT ( 'NONE',  ( 6.277390505771533514E-15, 32.49999999999999289, 34.17252228774368916 ) ) ;
#18039=CARTESIAN_POINT ( 'NONE',  ( 32.50000000000000000, 63.10000000000001563, -10.55989012756945833 ) ) ;
#18045=CARTESIAN_POINT ( 'NONE',  ( 25.94559702212998076, 66.99999999999998579, -20.21712673764820423 ) ) ;
#18046=CARTESIAN_POINT ( 'NONE',  ( 33.58253175000000113, 36.12500000273118417, -4.112674001490185761E-15 ) ) ;
#18047=CARTESIAN_POINT ( 'NONE',  ( 26.29305231718578995, 57.20000000000001705, -19.10302069950538240 ) ) ;
#18051=CARTESIAN_POINT ( 'NONE',  ( 26.29305231718579350, 61.30000000546238681, 19.10302069950537529 ) ) ;
#18056=CARTESIAN_POINT ( 'NONE',  ( 33.58253175000000113, 32.47500000273117138, -10.91162601494193751 ) ) ;
#18060=CARTESIAN_POINT ( 'NONE',  ( -20.08610463437156923, 24.80000000546235839, 27.64615127144130113 ) ) ;
#18069=CARTESIAN_POINT ( 'NONE',  ( -33.58253175000000113, 63.12500000273117706, 0.000000000000000000 ) ) ;
#18080=CARTESIAN_POINT ( 'NONE',  ( 33.58253175000000823, 74.27500000273117564, 10.91162601494192863 ) ) ;
#18085=CARTESIAN_POINT ( 'NONE',  ( -2.162160676586881955E-15, 58.62500000273118417, -35.31076352940723240 ) ) ;
#18086=CARTESIAN_POINT ( 'NONE',  ( 6.486482029760649416E-15, 19.87500000273119483, 35.31076352940723240 ) ) ;
#18087=CARTESIAN_POINT ( 'NONE',  ( 10.37757302488624767, 1.975000002731180926, 31.93888565452638417 ) ) ;
#18092=CARTESIAN_POINT ( 'NONE',  ( 6.486482029760649416E-15, 3.625000002731194826, 35.31076352940723240 ) ) ;
#18097=ORIENTED_EDGE ( 'NONE', *, *, #6211, .F. ) ;
#18098=CARTESIAN_POINT ( 'NONE',  ( 27.16883889988623935, 56.57500000273117990, -19.73931689729374384 ) ) ;
#18103=CARTESIAN_POINT ( 'NONE',  ( -27.16883889988623935, 27.32500000273117990, 19.73931689729374739 ) ) ;
#18106=CARTESIAN_POINT ( 'NONE',  ( 0.000000000000000000, 66.99999999999998579, 0.000000000000000000 ) ) ;
#18113=( BOUNDED_CURVE ( )  B_SPLINE_CURVE ( 2, ( #29659, #999, #6162, #21795, #13732, #32074, #3103, #670, #3428, #3593, #11158, #29495, #24202 ),
 .UNSPECIFIED., .F., .T. ) 
 B_SPLINE_CURVE_WITH_KNOTS ( ( 3, 2, 2, 2, 2, 2, 3 ),
 ( 0.2115384615384615363, 0.2128205128205128138, 0.2153846153846153966, 0.2179487179487179516, 0.2205128205128205066, 0.2230769230769230893, 0.2243589743589743668 ),
 .UNSPECIFIED. ) 
 CURVE ( )  GEOMETRIC_REPRESENTATION_ITEM ( )  RATIONAL_B_SPLINE_CURVE ( ( 0.9755282581475768211, 0.9755282581475768211, 1.000000000000000000, 0.9510565162951535312, 1.000000000000000000, 0.9510565162951535312, 1.000000000000000000, 0.9510565162951535312, 1.000000000000000000, 0.9510565162951535312, 1.000000000000000000, 0.9755282581475768211, 0.9755282581475768211 ) ) 
 REPRESENTATION_ITEM ( '' )  );
#18119=CARTESIAN_POINT ( 'NONE',  ( 26.29305231718578995, 19.20000000000000995, -19.10302069950538240 ) ) ;
#18128=CARTESIAN_POINT ( 'NONE',  ( 33.58253175000000823, 78.02500000273118985, 10.91162601494192863 ) ) ;
#18130=CARTESIAN_POINT ( 'NONE',  ( 20.75514604977248467, 34.67500000273118843, -28.56700777964554305 ) ) ;
#18136=CARTESIAN_POINT ( 'NONE',  ( 32.50000000000000711, 62.89999999999999147, 10.55989012756945122 ) ) ;
#18141=CARTESIAN_POINT ( 'NONE',  ( -10.37757302488624411, 70.97500000273120691, -31.93888565452638417 ) ) ;
#18146=CARTESIAN_POINT ( 'NONE',  ( -27.16883889988623935, 45.32500000273119412, 19.73931689729374739 ) ) ;
#18150=CARTESIAN_POINT ( 'NONE',  ( -10.04305231718578462, 6.900000005462383790, 30.90933677959249337 ) ) ;
#18169=CARTESIAN_POINT ( 'NONE',  ( 6.486482029760649416E-15, 55.87500000273118417, 35.31076352940723240 ) ) ;
#18175=CARTESIAN_POINT ( 'NONE',  ( 32.50000000000000000, 79.00000000000000000, -3.980102097228898626E-15 ) ) ;
#18176=CARTESIAN_POINT ( 'NONE',  ( 33.58253175000000113, 18.12500000273119127, -4.112674001490185761E-15 ) ) ;
#18182=CARTESIAN_POINT ( 'NONE',  ( -32.50000000000000000, 36.60000000546239818, 10.55989012756946366 ) ) ;
#18189=CARTESIAN_POINT ( 'NONE',  ( 6.486482029760649416E-15, 63.62500000273117706, 35.31076352940723240 ) ) ;
#18194=CARTESIAN_POINT ( 'NONE',  ( 10.37757302488624767, 5.725000002731183812, 31.93888565452638417 ) ) ;
#18202=DIRECTION ( 'NONE',  ( -0.8660254037844387076, 0.000000000000000000, -0.4999999999999998335 ) ) ;
#18205=CARTESIAN_POINT ( 'NONE',  ( 32.50000000000000000, 31.10000000000000497, -10.55989012756945833 ) ) ;
#18209=CARTESIAN_POINT ( 'NONE',  ( -26.02353298184806007, 67.00000000000000000, 20.33883978280647398 ) ) ;
#18219=CARTESIAN_POINT ( 'NONE',  ( 27.16883889988623935, 32.32500000273117990, -19.73931689729374384 ) ) ;
#18224=CARTESIAN_POINT ( 'NONE',  ( -26.29305231718579350, 56.30000000546238681, -19.10302069950537884 ) ) ;
#18230=CARTESIAN_POINT ( 'NONE',  ( 6.486482029760649416E-15, 35.87500000273118417, 35.31076352940723240 ) ) ;
#18234=CARTESIAN_POINT ( 'NONE',  ( -20.08610463437156923, 20.80000000546236549, 27.64615127144130113 ) ) ;
#18244=CARTESIAN_POINT ( 'NONE',  ( -20.75514604977248112, 63.42500000273118843, 28.56700777964554661 ) ) ;
#18255=CARTESIAN_POINT ( 'NONE',  ( 10.37757302488624056, 76.77500000273117564, -31.93888565452638417 ) ) ;
#18259=CARTESIAN_POINT ( 'NONE',  ( -20.75514604977248823, 54.82500000273118701, -28.56700777964554305 ) ) ;
#18260=CARTESIAN_POINT ( 'NONE',  ( -2.162160676586881955E-15, 16.87500000273120193, -35.31076352940723240 ) ) ;
#18261=CARTESIAN_POINT ( 'NONE',  ( -33.58253175000000113, 79.02500000273118985, -10.91162601494193218 ) ) ;
#18265=CARTESIAN_POINT ( 'NONE',  ( 32.50000000000000000, 73.50000000546238255, -3.980102097228898626E-15 ) ) ;
#18266=CARTESIAN_POINT ( 'NONE',  ( 31.53731130704408869, 52.00000000000002132, 11.55439184653631024 ) ) ;
#18272=CARTESIAN_POINT ( 'NONE',  ( 6.486482029760649416E-15, 55.87500000273118417, 35.31076352940723240 ) ) ;
#18279=CARTESIAN_POINT ( 'NONE',  ( -10.37757302488624411, 26.72500000273118914, -31.93888565452638417 ) ) ;
#18283=CARTESIAN_POINT ( 'NONE',  ( -20.08610463437156923, 58.29999999999999716, 27.64615127144130113 ) ) ;
#18293=CARTESIAN_POINT ( 'NONE',  ( -5.147494310547423346, 60.44874571845313227, 32.50000000000000000 ) ) ;
#18294=CARTESIAN_POINT ( 'NONE',  ( -26.29305231718578995, 14.20000000000000462, 19.10302069950538595 ) ) ;
#18300=CARTESIAN_POINT ( 'NONE',  ( -20.75514604977248112, 73.42500000273118133, 28.56700777964554661 ) ) ;
#18301=CARTESIAN_POINT ( 'NONE',  ( 6.486482029760649416E-15, 35.87500000273118417, 35.31076352940723240 ) ) ;
#18308=CARTESIAN_POINT ( 'NONE',  ( -26.29305231718579350, 57.80000000000000426, -19.10302069950537884 ) ) ;
#18309=FACE_BOUND ( 'NONE', #21270, .T. ) ;
#18313=CARTESIAN_POINT ( 'NONE',  ( 6.486482029760649416E-15, 75.87500000273119838, 35.31076352940723240 ) ) ;
#18318=CARTESIAN_POINT ( 'NONE',  ( 33.58253175000000113, 46.12500000273119127, -4.112674001490185761E-15 ) ) ;
#18319=ORIENTED_EDGE ( 'NONE', *, *, #13461, .T. ) ;
#18322=CARTESIAN_POINT ( 'NONE',  ( 32.50000000000000000, 1.600000005462365760, -10.55989012756945833 ) ) ;
#18340=CARTESIAN_POINT ( 'NONE',  ( 10.37757302488624767, 53.97500000273118559, 31.93888565452638417 ) ) ;
#18347=CARTESIAN_POINT ( 'NONE',  ( -32.50000000000000000, 78.10000000000000853, 10.55989012756946366 ) ) ;
#18348=CARTESIAN_POINT ( 'NONE',  ( -27.16883889988624290, 14.92500000273118488, -19.73931689729374028 ) ) ;
#18349=LINE ( 'NONE', #31201, #24289 ) ;
#18354=CARTESIAN_POINT ( 'NONE',  ( 26.29305231718579350, 33.30000000546239391, 19.10302069950537529 ) ) ;
#18360=CARTESIAN_POINT ( 'NONE',  ( 33.58253175000000113, 62.22500000273119269, -10.91162601494193751 ) ) ;
#18364=CARTESIAN_POINT ( 'NONE',  ( 33.58253175000000113, 8.125000002731184168, -4.112674001490185761E-15 ) ) ;
#18374=CARTESIAN_POINT ( 'NONE',  ( -20.08610463437157989, 23.70000000000000639, -27.64615127144129758 ) ) ;
#18385=CARTESIAN_POINT ( 'NONE',  ( -20.75514604977248823, 34.82500000273118701, -28.56700777964554305 ) ) ;
#18386=CARTESIAN_POINT ( 'NONE',  ( -5.147494310547423346, 64.94874572391552192, 32.50000000000000000 ) ) ;
#18390=CARTESIAN_POINT ( 'NONE',  ( -32.50000000000000000, 54.40000000546238823, -10.55989012756945478 ) ) ;
#18397=CARTESIAN_POINT ( 'NONE',  ( -27.16883889988623935, 25.57500000273120477, 19.73931689729374739 ) ) ;
#18401=CARTESIAN_POINT ( 'NONE',  ( 20.08610463437157279, 17.80000000546237615, -27.64615127144129758 ) ) ;
#18411=CARTESIAN_POINT ( 'NONE',  ( 5.779280353836490358E-15, 54.49999999999999289, 32.49999999999999289 ) ) ;
#18412=CARTESIAN_POINT ( 'NONE',  ( 10.37757302488624056, 64.52500000273118985, -31.93888565452638417 ) ) ;
#18425=CARTESIAN_POINT ( 'NONE',  ( -33.58253175000000113, 75.27500000273118985, -10.91162601494193218 ) ) ;
#18429=CARTESIAN_POINT ( 'NONE',  ( -27.16883889988623935, 53.32500000273120122, 19.73931689729374739 ) ) ;
#18431=CARTESIAN_POINT ( 'NONE',  ( 10.37757302488624767, 15.97500000273120691, 31.93888565452638417 ) ) ;
#18432=CARTESIAN_POINT ( 'NONE',  ( -27.16883889988624290, 3.175000002731187543, -19.73931689729374028 ) ) ;
#18436=CARTESIAN_POINT ( 'NONE',  ( -32.50000000000000000, 72.40000000546235981, -10.55989012756945478 ) ) ;
#18437=CARTESIAN_POINT ( 'NONE',  ( 26.02353298184809560, 52.00000000000001421, -20.33883978280646332 ) ) ;
#18443=CARTESIAN_POINT ( 'NONE',  ( 10.37757302488624056, 52.77500000273120406, -31.93888565452638417 ) ) ;
#18447=VERTEX_POINT ( 'NONE', #25757 ) ;
#18448=CARTESIAN_POINT ( 'NONE',  ( -20.75514604977248112, 21.42500000273120264, 28.56700777964554661 ) ) ;
#18451=CARTESIAN_POINT ( 'NONE',  ( -32.50000000000000000, 57.99999999999997868, 0.000000000000000000 ) ) ;
#18459=CARTESIAN_POINT ( 'NONE',  ( 20.08610463437157279, 65.80000000546237970, -27.64615127144129758 ) ) ;
#18460=CARTESIAN_POINT ( 'NONE',  ( -26.29305231718578995, 60.20000000000001705, 19.10302069950538595 ) ) ;
#18461=CARTESIAN_POINT ( 'NONE',  ( 20.08610463437158344, 18.69999999999998863, 27.64615127144129403 ) ) ;
#18466=EDGE_CURVE ( 'NONE', #25078, #11742, #2242, .T. ) ;
#18468=CARTESIAN_POINT ( 'NONE',  ( -20.75514604977248112, 75.42500000273120975, 28.56700777964554661 ) ) ;
#18470=CARTESIAN_POINT ( 'NONE',  ( 33.58253175000000113, 38.37500000273118417, -4.112674001490185761E-15 ) ) ;
#18475=CARTESIAN_POINT ( 'NONE',  ( 20.08610463437157279, 53.29999999999999716, -27.64615127144129758 ) ) ;
#18481=CARTESIAN_POINT ( 'NONE',  ( -27.16883889988624290, 71.17500000273118133, -19.73931689729374028 ) ) ;
#18485=ORIENTED_EDGE ( 'NONE', *, *, #765, .F. ) ;
#18487=CARTESIAN_POINT ( 'NONE',  ( -20.75514604977248823, 40.82500000273120122, -28.56700777964554305 ) ) ;
#18489=EDGE_LOOP ( 'NONE', ( #24747, #30085, #5972, #8706, #24538, #4836, #21806, #28257, #6305, #33335, #30995, #31625, #26865, #3601, #21555, #26069, #10535, #32581, #29034 ) ) ;
#18492=CARTESIAN_POINT ( 'NONE',  ( 32.50000000000000711, 5.400000005462376684, 10.55989012756945122 ) ) ;
#18511=CARTESIAN_POINT ( 'NONE',  ( 20.75514604977248467, 58.67500000273118843, -28.56700777964554305 ) ) ;
#18517=CARTESIAN_POINT ( 'NONE',  ( 10.04305231718578817, 75.40000000000000568, -30.90933677959249337 ) ) ;
#18518=CARTESIAN_POINT ( 'NONE',  ( 20.75514604977248467, 18.42500000273117422, -28.56700777964554305 ) ) ;
#18522=CARTESIAN_POINT ( 'NONE',  ( -26.29305231718579350, 38.30000000546239391, -19.10302069950537884 ) ) ;
#18527=CARTESIAN_POINT ( 'NONE',  ( -20.75514604977248823, 60.82500000273121543, -28.56700777964554305 ) ) ;
#18531=CARTESIAN_POINT ( 'NONE',  ( -2.162160676586881955E-15, 6.625000002731173510, -35.31076352940723240 ) ) ;
#18539=CARTESIAN_POINT ( 'NONE',  ( 5.779280353836490358E-15, 53.00000000546238255, 32.49999999999999289 ) ) ;
#18541=CARTESIAN_POINT ( 'NONE',  ( -20.08610463437156923, 20.30000000000000071, 27.64615127144130113 ) ) ;
#18545=CARTESIAN_POINT ( 'NONE',  ( -28.37133278852432738, 66.99999999999998579, 17.03823453610152683 ) ) ;
#18553=CARTESIAN_POINT ( 'NONE',  ( 10.37757302488624056, 34.52500000273118985, -31.93888565452638417 ) ) ;
#18559=CARTESIAN_POINT ( 'NONE',  ( -26.29305231718578995, 54.70000000546236407, 19.10302069950538595 ) ) ;
#18569=CARTESIAN_POINT ( 'NONE',  ( 10.37757302488624056, 28.77500000273118630, -31.93888565452638417 ) ) ;
#18573=CARTESIAN_POINT ( 'NONE',  ( -10.04305231718578462, 16.90000000546236336, 30.90933677959249337 ) ) ;
#18583=CARTESIAN_POINT ( 'NONE',  ( 27.16883889988623935, 62.32500000273120833, -19.73931689729374384 ) ) ;
#18592=CARTESIAN_POINT ( 'NONE',  ( -40.00000000000000711, 52.00000000000000711, 23.09401076758504345 ) ) ;
#18593=CARTESIAN_POINT ( 'NONE',  ( 33.58253175000000113, 72.47500000273119269, -10.91162601494193751 ) ) ;
#18597=CARTESIAN_POINT ( 'NONE',  ( 20.75514604977249178, 51.82500000273120122, 28.56700777964553950 ) ) ;
#18598=CARTESIAN_POINT ( 'NONE',  ( 27.16883889988624290, 18.17500000273118843, 19.73931689729373673 ) ) ;
#18599=CARTESIAN_POINT ( 'NONE',  ( -2.162160676586881955E-15, 6.875000002731180615, -35.31076352940723240 ) ) ;
#18604=CARTESIAN_POINT ( 'NONE',  ( -32.50000000000000000, 76.60000000546239107, 10.55989012756946366 ) ) ;
#18605=CARTESIAN_POINT ( 'NONE',  ( 10.64935084019646538, 52.00000000000002132, -30.92824909085711838 ) ) ;
#18612=CARTESIAN_POINT ( 'NONE',  ( -2.162160676586881955E-15, 46.87500000273118417, -35.31076352940723240 ) ) ;
#18617=CARTESIAN_POINT ( 'NONE',  ( 10.37757302488624056, 22.52500000273117919, -31.93888565452638417 ) ) ;
#18634=CARTESIAN_POINT ( 'NONE',  ( 10.04305231718578817, 15.40000000000001101, -30.90933677959249337 ) ) ;
#18640=CARTESIAN_POINT ( 'NONE',  ( 33.58253175000000823, 72.02500000273118985, 10.91162601494192863 ) ) ;
#18641=CARTESIAN_POINT ( 'NONE',  ( -33.58253175000000113, 37.47500000273118559, 10.91162601494193929 ) ) ;
#18646=CARTESIAN_POINT ( 'NONE',  ( -32.50000000000000000, 51.89999999999998437, -10.55989012756945478 ) ) ;
#18651=CARTESIAN_POINT ( 'NONE',  ( -2.162160676586881955E-15, 66.87500000273119838, -35.31076352940723240 ) ) ;
#18656=CARTESIAN_POINT ( 'NONE',  ( 27.16883889988624290, 45.92500000273118133, 19.73931689729373673 ) ) ;
#18657=DIRECTION ( 'NONE',  ( 0.000000000000000000, 1.000000000000000000, 0.000000000000000000 ) ) ;
#18661=CARTESIAN_POINT ( 'NONE',  ( -26.29305231718578995, 4.700000005462376507, 19.10302069950538595 ) ) ;
#18676=CYLINDRICAL_SURFACE ( 'NONE', #4464, 32.50000000000000000 ) ;
#18680=CARTESIAN_POINT ( 'NONE',  ( -20.75514604977248823, 55.07500000273117990, -28.56700777964554305 ) ) ;
#18687=CARTESIAN_POINT ( 'NONE',  ( -20.08610463437156923, 70.30000000000001137, 27.64615127144130113 ) ) ;
#18688=CARTESIAN_POINT ( 'NONE',  ( 6.486482029760649416E-15, 17.62500000273117351, 35.31076352940723240 ) ) ;
#18695=ORIENTED_EDGE ( 'NONE', *, *, #30881, .T. ) ;
#18696=CARTESIAN_POINT ( 'NONE',  ( 20.75514604977249178, 61.82500000273116569, 28.56700777964553950 ) ) ;
#18697=EDGE_CURVE ( 'NONE', #32671, #33362, #2466, .T. ) ;
#18701=CARTESIAN_POINT ( 'NONE',  ( -2.162160676586881955E-15, 2.625000002731183724, -35.31076352940723240 ) ) ;
#18709=CARTESIAN_POINT ( 'NONE',  ( -10.04305231718578462, 52.90000000546239534, 30.90933677959249337 ) ) ;
#18712=CARTESIAN_POINT ( 'NONE',  ( -32.50000000000000000, 25.89999999999999503, -10.55989012756945478 ) ) ;
#18716=CARTESIAN_POINT ( 'NONE',  ( -32.17340636219239514, 66.99999999999997158, 8.405285767817538556 ) ) ;
#18723=CARTESIAN_POINT ( 'NONE',  ( 13.42768774669677612, 66.99999999999998579, -30.32522641246981365 ) ) ;
#18725=CARTESIAN_POINT ( 'NONE',  ( -10.37757302488624411, 32.72500000273119269, -31.93888565452638417 ) ) ;
#18730=CARTESIAN_POINT ( 'NONE',  ( 32.50000000000000000, 53.50000000546238965, -3.980102097228898626E-15 ) ) ;
#18735=CARTESIAN_POINT ( 'NONE',  ( -20.75514604977248823, 27.07500000273119412, -28.56700777964554305 ) ) ;
#18739=CARTESIAN_POINT ( 'NONE',  ( 26.29305231718578995, 19.70000000546238894, -19.10302069950538240 ) ) ;
#18749=CARTESIAN_POINT ( 'NONE',  ( 33.58253175000000113, 52.12500000273119838, -4.112674001490185761E-15 ) ) ;
#18758=CARTESIAN_POINT ( 'NONE',  ( -20.75514604977248112, 65.67500000273118133, 28.56700777964554661 ) ) ;
#18762=CARTESIAN_POINT ( 'NONE',  ( 6.486482029760649416E-15, 55.62500000273119838, 35.31076352940723240 ) ) ;
#18763=CARTESIAN_POINT ( 'NONE',  ( -33.58253175000000113, 13.27500000273118097, -10.91162601494193218 ) ) ;
#18764=CARTESIAN_POINT ( 'NONE',  ( -10.37757302488624411, 6.975000002731198911, -31.93888565452638417 ) ) ;
#18768=CARTESIAN_POINT ( 'NONE',  ( -32.50000000000000000, 74.60000000546234844, 10.55989012756946366 ) ) ;
#18775=CARTESIAN_POINT ( 'NONE',  ( -27.16883889988624290, 45.17500000273118133, -19.73931689729374028 ) ) ;
#18780=CARTESIAN_POINT ( 'NONE',  ( 10.37757302488624056, 16.52500000273120051, -31.93888565452638417 ) ) ;
#18789=CARTESIAN_POINT ( 'NONE',  ( 0.000000000000000000, 52.00000000000000711, 32.50000000000000000 ) ) ;
#18792=CARTESIAN_POINT ( 'NONE',  ( -32.50000000000000000, 63.99999999999998579, 0.000000000000000000 ) ) ;
#18795=CARTESIAN_POINT ( 'NONE',  ( -20.08610463437156923, 60.29999999999997584, 27.64615127144130113 ) ) ;
#18796=CARTESIAN_POINT ( 'NONE',  ( -2.092463501923844636E-15, 7.499999999999995559, -34.17252228774368916 ) ) ;
#18802=CARTESIAN_POINT ( 'NONE',  ( 33.58253175000000113, 72.12500000273118417, -4.112674001490185761E-15 ) ) ;
#18803=CARTESIAN_POINT ( 'NONE',  ( -33.58253175000000113, 39.37500000273118417, 0.000000000000000000 ) ) ;
#18809=CARTESIAN_POINT ( 'NONE',  ( -20.08610463437156923, 52.30000000000001137, 27.64615127144130113 ) ) ;
#18815=CARTESIAN_POINT ( 'NONE',  ( -2.162160676586881955E-15, 68.87500000273118417, -35.31076352940723240 ) ) ;
#18820=CARTESIAN_POINT ( 'NONE',  ( -27.16883889988624290, 38.92500000273117422, -19.73931689729374028 ) ) ;
#18826=CARTESIAN_POINT ( 'NONE',  ( -26.29305231718578995, 0.7000000054623728429, 19.10302069950538595 ) ) ;
#18842=CARTESIAN_POINT ( 'NONE',  ( 10.37757302488624056, 56.77500000273121117, -31.93888565452638417 ) ) ;
#18848=CARTESIAN_POINT ( 'NONE',  ( -20.08610463437157989, 71.69999999999997442, -27.64615127144129758 ) ) ;
#18849=CARTESIAN_POINT ( 'NONE',  ( 33.58253175000000113, 6.225000002731185589, -10.91162601494193751 ) ) ;
#18858=CARTESIAN_POINT ( 'NONE',  ( -10.37757302488623701, 55.52500000273118275, 31.93888565452638417 ) ) ;
#18862=CARTESIAN_POINT ( 'NONE',  ( 33.58253175000000113, 2.125000002731192161, -4.112674001490185761E-15 ) ) ;
#18871=CARTESIAN_POINT ( 'NONE',  ( -2.092463501923844636E-15, 25.50000000000001066, -34.17252228774368916 ) ) ;
#18886=CARTESIAN_POINT ( 'NONE',  ( -27.16883889988624290, 30.92500000273119909, -19.73931689729374028 ) ) ;
#18887=CARTESIAN_POINT ( 'NONE',  ( -32.50000000000000000, 56.40000000546237402, -10.55989012756945300 ) ) ;
#18892=CARTESIAN_POINT ( 'NONE',  ( -10.04305231718579172, 54.10000000546237686, -30.90933677959248982 ) ) ;
#18903=CARTESIAN_POINT ( 'NONE',  ( 10.04305231718579705, 19.10000000546237331, 30.90933677959248982 ) ) ;
#18914=CARTESIAN_POINT ( 'NONE',  ( 20.75514604977249178, 53.82500000273119412, 28.56700777964553950 ) ) ;
#18919=CARTESIAN_POINT ( 'NONE',  ( -10.04305231718578462, 66.90000000546238823, 30.90933677959249337 ) ) ;
#18923=CARTESIAN_POINT ( 'NONE',  ( 6.486482029760649416E-15, 67.87500000273116996, 35.31076352940723240 ) ) ;
#18930=CARTESIAN_POINT ( 'NONE',  ( -33.58253175000000113, 55.02500000273118985, -10.91162601494193218 ) ) ;
#18931=CARTESIAN_POINT ( 'NONE',  ( -2.162160676586881955E-15, 10.87500000273118417, -35.31076352940723240 ) ) ;
#18932=CARTESIAN_POINT ( 'NONE',  ( 20.75514604977248467, 62.67500000273117422, -28.56700777964554305 ) ) ;
#18935=EDGE_CURVE ( 'NONE', #31633, #5766, #27952, .T. ) ;
#18937=CARTESIAN_POINT ( 'NONE',  ( -10.04305231718579172, 76.10000000546239107, -30.90933677959248982 ) ) ;
#18944=CARTESIAN_POINT ( 'NONE',  ( -33.58253175000000113, 49.47500000273118559, 10.91162601494193929 ) ) ;
#18949=CARTESIAN_POINT ( 'NONE',  ( 20.75514604977249178, 19.82500000273119412, 28.56700777964553950 ) ) ;
#18964=CARTESIAN_POINT ( 'NONE',  ( 10.04305231718579705, 8.599999999999981881, 30.90933677959248982 ) ) ;
#18970=CARTESIAN_POINT ( 'NONE',  ( -10.37757302488624411, 74.72500000273117848, -31.93888565452638417 ) ) ;
#18971=CARTESIAN_POINT ( 'NONE',  ( -33.58253175000000113, 27.37500000273117351, 0.000000000000000000 ) ) ;
#18977=CARTESIAN_POINT ( 'NONE',  ( 26.29305231718578995, 57.20000000000001705, -19.10302069950538240 ) ) ;
#18982=CARTESIAN_POINT ( 'NONE',  ( -33.58253175000000113, 65.27500000273117564, -10.91162601494193218 ) ) ;
#18988=CARTESIAN_POINT ( 'NONE',  ( 33.58253175000000823, 40.02500000273119696, 10.91162601494192863 ) ) ;
#19004=CARTESIAN_POINT ( 'NONE',  ( 20.08610463437158344, 53.20000000546237118, 27.64615127144129403 ) ) ;
#19009=CARTESIAN_POINT ( 'NONE',  ( 10.37757302488624767, 47.97500000273117848, 31.93888565452638417 ) ) ;
#19018=CARTESIAN_POINT ( 'NONE',  ( -26.29305231718578995, 72.20000000000000284, 19.10302069950538595 ) ) ;
#19019=CARTESIAN_POINT ( 'NONE',  ( -27.16883889988623935, 11.32500000273119234, 19.73931689729374739 ) ) ;
#19022=CARTESIAN_POINT ( 'NONE',  ( 1.093617666956751375E-13, 60.00000000546238255, -32.50000000000000711 ) ) ;
#19028=CARTESIAN_POINT ( 'NONE',  ( 27.16883889988623935, 54.32500000273120122, -19.73931689729374384 ) ) ;
#19033=CARTESIAN_POINT ( 'NONE',  ( 6.486482029760649416E-15, 1.625000002731185944, 35.31076352940723240 ) ) ;
#19043=CARTESIAN_POINT ( 'NONE',  ( 26.29305231718578995, 25.19999999999998508, -19.10302069950538240 ) ) ;
#19054=CARTESIAN_POINT ( 'NONE',  ( 20.75514604977248467, 30.42500000273117777, -28.56700777964554305 ) ) ;
#19055=CARTESIAN_POINT ( 'NONE',  ( -40.00000000000000711, 52.00000000000000711, 23.09401076758504345 ) ) ;
#19059=CARTESIAN_POINT ( 'NONE',  ( -32.50000000000000000, 46.40000000546238113, -10.55989012756945478 ) ) ;
#19064=CARTESIAN_POINT ( 'NONE',  ( 10.37757302488624056, 78.52500000273120406, -31.93888565452638417 ) ) ;
#19069=CARTESIAN_POINT ( 'NONE',  ( -2.092463501923844636E-15, 16.00000000546237544, -34.17252228774368916 ) ) ;
#19074=EDGE_CURVE ( 'NONE', #22688, #10580, #20405, .T. ) ;
#19087=CARTESIAN_POINT ( 'NONE',  ( -27.16883889988624290, 69.17500000273118133, -19.73931689729374028 ) ) ;
#19088=ORIENTED_EDGE ( 'NONE', *, *, #24946, .T. ) ;
#19093=CARTESIAN_POINT ( 'NONE',  ( -33.58253175000000113, 45.22500000273117848, 10.91162601494193929 ) ) ;
#19094=CARTESIAN_POINT ( 'NONE',  ( 20.75514604977248467, 10.67500000273119021, -28.56700777964554305 ) ) ;
#19095=CARTESIAN_POINT ( 'NONE',  ( -2.162160676586882350E-15, 60.87500000273117706, -35.31076352940722529 ) ) ;
#19099=CARTESIAN_POINT ( 'NONE',  ( 20.08610463437157279, 65.80000000546237970, -27.64615127144129758 ) ) ;
#19105=CARTESIAN_POINT ( 'NONE',  ( -33.58253175000000113, 49.27500000273118985, -10.91162601494193218 ) ) ;
#19111=CARTESIAN_POINT ( 'NONE',  ( 27.16883889988624290, 15.92500000273118488, 19.73931689729373673 ) ) ;
#19120=DIRECTION ( 'NONE',  ( 0.000000000000000000, 0.000000000000000000, 1.000000000000000000 ) ) ;
#19127=CARTESIAN_POINT ( 'NONE',  ( -20.08610463437156923, 10.30000000000000782, 27.64615127144130113 ) ) ;
#19133=CARTESIAN_POINT ( 'NONE',  ( 10.37757302488624767, 63.72500000273119269, 31.93888565452638417 ) ) ;
#19134=CARTESIAN_POINT ( 'NONE',  ( -33.58253175000000113, 27.47500000273118204, 10.91162601494193929 ) ) ;
#19135=CARTESIAN_POINT ( 'NONE',  ( -2.162160676586881955E-15, 16.87500000273120193, -35.31076352940723240 ) ) ;
#19142=CARTESIAN_POINT ( 'NONE',  ( 10.04305231718579705, 52.60000000000002274, 30.90933677959248982 ) ) ;
#19147=CARTESIAN_POINT ( 'NONE',  ( 33.58253175000000113, 66.37500000273121259, -4.112674001490185761E-15 ) ) ;
#19152=CARTESIAN_POINT ( 'NONE',  ( -10.37757302488624411, 34.72500000273119269, -31.93888565452638417 ) ) ;
#19175=CARTESIAN_POINT ( 'NONE',  ( 20.75514604977248467, 46.67500000273118133, -28.56700777964554305 ) ) ;
#19180=CARTESIAN_POINT ( 'NONE',  ( 10.04305231718579705, 74.59999999999998010, 30.90933677959248982 ) ) ;
#19181=CARTESIAN_POINT ( 'NONE',  ( 6.486482029760649416E-15, 7.625000002731185056, 35.31076352940723240 ) ) ;
#19190=CARTESIAN_POINT ( 'NONE',  ( -27.16883889988623935, 55.32500000273120122, 19.73931689729374739 ) ) ;
#19199=DIRECTION ( 'NONE',  ( 0.000000000000000000, 1.000000000000000000, 0.000000000000000000 ) ) ;
#19203=PRODUCT_DEFINITION_FORMATION_WITH_SPECIFIED_SOURCE ( 'ANY', '', #7096, .NOT_KNOWN. ) ;
#19213=B_SPLINE_CURVE_WITH_KNOTS ( 'NONE', 3,
 ( #28881, #42, #16028, #21007, #5719, #13103, #18605, #10363, #23409, #20841, #26314, #10530, #31456, #26144, #2803, #28540, #7612, #12933, #16197, #18437, #26483, #13270, #21345, #25973, #10199, #33698, #7950, #2977, #13446, #23745, #8277, #23913, #209, #5036, #5379, #31286, #15858, #5547, #20679, #10697, #2640, #7779, #18266, #21178 ),
 .UNSPECIFIED., .F., .F.,
 ( 4, 2, 2, 2, 2, 2, 2, 2, 2, 2, 2, 2, 2, 2, 2, 2, 2, 2, 2, 2, 2, 4 ),
 ( 0.000000000000000000, 0.004057857163981401158, 0.008115714327962802316, 0.01217357149194420000, 0.01420250007393489972, 0.01623142865592559769, 0.02028928581990698324, 0.02231821440189768121, 0.02434714298388837572, 0.02840500014786977862, 0.03246285731185117457, 0.03652071447583257052, 0.03854964305782326156, 0.04057857163981395260, 0.04463642880379534855, 0.04869428596777673757, 0.05072321454976744248, 0.05275214313175814740, 0.05681000029573955029, 0.05883892887773024827, 0.06086785745972094624, 0.06492571462370234914 ),
 .UNSPECIFIED. ) ;
#19219=CARTESIAN_POINT ( 'NONE',  ( 20.75514604977249178, 27.82500000273116925, 28.56700777964553950 ) ) ;
#19225=CARTESIAN_POINT ( 'NONE',  ( 6.277390505771533514E-15, 47.00000000546238965, 34.17252228774368916 ) ) ;
#19229=CARTESIAN_POINT ( 'NONE',  ( 6.486482029760649416E-15, 77.62500000273121259, 35.31076352940723240 ) ) ;
#19234=CARTESIAN_POINT ( 'NONE',  ( -32.50000000000000000, 8.500000005462373664, 0.000000000000000000 ) ) ;
#19249=CARTESIAN_POINT ( 'NONE',  ( -1.778240108872766143E-15, 59.50000000000000711, -32.49999999999999289 ) ) ;
#19250=CARTESIAN_POINT ( 'NONE',  ( 27.16883889988624290, 68.17500000273118133, 19.73931689729373673 ) ) ;
#19255=CARTESIAN_POINT ( 'NONE',  ( 27.16883889988624290, 45.92500000273118133, 19.73931689729373673 ) ) ;
#19256=CARTESIAN_POINT ( 'NONE',  ( -20.75514604977248823, 9.075000002731183457, -28.56700777964554305 ) ) ;
#19257=CARTESIAN_POINT ( 'NONE',  ( -33.58253175000000113, 65.37500000273121259, 0.000000000000000000 ) ) ;
#19261=CARTESIAN_POINT ( 'NONE',  ( -32.50000000000000000, 70.50000000546239676, 0.000000000000000000 ) ) ;
#19268=CARTESIAN_POINT ( 'NONE',  ( -20.75514604977248112, 45.67500000273119554, 28.56700777964554661 ) ) ;
#19274=CARTESIAN_POINT ( 'NONE',  ( -20.75514604977248112, 17.42500000273117777, 28.56700777964554661 ) ) ;
#19289=CARTESIAN_POINT ( 'NONE',  ( 32.50000000000000000, 13.09999999999999432, -10.55989012756945833 ) ) ;
#19295=CARTESIAN_POINT ( 'NONE',  ( -33.58253175000000113, 69.12500000273118417, 0.000000000000000000 ) ) ;
#19296=CARTESIAN_POINT ( 'NONE',  ( -27.16883889988623935, 31.57500000273118346, 19.73931689729374739 ) ) ;
#19297=CARTESIAN_POINT ( 'NONE',  ( -20.75514604977248112, 15.67500000273117600, 28.56700777964554661 ) ) ;
#19305=CARTESIAN_POINT ( 'NONE',  ( -10.04305231718579172, 47.60000000000001563, -30.90933677959248982 ) ) ;
#19311=CARTESIAN_POINT ( 'NONE',  ( -27.16883889988624290, 65.17500000273116711, -19.73931689729374028 ) ) ;
#19312=CARTESIAN_POINT ( 'NONE',  ( -5.147494310547423346, 62.44874571845315359, 32.50000000000000000 ) ) ;
#19316=CARTESIAN_POINT ( 'NONE',  ( 20.75514604977249178, 35.82500000273117990, 28.56700777964553950 ) ) ;
#19332=CARTESIAN_POINT ( 'NONE',  ( -5.147494310547423346, 54.94874572391554324, 32.50000000000000000 ) ) ;
#19337=CARTESIAN_POINT ( 'NONE',  ( 10.37757302488624056, 46.77500000273120406, -31.93888565452638417 ) ) ;
#19346=CARTESIAN_POINT ( 'NONE',  ( -10.04305231718578462, 66.40000000000000568, 30.90933677959249337 ) ) ;
#19347=CARTESIAN_POINT ( 'NONE',  ( 6.486482029760649416E-15, 9.625000002731178839, 35.31076352940723240 ) ) ;
#19357=CARTESIAN_POINT ( 'NONE',  ( -20.75514604977248112, 53.42500000273117422, 28.56700777964554661 ) ) ;
#19358=CARTESIAN_POINT ( 'NONE',  ( 33.58253175000000823, 28.27500000273118985, 10.91162601494192863 ) ) ;
#19384=CARTESIAN_POINT ( 'NONE',  ( -18.68038058909792554, 52.00000000000000000, 27.25458793344659369 ) ) ;
#19385=CARTESIAN_POINT ( 'NONE',  ( 20.75514604977249178, 25.82500000273117280, 28.56700777964553950 ) ) ;
#19386=CARTESIAN_POINT ( 'NONE',  ( -10.04305231718579172, 56.10000000546237686, -30.90933677959248982 ) ) ;
#19391=CARTESIAN_POINT ( 'NONE',  ( 26.29305231718578995, 47.70000000546238539, -19.10302069950538240 ) ) ;
#19395=CARTESIAN_POINT ( 'NONE',  ( 20.75514604977248467, 78.42500000273116711, -28.56700777964554305 ) ) ;
#19400=CARTESIAN_POINT ( 'NONE',  ( 32.50000000000000000, 9.600000005462375086, -10.55989012756945833 ) ) ;
#19401=( BOUNDED_CURVE ( )  B_SPLINE_CURVE ( 2, ( #2300, #7450, #33707, #33355, #15355, #15180, #12772, #2474, #28044, #20686, #15528, #10369, #25645 ),
 .UNSPECIFIED., .F., .T. ) 
 B_SPLINE_CURVE_WITH_KNOTS ( ( 3, 2, 2, 2, 2, 2, 3 ),
 ( 0.2371794871794871973, 0.2384615384615384748, 0.2410256410256410298, 0.2435897435897435848, 0.2461538461538461675, 0.2487179487179487225, 0.2500000000000000000 ),
 .UNSPECIFIED. ) 
 CURVE ( )  GEOMETRIC_REPRESENTATION_ITEM ( )  RATIONAL_B_SPLINE_CURVE ( ( 0.9755282581475768211, 0.9755282581475770431, 1.000000000000000000, 0.9510565162951535312, 1.000000000000000000, 0.9510565162951535312, 1.000000000000000000, 0.9510565162951535312, 1.000000000000000000, 0.9510565162951535312, 1.000000000000000000, 0.9755282581475768211, 0.9755282581475768211 ) ) 
 REPRESENTATION_ITEM ( '' )  );
#19410=CARTESIAN_POINT ( 'NONE',  ( -26.29305231718579350, 33.79999999999998295, -19.10302069950537884 ) ) ;
#19417=DIRECTION ( 'NONE',  ( -1.000000000000000000, 0.000000000000000000, 0.000000000000000000 ) ) ;
#19418=CARTESIAN_POINT ( 'NONE',  ( 33.58253175000000113, 68.37500000273121259, -4.112674001490185761E-15 ) ) ;
#19423=CARTESIAN_POINT ( 'NONE',  ( 33.58253175000000113, 48.22500000273119269, -10.91162601494193751 ) ) ;
#19424=CARTESIAN_POINT ( 'NONE',  ( -27.16883889988624290, 9.175000002731179549, -19.73931689729374028 ) ) ;
#19425=CARTESIAN_POINT ( 'NONE',  ( -20.75514604977248823, 61.07500000273119412, -28.56700777964554305 ) ) ;
#19429=CARTESIAN_POINT ( 'NONE',  ( 10.04305231718578817, 67.90000000546238823, -30.90933677959249337 ) ) ;
#19437=CARTESIAN_POINT ( 'NONE',  ( 27.16883889988624290, 38.17500000273120264, 19.73931689729373673 ) ) ;
#19439=CARTESIAN_POINT ( 'NONE',  ( 20.08610463437158344, 27.20000000546237118, 27.64615127144129403 ) ) ;
#19441=CARTESIAN_POINT ( 'NONE',  ( 10.37757302488624056, 8.525000002731195181, -31.93888565452638417 ) ) ;
#19450=DIRECTION ( 'NONE',  ( -0.8660254037844387076, 0.000000000000000000, -0.4999999999999998335 ) ) ;
#19452=COLOUR_RGB ( '', 0.72549020, 0.75294118, 0.79215686) ;
#19459=CARTESIAN_POINT ( 'NONE',  ( 26.29305231718578995, 9.199999999999999289, -19.10302069950538240 ) ) ;
#19465=CARTESIAN_POINT ( 'NONE',  ( 27.16883889988623935, 64.32500000273121543, -19.73931689729374384 ) ) ;
#19466=CARTESIAN_POINT ( 'NONE',  ( -33.58253175000000113, 29.37500000273117351, 0.000000000000000000 ) ) ;
#19467=CARTESIAN_POINT ( 'NONE',  ( -33.58253175000000113, 15.27500000273118985, -10.91162601494193218 ) ) ;
#19472=CARTESIAN_POINT ( 'NONE',  ( -32.50000000000000000, 48.00000000000000000, 0.000000000000000000 ) ) ;
#19478=CARTESIAN_POINT ( 'NONE',  ( -33.58253175000000113, 57.37500000273119838, 0.000000000000000000 ) ) ;
#19482=ORIENTED_EDGE ( 'NONE', *, *, #14265, .F. ) ;
#19483=CARTESIAN_POINT ( 'NONE',  ( 20.75514604977248467, 36.42500000273118843, -28.56700777964554305 ) ) ;
#19493=ADVANCED_FACE ( 'NONE', ( #19514 ), #11285, .F. ) ;
#19506=CARTESIAN_POINT ( 'NONE',  ( 20.75514604977249178, 52.07500000273119412, 28.56700777964553950 ) ) ;
#19511=CARTESIAN_POINT ( 'NONE',  ( 32.50000000000000000, 67.10000000000000853, -10.55989012756945833 ) ) ;
#19514=FACE_OUTER_BOUND ( 'NONE', #8915, .T. ) ;
#19516=CARTESIAN_POINT ( 'NONE',  ( -32.50000000000000000, 65.99999999999998579, 0.000000000000000000 ) ) ;
#19521=CARTESIAN_POINT ( 'NONE',  ( 20.75514604977248467, 56.42500000273120264, -28.56700777964554305 ) ) ;
#19522=CARTESIAN_POINT ( 'NONE',  ( 27.16883889988624290, 26.17500000273119554, 19.73931689729373673 ) ) ;
#19537=CARTESIAN_POINT ( 'NONE',  ( 27.16883889988624290, 55.92500000273119554, 19.73931689729373673 ) ) ;
#19553=CARTESIAN_POINT ( 'NONE',  ( 20.75514604977248467, 26.42500000273118843, -28.56700777964554305 ) ) ;
#19558=CARTESIAN_POINT ( 'NONE',  ( 6.277390505771533514E-15, 51.00000000546238255, 34.17252228774368916 ) ) ;
#19559=CARTESIAN_POINT ( 'NONE',  ( 5.779280353836490358E-15, 59.00000000546238255, 32.49999999999999289 ) ) ;
#19562=CARTESIAN_POINT ( 'NONE',  ( -10.37757302488623701, 75.52500000273120406, 31.93888565452638417 ) ) ;
#19568=CARTESIAN_POINT ( 'NONE',  ( -32.50000000000000000, 12.40000000546237224, -10.55989012756945478 ) ) ;
#19578=CARTESIAN_POINT ( 'NONE',  ( 10.04305231718578817, 37.40000000000000568, -30.90933677959249337 ) ) ;
#19590=CARTESIAN_POINT ( 'NONE',  ( -10.37757302488623701, 49.52500000273117564, 31.93888565452638417 ) ) ;
#19591=CARTESIAN_POINT ( 'NONE',  ( 27.16883889988623935, 4.575000002731186122, -19.73931689729374384 ) ) ;
#19592=CARTESIAN_POINT ( 'NONE',  ( -33.58253175000000113, 61.47500000273118559, 10.91162601494193929 ) ) ;
#19596=CARTESIAN_POINT ( 'NONE',  ( -10.04305231718578462, 64.90000000546237402, 30.90933677959249337 ) ) ;
#19600=CARTESIAN_POINT ( 'NONE',  ( -5.147494310547423346, 54.44874571845314648, 32.50000000000000000 ) ) ;
#19603=CARTESIAN_POINT ( 'NONE',  ( -10.37757302488624411, 38.97500000273117138, -31.93888565452638417 ) ) ;
#19605=CARTESIAN_POINT ( 'NONE',  ( 32.50000000000000711, 29.40000000546239178, 10.55989012756945122 ) ) ;
#19609=VERTEX_POINT ( 'NONE', #19022 ) ;
#19614=CARTESIAN_POINT ( 'NONE',  ( 27.16883889988623935, 66.32500000273118701, -19.73931689729374384 ) ) ;
#19621=DIRECTION ( 'NONE',  ( 0.000000000000000000, 1.000000000000000000, 0.000000000000000000 ) ) ;
#19624=CARTESIAN_POINT ( 'NONE',  ( -10.04305231718578462, 6.400000000000003020, 30.90933677959249337 ) ) ;
#19629=CARTESIAN_POINT ( 'NONE',  ( -33.58253175000000113, 67.02500000273117564, -10.91162601494193218 ) ) ;
#19630=CARTESIAN_POINT ( 'NONE',  ( 33.58253175000000113, 30.47500000273117493, -10.91162601494193751 ) ) ;
#19631=CARTESIAN_POINT ( 'NONE',  ( -20.75514604977248112, 13.67500000273118133, 28.56700777964554661 ) ) ;
#19638=CARTESIAN_POINT ( 'NONE',  ( 20.08610463437158344, 46.70000000000000284, 27.64615127144129403 ) ) ;
#19644=CARTESIAN_POINT ( 'NONE',  ( 27.16883889988624290, 62.17500000273119554, 19.73931689729373673 ) ) ;
#19648=VERTEX_POINT ( 'NONE', #14195 ) ;
#19649=CARTESIAN_POINT ( 'NONE',  ( 33.58253175000000113, 28.22500000273119269, -10.91162601494193751 ) ) ;
#19670=CARTESIAN_POINT ( 'NONE',  ( 6.486482029760649416E-15, 49.87500000273119838, 35.31076352940723240 ) ) ;
#19676=CARTESIAN_POINT ( 'NONE',  ( -20.08610463437157989, 63.69999999999998863, -27.64615127144129758 ) ) ;
#19681=CARTESIAN_POINT ( 'NONE',  ( 27.16883889988623935, 78.57500000273120122, -19.73931689729374384 ) ) ;
#19685=ORIENTED_EDGE ( 'NONE', *, *, #23429, .F. ) ;
#19686=CARTESIAN_POINT ( 'NONE',  ( -20.75514604977248112, 47.42500000273118843, 28.56700777964554661 ) ) ;
#19687=CARTESIAN_POINT ( 'NONE',  ( -33.58253175000000113, 21.37500000273119483, 0.000000000000000000 ) ) ;
#19691=DIRECTION ( 'NONE',  ( 0.000000000000000000, 1.000000000000000000, 0.000000000000000000 ) ) ;
#19702=CARTESIAN_POINT ( 'NONE',  ( 6.486482029760648627E-15, 55.62500000273119838, 35.31076352940722529 ) ) ;
#19716=CARTESIAN_POINT ( 'NONE',  ( -20.75514604977248823, 18.82500000273119767, -28.56700777964554305 ) ) ;
#19718=CARTESIAN_POINT ( 'NONE',  ( 5.147494310547535257, 55.94874572391554324, -32.49999999999996447 ) ) ;
#19721=CARTESIAN_POINT ( 'NONE',  ( 26.29305231718579350, 45.30000000546237260, 19.10302069950537529 ) ) ;
#19729=CARTESIAN_POINT ( 'NONE',  ( 33.58253175000000823, 78.02500000273118985, 10.91162601494192863 ) ) ;
#19734=CARTESIAN_POINT ( 'NONE',  ( 32.50000000000000000, 11.60000000546238397, -10.55989012756945833 ) ) ;
#19743=CARTESIAN_POINT ( 'NONE',  ( 6.277390505771533514E-15, 34.49999999999998579, 34.17252228774368916 ) ) ;
#19751=CARTESIAN_POINT ( 'NONE',  ( 5.779280353836490358E-15, 55.00000000546238965, 32.49999999999999289 ) ) ;
#19755=CARTESIAN_POINT ( 'NONE',  ( -27.16883889988624290, 38.92500000273117422, -19.73931689729374028 ) ) ;
#19756=CARTESIAN_POINT ( 'NONE',  ( 20.75514604977249178, 6.075000002731190563, 28.56700777964553950 ) ) ;
#19757=CARTESIAN_POINT ( 'NONE',  ( -33.58253175000000113, 53.47500000273117848, 10.91162601494193929 ) ) ;
#19761=CARTESIAN_POINT ( 'NONE',  ( 6.277390505771533514E-15, 65.00000000546236834, 34.17252228774368916 ) ) ;
#19764=CARTESIAN_POINT ( 'NONE',  ( -26.29305231718579350, 53.79999999999999716, -19.10302069950537884 ) ) ;
#19767=CARTESIAN_POINT ( 'NONE',  ( 33.58253175000000113, 40.47500000273118559, -10.91162601494193751 ) ) ;
#19769=CARTESIAN_POINT ( 'NONE',  ( -32.50000000000000000, 28.60000000546238397, 10.55989012756946366 ) ) ;
#19782=DIRECTION ( 'NONE',  ( 0.000000000000000000, 1.000000000000000000, 0.000000000000000000 ) ) ;
#19786=FACE_OUTER_BOUND ( 'NONE', #8910, .T. ) ;
#19787=CARTESIAN_POINT ( 'NONE',  ( 10.37757302488624056, 78.77500000273117564, -31.93888565452638417 ) ) ;
#19793=CARTESIAN_POINT ( 'NONE',  ( 6.486482029760649416E-15, 67.62500000273119838, 35.31076352940723240 ) ) ;
#19794=CARTESIAN_POINT ( 'NONE',  ( -27.16883889988624290, 25.17500000273119198, -19.73931689729374028 ) ) ;
#19795=CARTESIAN_POINT ( 'NONE',  ( 10.37757302488624056, 14.77500000273117209, -31.93888565452638417 ) ) ;
#19800=CARTESIAN_POINT ( 'NONE',  ( -10.04305231718578462, 48.39999999999998437, 30.90933677959249337 ) ) ;
#19807=CARTESIAN_POINT ( 'NONE',  ( -20.75514604977248112, 59.67500000273118133, 28.56700777964554661 ) ) ;
#19812=CARTESIAN_POINT ( 'NONE',  ( -20.75514604977248112, 33.42500000273120264, 28.56700777964554661 ) ) ;
#19833=CARTESIAN_POINT ( 'NONE',  ( -33.58253175000000113, 43.27500000273117564, -10.91162601494193218 ) ) ;
#19838=CARTESIAN_POINT ( 'NONE',  ( 10.04305231718579705, 64.60000000000000853, 30.90933677959248982 ) ) ;
#19849=CARTESIAN_POINT ( 'NONE',  ( 33.58253175000000113, 50.22500000273118559, -10.91162601494193751 ) ) ;
#19850=CARTESIAN_POINT ( 'NONE',  ( -20.75514604977248823, 23.07500000273117635, -28.56700777964554305 ) ) ;
#19866=CARTESIAN_POINT ( 'NONE',  ( 20.75514604977249178, 55.82500000273118701, 28.56700777964553950 ) ) ;
#19882=CARTESIAN_POINT ( 'NONE',  ( -10.37757302488624411, 20.72500000273118204, -31.93888565452638417 ) ) ;
#19887=CARTESIAN_POINT ( 'NONE',  ( -10.04305231718579172, 42.10000000546236265, -30.90933677959248982 ) ) ;
#19895=CARTESIAN_POINT ( 'NONE',  ( -10.37757302488624411, 70.72500000273117848, -31.93888565452638417 ) ) ;
#19902=CARTESIAN_POINT ( 'NONE',  ( -26.29305231718579350, 8.300000005462369046, -19.10302069950537884 ) ) ;
#19911=( NAMED_UNIT ( * ) SI_UNIT ( $, .STERADIAN. ) SOLID_ANGLE_UNIT ( ) );
#19912=CARTESIAN_POINT ( 'NONE',  ( -32.50000000000000000, 38.09999999999999432, 10.55989012756946366 ) ) ;
#19927=CARTESIAN_POINT ( 'NONE',  ( 10.37757302488624056, 38.52500000273119696, -31.93888565452638417 ) ) ;
#19928=CARTESIAN_POINT ( 'NONE',  ( 10.37757302488624056, 2.775000002731189852, -31.93888565452638417 ) ) ;
#19929=CARTESIAN_POINT ( 'NONE',  ( -33.58253175000000113, 53.27500000273118275, -10.91162601494193041 ) ) ;
#19932=CARTESIAN_POINT ( 'NONE',  ( 32.50000000000000000, 61.60000000546236976, -10.55989012756945833 ) ) ;
#19938=CARTESIAN_POINT ( 'NONE',  ( -33.58253175000000113, 39.27500000273118275, -10.91162601494193218 ) ) ;
#19942=CARTESIAN_POINT ( 'NONE',  ( 20.08610463437157279, 27.80000000546238326, -27.64615127144129758 ) ) ;
#19943=ORIENTED_EDGE ( 'NONE', *, *, #9844, .T. ) ;
#19953=CARTESIAN_POINT ( 'NONE',  ( -29.51723652120143981, 66.96161537668497488, -16.50702486923799128 ) ) ;
#19956=EDGE_CURVE ( 'NONE', #2905, #15118, #32787, .T. ) ;
#19965=CARTESIAN_POINT ( 'NONE',  ( -2.162160676586881955E-15, 78.87500000273118417, -35.31076352940723240 ) ) ;
#19970=CARTESIAN_POINT ( 'NONE',  ( -20.75514604977248823, 62.82500000273119412, -28.56700777964554305 ) ) ;
#19971=CARTESIAN_POINT ( 'NONE',  ( 6.486482029760649416E-15, 25.87500000273117351, 35.31076352940723240 ) ) ;
#19972=CARTESIAN_POINT ( 'NONE',  ( 33.58253175000000113, 8.375000002731184168, -4.112674001490185761E-15 ) ) ;
#19976=CARTESIAN_POINT ( 'NONE',  ( 10.37757302488624767, 7.725000002731172266, 31.93888565452638417 ) ) ;
#19978=CARTESIAN_POINT ( 'NONE',  ( 10.04305231718579705, 44.60000000000001563, 30.90933677959248982 ) ) ;
#19983=CARTESIAN_POINT ( 'NONE',  ( -33.58253175000000113, 61.47500000273117848, 10.91162601494193929 ) ) ;
#19988=CARTESIAN_POINT ( 'NONE',  ( 33.58253175000000113, 32.12500000273120548, -4.112674001490185761E-15 ) ) ;
#19991=ORIENTED_EDGE ( 'NONE', *, *, #21409, .T. ) ;
#20010=CARTESIAN_POINT ( 'NONE',  ( 27.16883889988623935, 76.32500000273120122, -19.73931689729374384 ) ) ;
#20011=CARTESIAN_POINT ( 'NONE',  ( 33.58253175000000823, 40.27500000273118985, 10.91162601494192863 ) ) ;
#20017=CARTESIAN_POINT ( 'NONE',  ( 26.29305231718578995, 65.20000000000001705, -19.10302069950538240 ) ) ;
#20027=CARTESIAN_POINT ( 'NONE',  ( -33.58253175000000113, 47.12500000273119127, 0.000000000000000000 ) ) ;
#20028=CARTESIAN_POINT ( 'NONE',  ( 33.58253175000000113, 24.47500000273118914, -10.91162601494193751 ) ) ;
#20036=MECHANICAL_DESIGN_GEOMETRIC_PRESENTATION_REPRESENTATION('',(#5249),#9618);
#20051=CARTESIAN_POINT ( 'NONE',  ( 33.58253175000000113, 60.47500000273118559, -10.91162601494193751 ) ) ;
#20055=DIRECTION ( 'NONE',  ( 0.000000000000000000, 1.000000000000000000, 0.000000000000000000 ) ) ;
#20058=CARTESIAN_POINT ( 'NONE',  ( 20.08610463437157279, 63.80000000546237970, -27.64615127144129758 ) ) ;
#20059=CARTESIAN_POINT ( 'NONE',  ( -32.52223864317537050, 52.00000000000001421, 1.355835680407736499 ) ) ;
#20060=CARTESIAN_POINT ( 'NONE',  ( -10.37757302488624411, 24.72500000273118559, -31.93888565452638417 ) ) ;
#20063=EDGE_CURVE ( 'NONE', #33963, #30034, #8366, .T. ) ;
#20066=CARTESIAN_POINT ( 'NONE',  ( -20.08610463437156923, 40.80000000546237260, 27.64615127144130113 ) ) ;
#20073=CARTESIAN_POINT ( 'NONE',  ( 20.75514604977249178, 69.82500000273118701, 28.56700777964553950 ) ) ;
#20080=CARTESIAN_POINT ( 'NONE',  ( -27.16883889988623935, 13.32500000273119412, 19.73931689729374739 ) ) ;
#20087=DIRECTION ( 'NONE',  ( 0.000000000000000000, 0.000000000000000000, 1.000000000000000000 ) ) ;
#20089=CARTESIAN_POINT ( 'NONE',  ( 26.29305231718578995, 33.19999999999999574, -19.10302069950538240 ) ) ;
#20097=ORIENTED_EDGE ( 'NONE', *, *, #29070, .T. ) ;
#20102=CARTESIAN_POINT ( 'NONE',  ( -33.58253175000000113, 43.22500000273118559, 10.91162601494193929 ) ) ;
#20103=CARTESIAN_POINT ( 'NONE',  ( -27.16883889988623935, 5.575000002731187010, 19.73931689729374739 ) ) ;
#20104=CARTESIAN_POINT ( 'NONE',  ( 33.58253175000000113, 58.47500000273119269, -10.91162601494193574 ) ) ;
#20108=CARTESIAN_POINT ( 'NONE',  ( 32.50000000000000000, 61.50000000546239676, -3.980102097228898626E-15 ) ) ;
#20116=CARTESIAN_POINT ( 'NONE',  ( 20.75514604977248467, 38.67500000273117422, -28.56700777964554305 ) ) ;
#20118=ORIENTED_EDGE ( 'NONE', *, *, #30881, .F. ) ;
#20120=CARTESIAN_POINT ( 'NONE',  ( 32.50000000000000000, 31.50000000546236834, -3.980102097228898626E-15 ) ) ;
#20124=ORIENTED_EDGE ( 'NONE', *, *, #18935, .T. ) ;
#20137=DIRECTION ( 'NONE',  ( 0.000000000000000000, 0.000000000000000000, 1.000000000000000000 ) ) ;
#20140=CARTESIAN_POINT ( 'NONE',  ( 6.277390505771533514E-15, 4.500000000000003553, 34.17252228774368916 ) ) ;
#20141=ORIENTED_EDGE ( 'NONE', *, *, #31700, .F. ) ;
#20145=CARTESIAN_POINT ( 'NONE',  ( -27.16883889988624290, 62.92500000273119554, -19.73931689729374028 ) ) ;
#20146=CARTESIAN_POINT ( 'NONE',  ( -20.75514604977248112, 23.67500000273118843, 28.56700777964554661 ) ) ;
#20147=CARTESIAN_POINT ( 'NONE',  ( 33.58253175000000113, 12.37500000273118772, -4.112674001490185761E-15 ) ) ;
#20151=CARTESIAN_POINT ( 'NONE',  ( 26.29305231718579350, 77.30000000546237970, 19.10302069950537529 ) ) ;
#20153=CARTESIAN_POINT ( 'NONE',  ( -20.08610463437157989, 43.69999999999998863, -27.64615127144129758 ) ) ;
#20159=CARTESIAN_POINT ( 'NONE',  ( -33.58253175000000113, 61.37500000273120548, 0.000000000000000000 ) ) ;
#20164=ORIENTED_EDGE ( 'NONE', *, *, #31033, .F. ) ;
#20165=CARTESIAN_POINT ( 'NONE',  ( -33.58253175000000113, 33.22500000273117138, 10.91162601494193929 ) ) ;
#20184=CARTESIAN_POINT ( 'NONE',  ( -33.58253175000000113, 45.47500000273119980, 10.91162601494193929 ) ) ;
#20191=CARTESIAN_POINT ( 'NONE',  ( -2.092463501923844636E-15, 57.49999999999999289, -34.17252228774368916 ) ) ;
#20196=CARTESIAN_POINT ( 'NONE',  ( -33.58253175000000113, 79.27500000273118985, -10.91162601494193218 ) ) ;
#20201=CARTESIAN_POINT ( 'NONE',  ( -20.75514604977248823, 52.82500000273116569, -28.56700777964554305 ) ) ;
#20202=CARTESIAN_POINT ( 'NONE',  ( -33.58253175000000113, 23.47500000273119269, 10.91162601494193929 ) ) ;
#20228=CARTESIAN_POINT ( 'NONE',  ( -2.162160676586881955E-15, 62.87500000273120548, -35.31076352940723240 ) ) ;
#20236=CARTESIAN_POINT ( 'NONE',  ( 33.58253175000000823, 22.02500000273117919, 10.91162601494192863 ) ) ;
#20241=CARTESIAN_POINT ( 'NONE',  ( 10.04305231718578817, 39.90000000546238823, -30.90933677959249337 ) ) ;
#20246=CARTESIAN_POINT ( 'NONE',  ( 33.58253175000000113, 70.22500000273120691, -10.91162601494193751 ) ) ;
#20252=CARTESIAN_POINT ( 'NONE',  ( 27.16883889988623935, 12.32500000273119234, -19.73931689729374384 ) ) ;
#20261=CARTESIAN_POINT ( 'NONE',  ( 32.50000000000000711, 26.89999999999999147, 10.55989012756945122 ) ) ;
#20273=CARTESIAN_POINT ( 'NONE',  ( 10.37757302488624767, 39.72500000273119980, 31.93888565452638417 ) ) ;
#20274=CARTESIAN_POINT ( 'NONE',  ( 20.75514604977248467, 4.675000002731191096, -28.56700777964554305 ) ) ;
#20275=CARTESIAN_POINT ( 'NONE',  ( -2.162160676586882350E-15, 54.87500000273119838, -35.31076352940722529 ) ) ;
#20279=CARTESIAN_POINT ( 'NONE',  ( 10.04305231718578817, 61.90000000546237402, -30.90933677959249337 ) ) ;
#20284=CARTESIAN_POINT ( 'NONE',  ( -1.137977401836464321E-14, 52.00000000000000711, 46.18802153517007270 ) ) ;
#20286=CARTESIAN_POINT ( 'NONE',  ( 33.58253175000000823, 36.27500000273119696, 10.91162601494192863 ) ) ;
#20290=CARTESIAN_POINT ( 'NONE',  ( -26.29305231718578995, 20.70000000546238894, 19.10302069950538595 ) ) ;
#20308=CARTESIAN_POINT ( 'NONE',  ( 10.04305231718578817, 5.400000000000002132, -30.90933677959249337 ) ) ;
#20314=CARTESIAN_POINT ( 'NONE',  ( 33.58253175000000823, 60.02500000273116854, 10.91162601494192863 ) ) ;
#20315=CARTESIAN_POINT ( 'NONE',  ( 27.16883889988624290, 26.17500000273119554, 19.73931689729373673 ) ) ;
#20316=CARTESIAN_POINT ( 'NONE',  ( 20.75514604977249178, 10.07500000273119234, 28.56700777964553950 ) ) ;
#20321=CARTESIAN_POINT ( 'NONE',  ( -2.092463501923844636E-15, 78.00000000546238255, -34.17252228774368916 ) ) ;
#20323=CARTESIAN_POINT ( 'NONE',  ( -26.29305231718579350, 39.79999999999999005, -19.10302069950537884 ) ) ;
#20328=CARTESIAN_POINT ( 'NONE',  ( 10.37757302488624767, 53.97500000273118559, 31.93888565452638417 ) ) ;
#20333=CARTESIAN_POINT ( 'NONE',  ( -33.58253175000000113, 29.22500000273118914, 10.91162601494193929 ) ) ;
#20356=CARTESIAN_POINT ( 'NONE',  ( -20.75514604977248112, 45.67500000273119554, 28.56700777964554661 ) ) ;
#20361=CARTESIAN_POINT ( 'NONE',  ( -10.04305231718578462, 62.39999999999999858, 30.90933677959249337 ) ) ;
#20366=CARTESIAN_POINT ( 'NONE',  ( -10.37757302488623701, 77.77500000273117564, 31.93888565452638417 ) ) ;
#20371=CARTESIAN_POINT ( 'NONE',  ( 33.58253175000000823, 48.02500000273119696, 10.91162601494192863 ) ) ;
#20372=CARTESIAN_POINT ( 'NONE',  ( 27.16883889988623935, 20.57500000273120122, -19.73931689729374384 ) ) ;
#20376=CARTESIAN_POINT ( 'NONE',  ( -1.778240108872766143E-15, 62.00000000546238255, -32.49999999999999289 ) ) ;
#20396=CARTESIAN_POINT ( 'NONE',  ( 20.75514604977248467, 62.67500000273117422, -28.56700777964554305 ) ) ;
#20402=CARTESIAN_POINT ( 'NONE',  ( 27.16883889988624290, 19.92500000273118843, 19.73931689729373673 ) ) ;
#20404=CARTESIAN_POINT ( 'NONE',  ( 26.29305231718579350, 52.79999999999999716, 19.10302069950537529 ) ) ;
#20405=LINE ( 'NONE', #7177, #11111 ) ;
#20407=CARTESIAN_POINT ( 'NONE',  ( 32.50000000000000711, 43.40000000546238113, 10.55989012756945122 ) ) ;
#20413=CARTESIAN_POINT ( 'NONE',  ( -20.75514604977248112, 69.42500000273116711, 28.56700777964554661 ) ) ;
#20421=CARTESIAN_POINT ( 'NONE',  ( 20.75514604977249178, 9.825000002731188786, 28.56700777964553950 ) ) ;
#20431=CARTESIAN_POINT ( 'NONE',  ( 20.08610463437158344, 28.69999999999999574, 27.64615127144129403 ) ) ;
#20435=CARTESIAN_POINT ( 'NONE',  ( -1.353501352685664516, 67.00000000000001421, 32.52334280248232545 ) ) ;
#20445=CARTESIAN_POINT ( 'NONE',  ( 10.37757302488624056, 40.52500000273119696, -31.93888565452638417 ) ) ;
#20446=CARTESIAN_POINT ( 'NONE',  ( 0.000000000000000000, 52.00000000000000711, 0.000000000000000000 ) ) ;
#20447=CARTESIAN_POINT ( 'NONE',  ( 27.16883889988624290, 56.17500000273119554, 19.73931689729373673 ) ) ;
#20451=CARTESIAN_POINT ( 'NONE',  ( 32.50000000000000711, 63.40000000546236691, 10.55989012756945122 ) ) ;
#20458=CARTESIAN_POINT ( 'NONE',  ( 27.16883889988623935, 34.57500000273118701, -19.73931689729374384 ) ) ;
#20462=CARTESIAN_POINT ( 'NONE',  ( 20.08610463437157279, 21.80000000546236549, -27.64615127144129758 ) ) ;
#20466=ORIENTED_EDGE ( 'NONE', *, *, #32022, .T. ) ;
#20473=CARTESIAN_POINT ( 'NONE',  ( -27.16883889988623935, 63.32500000273120833, 19.73931689729374739 ) ) ;
#20483=CARTESIAN_POINT ( 'NONE',  ( 27.16883889988623935, 76.57500000273120122, -19.73931689729374384 ) ) ;
#20488=CARTESIAN_POINT ( 'NONE',  ( 27.16883889988624290, 59.92500000273119554, 19.73931689729373673 ) ) ;
#20489=CARTESIAN_POINT ( 'NONE',  ( 20.75514604977248467, 20.67500000273119909, -28.56700777964554305 ) ) ;
#20490=CARTESIAN_POINT ( 'NONE',  ( 33.58253175000000823, 8.275000002731191628, 10.91162601494192863 ) ) ;
#20496=CARTESIAN_POINT ( 'NONE',  ( -33.58253175000000113, 3.225000002731179372, 10.91162601494193929 ) ) ;
#20498=CARTESIAN_POINT ( 'NONE',  ( 32.50000000000000000, 43.00000000000000000, -3.980102097228898626E-15 ) ) ;
#20504=CARTESIAN_POINT ( 'NONE',  ( 5.779280353836490358E-15, 61.00000000546238255, 32.49999999999999289 ) ) ;
#20506=CARTESIAN_POINT ( 'NONE',  ( -10.37757302488623701, 51.77500000273120406, 31.93888565452638417 ) ) ;
#20510=ORIENTED_EDGE ( 'NONE', *, *, #4410, .F. ) ;
#20511=CARTESIAN_POINT ( 'NONE',  ( 33.58253175000000113, 24.12500000273119838, -4.112674001490185761E-15 ) ) ;
#20513=ORIENTED_EDGE ( 'NONE', *, *, #16923, .T. ) ;
#20515=B_SPLINE_CURVE_WITH_KNOTS ( 'NONE', 3,
 ( #1656, #30144, #3909, #25530, #6648, #2007, #12483, #25008, #22952, #9907 ),
 .UNSPECIFIED., .F., .F.,
 ( 4, 2, 2, 2, 4 ),
 ( 0.000000000000000000, 0.006590582801587962884, 0.01318116560317592577, 0.01977174840476388779, 0.02636233120635185154 ),
 .UNSPECIFIED. ) ;
#20528=CARTESIAN_POINT ( 'NONE',  ( 5.147494310547434893, 54.55125428154683220, 32.49999999999999289 ) ) ;
#20529=CARTESIAN_POINT ( 'NONE',  ( 26.29305231718579350, 14.79999999999999361, 19.10302069950537529 ) ) ;
#20534=CARTESIAN_POINT ( 'NONE',  ( -33.58253175000000113, 77.22500000273117848, 10.91162601494193929 ) ) ;
#20535=CARTESIAN_POINT ( 'NONE',  ( -27.16883889988623935, 41.57500000273119412, 19.73931689729374739 ) ) ;
#20540=CARTESIAN_POINT ( 'NONE',  ( -2.092463501923844636E-15, 59.50000000000001421, -34.17252228774368916 ) ) ;
#20544=CARTESIAN_POINT ( 'NONE',  ( 27.16883889988624290, 76.17500000273118133, 19.73931689729373673 ) ) ;
#20549=CARTESIAN_POINT ( 'NONE',  ( 20.75514604977249178, 41.82500000273119412, 28.56700777964553950 ) ) ;
#20551=ORIENTED_EDGE ( 'NONE', *, *, #23429, .T. ) ;
#20554=CARTESIAN_POINT ( 'NONE',  ( 6.277390505771533514E-15, 3.000000005462379882, 34.17252228774368916 ) ) ;
#20558=PRODUCT_DEFINITION_SHAPE ( 'NONE', 'NONE',  #7646 ) ;
#20575=CARTESIAN_POINT ( 'NONE',  ( 33.58253175000000113, 62.47500000273118559, -10.91162601494193751 ) ) ;
#20581=CARTESIAN_POINT ( 'NONE',  ( 32.50000000000000711, 76.89999999999999147, 10.55989012756945122 ) ) ;
#20582=CARTESIAN_POINT ( 'NONE',  ( -10.37757302488624411, 14.72500000273117848, -31.93888565452638417 ) ) ;
#20587=CARTESIAN_POINT ( 'NONE',  ( -26.29305231718579350, 40.30000000546237260, -19.10302069950537884 ) ) ;
#20593=CARTESIAN_POINT ( 'NONE',  ( 6.486482029760649416E-15, 69.62500000273118417, 35.31076352940723240 ) ) ;
#20600=CARTESIAN_POINT ( 'NONE',  ( -10.37757302488624411, 8.725000002731173154, -31.93888565452638417 ) ) ;
#20610=CARTESIAN_POINT ( 'NONE',  ( 5.485887633599118468E-07, 52.00000000000003553, -32.49999999999999289 ) ) ;
#20613=CARTESIAN_POINT ( 'NONE',  ( -32.50000000000000000, 29.89999999999998437, -10.55989012756945478 ) ) ;
#20626=CARTESIAN_POINT ( 'NONE',  ( -27.16883889988624290, 34.92500000273117422, -19.73931689729374028 ) ) ;
#20630=CARTESIAN_POINT ( 'NONE',  ( -20.08610463437157989, 60.20000000546237828, -27.64615127144129758 ) ) ;
#20638=CARTESIAN_POINT ( 'NONE',  ( 27.16883889988624290, 36.17500000273120264, 19.73931689729373673 ) ) ;
#20642=CARTESIAN_POINT ( 'NONE',  ( 32.50000000000000000, 25.60000000546239107, -10.55989012756945833 ) ) ;
#20655=CARTESIAN_POINT ( 'NONE',  ( 20.75514604977248467, 64.42500000273116711, -28.56700777964554305 ) ) ;
#20665=CARTESIAN_POINT ( 'NONE',  ( -10.37757302488623701, 71.77500000273118985, 31.93888565452638417 ) ) ;
#20672=CARTESIAN_POINT ( 'NONE',  ( -20.75514604977248112, 61.42500000273118133, 28.56700777964554661 ) ) ;
#20673=CARTESIAN_POINT ( 'NONE',  ( -33.58253175000000113, 15.47500000273118381, 10.91162601494193929 ) ) ;
#20674=CARTESIAN_POINT ( 'NONE',  ( 6.486482029760649416E-15, 1.875000002731192383, 35.31076352940723240 ) ) ;
#20678=CARTESIAN_POINT ( 'NONE',  ( 10.37757302488624056, 4.525000002731191628, -31.93888565452638417 ) ) ;
#20679=CARTESIAN_POINT ( 'NONE',  ( 32.87414713444668024, 52.00000000000002132, 6.322578566052129645 ) ) ;
#20680=CARTESIAN_POINT ( 'NONE',  ( 10.04305231718578817, 39.40000000000000568, -30.90933677959249337 ) ) ;
#20685=CARTESIAN_POINT ( 'NONE',  ( -10.37757302488624411, 50.97500000273118559, -31.93888565452638417 ) ) ;
#20686=CARTESIAN_POINT ( 'NONE',  ( 20.08610463437158344, 59.20000000546237828, 27.64615127144129403 ) ) ;
#20690=CARTESIAN_POINT ( 'NONE',  ( 33.58253175000000823, 24.02500000273117564, 10.91162601494192863 ) ) ;
#20692=EDGE_LOOP ( 'NONE', ( #1399, #28194, #6438, #14622 ) ) ;
#20693=CARTESIAN_POINT ( 'NONE',  ( -5.147494310547322094, 57.55125428154683931, -32.50000000000003553 ) ) ;
#20705=CARTESIAN_POINT ( 'NONE',  ( -20.08610463437157989, 15.69999999999999929, -27.64615127144129758 ) ) ;
#20711=CARTESIAN_POINT ( 'NONE',  ( -27.16883889988623935, 39.57500000273118701, 19.73931689729374739 ) ) ;
#20717=CARTESIAN_POINT ( 'NONE',  ( 6.277390505771533514E-15, 58.49999999999997868, 34.17252228774368916 ) ) ;
#20721=CARTESIAN_POINT ( 'NONE',  ( 20.75514604977248467, 70.67500000273118133, -28.56700777964554305 ) ) ;
#20727=CARTESIAN_POINT ( 'NONE',  ( 33.58253175000000113, 44.12500000273119127, -4.112674001490185761E-15 ) ) ;
#20731=CARTESIAN_POINT ( 'NONE',  ( 26.29305231718578995, 5.700000005462377395, -19.10302069950538240 ) ) ;
#20750=CARTESIAN_POINT ( 'NONE',  ( 10.37757302488624056, 62.77500000273118985, -31.93888565452638417 ) ) ;
#20756=CARTESIAN_POINT ( 'NONE',  ( -33.58253175000000113, 17.02500000273118985, -10.91162601494193218 ) ) ;
#20761=CARTESIAN_POINT ( 'NONE',  ( 32.50000000000000000, 37.60000000546235555, -10.55989012756945833 ) ) ;
#20766=CARTESIAN_POINT ( 'NONE',  ( -33.58253175000000113, 65.02500000273118985, -10.91162601494193218 ) ) ;
#20771=CARTESIAN_POINT ( 'NONE',  ( 20.75514604977248467, 6.425000002731192872, -28.56700777964554305 ) ) ;
#20781=CARTESIAN_POINT ( 'NONE',  ( -20.08610463437156923, 32.29999999999999716, 27.64615127144130113 ) ) ;
#20791=EDGE_CURVE ( 'NONE', #5766, #29627, #18013, .T. ) ;
#20793=CARTESIAN_POINT ( 'NONE',  ( -20.75514604977248823, 36.82500000273117990, -28.56700777964554305 ) ) ;
#20798=CARTESIAN_POINT ( 'NONE',  ( -10.04305231718579172, 52.10000000546237686, -30.90933677959248982 ) ) ;
#20805=CARTESIAN_POINT ( 'NONE',  ( 33.58253175000000113, 36.47500000273119269, -10.91162601494193751 ) ) ;
#20809=CARTESIAN_POINT ( 'NONE',  ( 20.08610463437158344, 21.20000000546238894, 27.64615127144129403 ) ) ;
#20814=DIRECTION ( 'NONE',  ( 0.000000000000000000, 1.000000000000000000, 0.000000000000000000 ) ) ;
#20819=CARTESIAN_POINT ( 'NONE',  ( 10.37757302488624056, 62.52500000273118985, -31.93888565452638417 ) ) ;
#20823=( BOUNDED_SURFACE ( )  B_SPLINE_SURFACE ( 1, 2, ( 
 ( #12844, #23318, #30853, #23487, #28791, #4773, #25547, #33948, #7344, #15251, #18175, #2193, #12668, #23136, #26228, #15601, #2549, #31366, #2027, #18347, #28115, #33783, #13180, #12501, #31199, #23658, #7690, #33428, #9925, #33603, #10101, #20581, #31026, #7523, #18007, #5117, #29459, #3391, #295, #5962, #14023, #23995, #13695, #13861, #3060, #24326, #18517, #630, #24487, #16113, #26396, #31537, #466, #16605, #19180, #5459, #10782, #800, #26565, #8031, #13532, #10949, #21259, #28963, #11282, #29126, #16276, #13355, #29618, #5629, #31704, #8360, #26734, #3227, #21425, #8196, #11120, #31866, #19018, #21760, #2889, #8531, #24160, #18848, #29296, #21588, #8697, #23830, #15940, #21091, #5794, #32203, #6121, #32034, #27058, #3551, #16440, #18687, #26892, #10611, #30122, #17271, #32367, #1467, #14357, #6464, #9191, #1630, #11943, #25154, #960, #1120, #6792, #22412, #14524, #16938, #6625, #12108, #17104, #27563, #11605, #4222, #9535, #32531, #6292, #14696, #22087, #9031, #32860, #19511, #29959, #27395, #30463, #30291, #27733, #22580, #19346, #33031, #8861, #4049, #6961, #3884, #9357, #1292, #11440, #29788, #24983, #16768, #20017, #21917, #24815, #11774, #17446, #27227, #19838, #4389, #22254, #3721, #14191, #32697, #27907, #14863, #24646, #19676, #28580, #7302, #12282, #28246, #17786, #15040, #22756, #18136, #9882, #30985, #28073, #10400, #20361, #25505, #23097, #7485, #17965, #30807, #12459, #15385, #12628, #33741, #5076, #17611, #23276, #28414, #4729, #15210, #25841, #23449, #4562, #33206, #1806, #33560, #15562, #26014, #2328, #20879, #2507, #4904, #7131, #20540, #22929, #12804, #7650, #9709, #10236, #25673, #2154, #10060, #12974, #20717, #33910, #25327, #1984, #31158, #31328, #7819, #18308, #28753, #5250, #20191, #30634, #33385, #18977, #24290, #13314, #21049, #29422, #2844, #23787, #13657, #254, #10739, #21217, #11242, #11079, #31994, #5924, #83, #16401, #13141, #21382, #21719, #8157, #24122, #16069, #26186, #10570, #5756, #31498, #21548, #2682, #31661, #29579, #16237, #8490, #23954, #761, #26855, #7990, #15899, #32164, #18475, #3351, #26525, #13821, #588, #8657, #5419, #19142, #15732, #29084, #18809, #23614, #29253, #28919, #18646, #26354, #5588, #26691, #3017, #13489, #424, #10910, #31827, #8320, #3187, #923, #29747, #9315, #22046, #27018, #8992, #32492, #6253, #3514, #32824, #24610, #11732, #8820, #25117, #1084, #16732, #3844, #22213, #32660, #11564, #27188, #30081, #27359, #14486, #19800, #32329, #4011, #9155, #19472, #29922, #6587, #4184, #19305, #13985, #16564, #14318, #30250, #6753, #17063, #1592, #17233, #19638, #21879, #1252, #3680, #27524, #22376, #24447, #24942, #6425, #16897, #24774, #27693, #1426, #14657, #6081, #14153, #11904, #12070, #22540, #32989, #9496, #19978, #11402, #28208, #9673, #17928, #12766, #7093, #25291, #28379, #20153, #30598, #33521, #17577, #28036, #4523, #33699, #20498, #7444, #4868, #4351, #15348, #17406, #17748, #10200, #14998, #10025, #22891, #6923, #14827, #25639, #1763, #30947, #30424, #25468, #27869, #25802, #23239, #2118, #12243, #31120, #1945, #12421, #22721, #33348, #7613, #12591, #33169, #9846, #20323, #2293, #30772, #7263, #20680, #4694, #15174, #23062, #17341, #21983, #27294, #22651, #29859, #27804, #3951, #4288, #12009, #19912, #16838, #22479, #30534, #6531, #30189, #30361, #19578, #6862, #1021, #17175, #7030, #32597, #8929, #14093, #17004, #33103, #1702, #32431, #3786, #14763, #9097, #24549, #30026, #27461, #14256, #11503, #25227, #11672, #32765, #6359, #12181, #22155, #24714, #24881, #9259, #19743, #14426, #1191, #27633, #1364, #1534, #9608, #19410, #25053, #6691, #11841, #22320, #4121, #20089, #14596, #32928, #3619, #9427, #27125, #7718, #18034, #2579, #20781, #31057, #33284, #12699, #15110, #23170, #33810, #14935, #28480, #30880, #22999, #25740, #18205, #4976, #28648, #17513, #17684, #23348, #15454, #7550, #33456, #33632, #5144, #10131, #20613, #28145, #31225, #26083, #25574, #22824, #15631, #4631, #2054, #25909, #12530, #9955, #20431, #13043, #12871, #10303, #23514, #1878, #33974, #25400, #2403, #10467, #7377, #20946, #17861, #27974, #12355, #31395, #9781, #4458, #20261, #28312, #30706, #7201, #4800, #15280, #2222, #13558, #8559, #8218, #18712, #24020, #24183, #16300, #18871, #824, #26590, #19043, #490, #29148, #656, #5654, #24353, #31727, #3249, #28987, #8056, #5486, #10973, #16136, #3086, #21447, #18374, #31890, #26253, #31558, #11305, #8386, #11144, #21287, #21783, #29320, #5822, #21614, #26757, #13887, #13719, #32059, #26916, #29481, #5985, #16462, #7885, #28819, #3413, #5317, #15797, #2741, #13205, #10807, #15965, #2915, #23681, #21115, #147, #10636, #18541, #26421, #13382, #23854, #320, #21203, #23435, #12961, #31146, #23772, #29071, #18119, #25828, #240, #7637, #28566, #18461, #5062, #15547, #25999, #16056, #15885, #2830, #10726, #4892, #31647, #17954, #26174, #26511, #33896, #28905, #20865, #30972, #15373, #10554, #2318, #26341, #7472, #2492, #411, #21035, #13299, #28739, #5575, #8145, #12791, #20705, #3004, #23265, #18634, #31311, #13477, #5406, #23942, #10225, #20529, #28403, #10387, #23601, #33727, #7805, #18294, #5235, #31485, #15719, #2668, #13127, #68, #7975, #31980, #909, #32149, #19289, #24596, #3175, #8806, #3499, #24274, #742, #11388, #8977, #13644, #31814, #21370, #8642, #14140, #1070, #21865, #29907, #11550, #24432, #26679, #6065, #8477, #16548, #27173, #8305, #32315, #11227, #16387, #19127, #22032, #29732, #32476, #10897, #11066, #16718, #6237, #3666, #26840, #5910, #19459, #13806, #3335, #21532, #6410, #16882, #18964, #16225, #27345, #29408, #21703, #3831, #29564, #27001, #13969, #14305, #24761, #18796, #29240, #5744, #24108, #576, #6911, #7248, #27681, #33156, #1580, #11717, #19624, #25277, #30069, #7080, #22200, #32810, #15160, #1750, #28021, #9482, #20308, #25453, #6575, #1414, #30758, #3999, #1929, #12057, #12407, #20140, #4509, #24929, #30584, #4681, #14645, #4338, #14983, #4171, #22877, #9141, #12230, #1239, #6741, #17049, #32647, #25104, #17735, #9831, #27511, #11892, #33334, #17222, #14472, #22527, #32978 ),
 ( #28193, #17564, #14812, #22363, #9303, #19965, #19787, #30236, #22704, #30411, #17392, #27856, #9659, #23565, #28366, #33858, #5198, #7600, #28869, #31608, #10684, #4854, #2629, #15508, #7768, #2454, #18255, #12920, #20483, #10012, #28701, #23048, #25960, #29, #15846, #10519, #21166, #13091, #15334, #31445, #7937, #18425, #15682, #23396, #25789, #5366, #13258, #5536, #26131, #31106, #31275, #18080, #23734, #5023, #20996, #12578, #10352, #20830, #26303, #33507, #2792, #198, #25626, #28528, #8106, #30934, #2105, #10183, #7427, #18593, #29033, #17914, #2278, #12753, #23225, #33684, #20665, #3133, #16017, #870, #16185, #21660, #16676, #16347, #26803, #32105, #32274, #24395, #26960, #8940, #704, #27132, #8604, #3298, #8767, #13763, #32439, #5869, #11350, #13606, #26639, #24072, #19087, #24233, #11190, #29526, #26471, #6029, #372, #5707, #19418, #16508, #19250, #29370, #29867, #18923, #3461, #10858, #2965, #537, #13433, #13931, #21828, #23901, #29690, #3627, #21333, #6196, #14101, #11024, #31774, #24557, #21494, #1031, #11511, #21991, #8266, #18758, #29202, #31942, #8434, #33777, #25541, #7516, #12494, #17648, #33596, #4596, #23312, #30668, #2187, #27941, #6997, #4424, #9919, #28109, #15073, #2019, #16846, #22963, #24723, #30496, #10268, #33421, #10096, #20228, #20750, #20396, #30847, #20575, #4766, #12838, #7338, #17823, #25873, #28280, #15244, #25706, #6368, #27302, #31019, #23130, #12661, #1667, #18001, #9742, #14899, #1841, #28446, #20051, #4937, #3793, #15419, #2365, #9574, #14266, #12142, #22791, #22615, #33068, #17479, #25363, #12321, #7166, #33244, #8025, #23822, #18511, #26049, #15595, #13349, #28611, #21083, #5623, #21417, #29120, #26726, #8190, #20909, #3054, #13525, #23988, #10776, #31532, #31360, #460, #18842, #11113, #288, #2712, #2883, #13173, #29288, #10605, #16107, #18169, #5453, #28957, #26558, #5111, #21253, #10942, #31193, #18680, #24153, #15934, #31860, #31697, #26390, #8353, #5788, #13689, #16269, #3221, #18340, #7852, #28785, #624, #7683, #2543, #13009, #23481, #33943, #10434, #5283, #15766, #26220, #23651, #113, #14518, #6286, #16762, #14351, #19506, #27556, #27221, #32524, #6619, #3714, #14184, #24640, #4044, #24977, #1286, #3878, #1114, #5955, #24808, #24480, #8691, #16597, #11599, #793, #27389, #1460, #19670, #29953, #24320, #29781, #22080, #3545, #11765, #21582, #17098, #11276, #9024, #11434, #6457, #32361, #16931, #8855, #16435, #26887, #22247, #19009, #21911, #32691, #9186, #30115, #32028, #8525, #21752, #29453, #3384, #13854, #32197, #19337, #19175, #29612, #6114, #27052, #14017, #954, #17606, #17439, #33554, #25324, #20356, #32855, #20184, #9704, #30803, #9351, #28068, #7296, #25836, #14858, #15034, #6787, #11938, #30458, #22407, #4555, #30628, #4899, #12277, #10054, #17265, #33201, #1979, #33025, #19833, #17781, #12103, #25499, #12623, #22750, #7125, #12454, #28239, #4724, #22924, #23091, #33380, #9876, #15205, #25669, #2148, #20535, #15380, #30979, #7479, #17960, #28409, #30286, #27728, #4216, #1799, #14690, #9530, #22574, #20011, #25149, #1625, #6955, #27901, #4383, #10563, #20711, #26007, #18803, #31492, #5583, #15726, #29247, #21042, #7982, #29078, #248, #8313, #18470, #13306, #21377, #28912, #5413, #15892, #5751, #16232, #16063, #18641, #26348, #31153, #26518, #5244, #23442, #31321, #2838, #15554, #8152, #2324, #418, #10733, #5070, #23781, #21210, #18301, #3012, #12798, #31822, #2500, #31655, #26181, #13484, #13134, #23949, #23608, #7644, #18130, #10905, #33734, #2676, #23271, #10231, #28574, #12968, #33903, #10394, #20873, #7812, #28746, #76, #27009, #16394, #29915, #14312, #6581, #8813, #32156, #32322, #8649, #24767, #6072, #1077, #13651, #916, #24439, #11557, #24116, #19296, #22039, #26686, #29571, #29740, #21539, #3182, #11234, #583, #6244, #11395, #19630, #3506, #1245, #31987, #13976, #16725, #13814, #11074, #32483, #26847, #27180, #19466, #21872, #11723, #16889, #8484, #3344, #22206, #29416, #27352, #3673, #3837, #8984, #6417, #24281, #32653, #30075, #16556, #14147, #9148, #19134, #18971, #5917, #24603, #749, #21710, #32817, #4005, #30417, #23054, #25632, #11898, #6747, #20315, #32984, #14478, #19971, #9488, #17227, #24935, #9837, #1587, #22712, #19794, #2111, #12063, #27687, #14819, #33162, #9665, #22534, #4177, #7086, #4344, #25460, #30764, #9309, #14990, #20146, #6916, #17398, #17570, #15166, #30242, #1420, #27518, #25284, #7254, #17741, #28028, #12584, #28201, #30590, #14651, #12236, #25111, #4515, #33340, #22370, #1935, #27862, #1756, #12413, #4687, #22883, #33513, #17056, #10018, #20489, #30940, #21001, #23403, #2460, #8111, #10357, #33864, #18086, #10691, #16022, #5029, #12759, #21172, #28534, #15515, #5371, #25966, #12926, #20835, #2970, #2797, #23739, #31614, #25795, #18598, #4860, #13097, #13440, #31280, #15852, #7773, #17921, #2284, #31450, #23231, #13264, #28372, #18260, #21338, #33691, #7943, #10190, #203, #15340, #28706, #7435, #18431, #29038, #15688, #26477, #5541, #20673, #7606, #23907, #31112, #378, #5204, #10864, #26308, #26137, #2634, #23570, #35, #10524, #28875, #1037, #24239, #24564, #5713, #21835, #1204, #3304, #13612, #18763, #11196, #3800, #6374, #26645, #21499, #11517, #13769, #29207, #710, #21667, #31947, #16191, #21997, #16354, #3467, #542, #16852, #26809, #8440, #29532, #13937, #24401, #32113, #18931, #32280, #19094, #6202, #32445, #24077, #29697, #877, #8611, #6035, #8773, #29874, #11030, #3139, #8271, #16514, #8946, #19424, #19256, #27309, #14272, #11357, #29377, #26966, #5876, #16682, #14107, #27139, #3633, #24729, #11685, #31779, #22838, #22667, #12370, #22169, #22333, #27988, #9622, #1717, #4135, #17189, #33298, #25066, #14610, #32778, #25416, #30721, #19756, #27477, #1894, #9272, #30205, #20103, #6707, #27647, #1547, #17699, #17527, #4475, #9798, #6544, #20274, #19591, #27819, #28159, #12023, #30549, #22492, #32613, #11854, #14950, #7216, #4645, #12196, #32943, #9444, #15125, #25588, #2068, #4302, #19928, #14777, #30374, #9110, #6875, #7045, #30039, #17355, #25242, #17017, #3966, #33119, #14439, #24894, #1380 ) ),
 .UNSPECIFIED., .F., .F., .T. ) 
 B_SPLINE_SURFACE_WITH_KNOTS ( ( 2, 2 ),
 ( 3, 2, 2, 2, 2, 2, 2, 2, 2, 2, 2, 2, 2, 2, 2, 2, 2, 2, 2, 2, 2, 2, 2, 2, 2, 2, 2, 2, 2, 2, 2, 2, 2, 2, 2, 2, 2, 2, 2, 2, 2, 2, 2, 2, 2, 2, 2, 2, 2, 2, 2, 2, 2, 2, 2, 2, 2, 2, 2, 2, 2, 2, 2, 2, 2, 2, 2, 2, 2, 2, 2, 2, 2, 2, 2, 2, 2, 2, 2, 2, 2, 2, 2, 2, 2, 2, 2, 2, 2, 2, 2, 2, 2, 2, 2, 2, 2, 2, 2, 2, 2, 2, 2, 2, 2, 2, 2, 2, 2, 2, 2, 2, 2, 2, 2, 2, 2, 2, 2, 2, 2, 2, 2, 2, 2, 2, 2, 2, 2, 2, 2, 2, 2, 2, 2, 2, 2, 2, 2, 2, 2, 2, 2, 2, 2, 2, 2, 2, 2, 2, 2, 2, 2, 2, 2, 2, 2, 2, 2, 2, 2, 2, 2, 2, 2, 2, 2, 2, 2, 2, 2, 2, 2, 2, 2, 2, 2, 2, 2, 2, 2, 2, 2, 2, 2, 2, 2, 2, 2, 2, 2, 2, 2, 2, 2, 2, 2, 2, 2, 2, 2, 2, 2, 2, 2, 2, 2, 2, 2, 2, 2, 2, 2, 2, 2, 2, 2, 2, 2, 2, 2, 2, 2, 2, 2, 2, 2, 2, 2, 2, 2, 2, 2, 2, 2, 2, 2, 2, 2, 2, 2, 2, 2, 2, 2, 2, 2, 2, 2, 2, 2, 2, 2, 2, 2, 2, 2, 2, 2, 2, 2, 2, 2, 2, 2, 2, 2, 2, 2, 2, 2, 2, 2, 2, 2, 2, 2, 2, 2, 2, 2, 2, 2, 2, 2, 2, 2, 2, 2, 2, 2, 2, 2, 2, 2, 2, 2, 2, 2, 2, 2, 2, 2, 2, 2, 2, 2, 2, 2, 2, 2, 2, 2, 2, 2, 2, 2, 2, 2, 2, 2, 2, 2, 2, 2, 2, 2, 2, 2, 2, 2, 2, 2, 2, 2, 2, 2, 2, 2, 2, 2, 2, 2, 2, 2, 2, 2, 2, 2, 2, 2, 2, 2, 2, 2, 2, 2, 2, 2, 2, 2, 2, 2, 2, 2, 2, 2, 2, 2, 2, 2, 2, 2, 2, 2, 2, 2, 2, 2, 2, 2, 2, 2, 2, 2, 2, 2, 2, 2, 2, 3 ),
 ( 0.000000000000000000, 1.000000000000000000 ),
 ( 0.000000000000000000, 0.002564102564102564100, 0.005128205128205128201, 0.007692307692307692735, 0.01025641025641025640, 0.01282051282051282007, 0.01538461538461538547, 0.01794871794871794740, 0.02051282051282051280, 0.02307692307692307820, 0.02564102564102564014, 0.02820512820512820554, 0.03076923076923077094, 0.03333333333333333287, 0.03589743589743589480, 0.03846153846153846367, 0.04102564102564102561, 0.04358974358974358754, 0.04615384615384615641, 0.04871794871794871834, 0.05128205128205128027, 0.05384615384615384914, 0.05641025641025641107, 0.05897435897435897301, 0.06153846153846154188, 0.06410256410256409687, 0.06666666666666666574, 0.06923076923076923461, 0.07179487179487178961, 0.07435897435897435848, 0.07692307692307692735, 0.07948717948717948234, 0.08205128205128205121, 0.08461538461538462008, 0.08717948717948717507, 0.08974358974358974395, 0.09230769230769231282, 0.09487179487179486781, 0.09743589743589743668, 0.1000000000000000056, 0.1025641025641025605, 0.1051282051282051294, 0.1076923076923076983, 0.1102564102564102533, 0.1128205128205128221, 0.1153846153846153910, 0.1179487179487179460, 0.1205128205128205149, 0.1230769230769230838, 0.1256410256410256387, 0.1282051282051281937, 0.1307692307692307765, 0.1333333333333333315, 0.1358974358974358865, 0.1384615384615384692, 0.1410256410256410242, 0.1435897435897435792, 0.1461538461538461620, 0.1487179487179487170, 0.1512820512820512719, 0.1538461538461538547, 0.1564102564102564097, 0.1589743589743589647, 0.1615384615384615474, 0.1641025641025641024, 0.1666666666666666574, 0.1692307692307692402, 0.1717948717948717952, 0.1743589743589743501, 0.1769230769230769329, 0.1794871794871794879, 0.1820512820512820429, 0.1846153846153846256, 0.1871794871794871806, 0.1897435897435897356, 0.1923076923076923184, 0.1948717948717948734, 0.1974358974358974284, 0.2000000000000000111, 0.2025641025641025661, 0.2051282051282051211, 0.2076923076923077038, 0.2102564102564102588, 0.2128205128205128138, 0.2153846153846153966, 0.2179487179487179516, 0.2205128205128205066, 0.2230769230769230893, 0.2256410256410256443, 0.2282051282051281993, 0.2307692307692307820, 0.2333333333333333370, 0.2358974358974358920, 0.2384615384615384748, 0.2410256410256410298, 0.2435897435897435848, 0.2461538461538461675, 0.2487179487179487225, 0.2512820512820512775, 0.2538461538461538325, 0.2564102564102563875, 0.2589743589743589980, 0.2615384615384615530, 0.2641025641025641080, 0.2666666666666666630, 0.2692307692307692180, 0.2717948717948717730, 0.2743589743589743835, 0.2769230769230769384, 0.2794871794871794934, 0.2820512820512820484, 0.2846153846153846034, 0.2871794871794871584, 0.2897435897435897689, 0.2923076923076923239, 0.2948717948717948789, 0.2974358974358974339, 0.2999999999999999889, 0.3025641025641025439, 0.3051282051282051544, 0.3076923076923077094, 0.3102564102564102644, 0.3128205128205128194, 0.3153846153846153744, 0.3179487179487179294, 0.3205128205128205399, 0.3230769230769230949, 0.3256410256410256499, 0.3282051282051282048, 0.3307692307692307598, 0.3333333333333333148, 0.3358974358974358698, 0.3384615384615384803, 0.3410256410256410353, 0.3435897435897435903, 0.3461538461538461453, 0.3487179487179487003, 0.3512820512820512553, 0.3538461538461538658, 0.3564102564102564208, 0.3589743589743589758, 0.3615384615384615308, 0.3641025641025640858, 0.3666666666666666408, 0.3692307692307692513, 0.3717948717948718063, 0.3743589743589743613, 0.3769230769230769162, 0.3794871794871794712, 0.3820512820512820262, 0.3846153846153846367, 0.3871794871794871917, 0.3897435897435897467, 0.3923076923076923017, 0.3948717948717948567, 0.3974358974358974117, 0.4000000000000000222, 0.4025641025641025772, 0.4051282051282051322, 0.4076923076923076872, 0.4102564102564102422, 0.4128205128205127972, 0.4153846153846154077, 0.4179487179487179627, 0.4205128205128205177, 0.4230769230769230727, 0.4256410256410256276, 0.4282051282051281826, 0.4307692307692307931, 0.4333333333333333481, 0.4358974358974359031, 0.4384615384615384581, 0.4410256410256410131, 0.4435897435897435681, 0.4461538461538461786, 0.4487179487179487336, 0.4512820512820512886, 0.4538461538461538436, 0.4564102564102563986, 0.4589743589743589536, 0.4615384615384615641, 0.4641025641025641191, 0.4666666666666666741, 0.4692307692307692291, 0.4717948717948717841, 0.4743589743589743390, 0.4769230769230769496, 0.4794871794871795045, 0.4820512820512820595, 0.4846153846153846145, 0.4871794871794871695, 0.4897435897435897245, 0.4923076923076923350, 0.4948717948717948900, 0.4974358974358974450, 0.5000000000000000000, 0.5025641025641025550, 0.5051282051282051100, 0.5076923076923076650, 0.5102564102564102200, 0.5128205128205127750, 0.5153846153846153300, 0.5179487179487179960, 0.5205128205128205510, 0.5230769230769231060, 0.5256410256410256610, 0.5282051282051282159, 0.5307692307692307709, 0.5333333333333333259, 0.5358974358974358809, 0.5384615384615384359, 0.5410256410256409909, 0.5435897435897435459, 0.5461538461538461009, 0.5487179487179487669, 0.5512820512820513219, 0.5538461538461538769, 0.5564102564102564319, 0.5589743589743589869, 0.5615384615384615419, 0.5641025641025640969, 0.5666666666666666519, 0.5692307692307692069, 0.5717948717948717618, 0.5743589743589743168, 0.5769230769230768718, 0.5794871794871795379, 0.5820512820512820928, 0.5846153846153846478, 0.5871794871794872028, 0.5897435897435897578, 0.5923076923076923128, 0.5948717948717948678, 0.5974358974358974228, 0.5999999999999999778, 0.6025641025641025328, 0.6051282051282050878, 0.6076923076923076428, 0.6102564102564103088, 0.6128205128205128638, 0.6153846153846154188, 0.6179487179487179738, 0.6205128205128205288, 0.6230769230769230838, 0.6256410256410256387, 0.6282051282051281937, 0.6307692307692307487, 0.6333333333333333037, 0.6358974358974358587, 0.6384615384615384137, 0.6410256410256410797, 0.6435897435897436347, 0.6461538461538461897, 0.6487179487179487447, 0.6512820512820512997, 0.6538461538461538547, 0.6564102564102564097, 0.6589743589743589647, 0.6615384615384615197, 0.6641025641025640747, 0.6666666666666666297, 0.6692307692307691847, 0.6717948717948717396, 0.6743589743589744057, 0.6769230769230769607, 0.6794871794871795156, 0.6820512820512820706, 0.6846153846153846256, 0.6871794871794871806, 0.6897435897435897356, 0.6923076923076922906, 0.6948717948717948456, 0.6974358974358974006, 0.6999999999999999556, 0.7025641025641025106, 0.7051282051282051766, 0.7076923076923077316, 0.7102564102564102866, 0.7128205128205128416, 0.7153846153846153966, 0.7179487179487179516, 0.7205128205128205066, 0.7230769230769230616, 0.7256410256410256165, 0.7282051282051281715, 0.7307692307692307265, 0.7333333333333332815, 0.7358974358974359475, 0.7384615384615385025, 0.7410256410256410575, 0.7435897435897436125, 0.7461538461538461675, 0.7487179487179487225, 0.7512820512820512775, 0.7538461538461538325, 0.7564102564102563875, 0.7589743589743589425, 0.7615384615384614975, 0.7641025641025640525, 0.7666666666666667185, 0.7692307692307692735, 0.7717948717948718285, 0.7743589743589743835, 0.7769230769230769384, 0.7794871794871794934, 0.7820512820512820484, 0.7846153846153846034, 0.7871794871794871584, 0.7897435897435897134, 0.7923076923076922684, 0.7948717948717948234, 0.7974358974358974894, 0.8000000000000000444, 0.8025641025641025994, 0.8051282051282051544, 0.8076923076923077094, 0.8102564102564102644, 0.8128205128205128194, 0.8153846153846153744, 0.8179487179487179294, 0.8205128205128204844, 0.8230769230769230393, 0.8256410256410255943, 0.8282051282051282604, 0.8307692307692308153, 0.8333333333333333703, 0.8358974358974359253, 0.8384615384615384803, 0.8410256410256410353, 0.8435897435897435903, 0.8461538461538461453, 0.8487179487179487003, 0.8512820512820512553, 0.8538461538461538103, 0.8564102564102563653, 0.8589743589743589203, 0.8615384615384615863, 0.8641025641025641413, 0.8666666666666666963, 0.8692307692307692513, 0.8717948717948718063, 0.8743589743589743613, 0.8769230769230769162, 0.8794871794871794712, 0.8820512820512820262, 0.8846153846153845812, 0.8871794871794871362, 0.8897435897435896912, 0.8923076923076923572, 0.8948717948717949122, 0.8974358974358974672, 0.9000000000000000222, 0.9025641025641025772, 0.9051282051282051322, 0.9076923076923076872, 0.9102564102564102422, 0.9128205128205127972, 0.9153846153846153522, 0.9179487179487179072, 0.9205128205128204621, 0.9230769230769231282, 0.9256410256410256832, 0.9282051282051282382, 0.9307692307692307931, 0.9333333333333333481, 0.9358974358974359031, 0.9384615384615384581, 0.9410256410256410131, 0.9435897435897435681, 0.9461538461538461231, 0.9487179487179486781, 0.9512820512820512331, 0.9538461538461538991, 0.9564102564102564541, 0.9589743589743590091, 0.9615384615384615641, 0.9641025641025641191, 0.9666666666666666741, 0.9692307692307692291, 0.9717948717948717841, 0.9743589743589743390, 0.9769230769230768940, 0.9794871794871794490, 0.9820512820512820040, 0.9846153846153846700, 0.9871794871794872250, 0.9897435897435897800, 0.9923076923076923350, 0.9948717948717948900, 0.9974358974358974450, 1.000000000000000000 ),
 .UNSPECIFIED. ) 
 GEOMETRIC_REPRESENTATION_ITEM ( )  RATIONAL_B_SPLINE_SURFACE ( (
 ( 1.000000000000000000, 0.9510565162951535312, 1.000000000000000000, 0.9510565162951535312, 1.000000000000000000, 0.9510565162951535312, 1.000000000000000000, 0.9510565162951535312, 1.000000000000000000, 0.9510565162951535312, 1.000000000000000000, 0.9510565162951535312, 1.000000000000000000, 0.9510565162951535312, 1.000000000000000000, 0.9510565162951535312, 1.000000000000000000, 0.9510565162951535312, 1.000000000000000000, 0.9510565162951535312, 1.000000000000000000, 0.9510565162951535312, 1.000000000000000000, 0.9510565162951535312, 1.000000000000000000, 0.9510565162951535312, 1.000000000000000000, 0.9510565162951535312, 1.000000000000000000, 0.9510565162951535312, 1.000000000000000000, 0.9510565162951535312, 1.000000000000000000, 0.9510565162951535312, 1.000000000000000000, 0.9510565162951535312, 1.000000000000000000, 0.9510565162951535312, 1.000000000000000000, 0.9510565162951535312, 1.000000000000000000, 0.9510565162951535312, 1.000000000000000000, 0.9510565162951535312, 1.000000000000000000, 0.9510565162951535312, 1.000000000000000000, 0.9510565162951535312, 1.000000000000000000, 0.9510565162951535312, 1.000000000000000000, 0.9510565162951535312, 1.000000000000000000, 0.9510565162951535312, 1.000000000000000000, 0.9510565162951535312, 1.000000000000000000, 0.9510565162951535312, 1.000000000000000000, 0.9510565162951535312, 1.000000000000000000, 0.9510565162951535312, 1.000000000000000000, 0.9510565162951535312, 1.000000000000000000, 0.9510565162951535312, 1.000000000000000000, 0.9510565162951535312, 1.000000000000000000, 0.9510565162951535312, 1.000000000000000000, 0.9510565162951535312, 1.000000000000000000, 0.9510565162951535312, 1.000000000000000000, 0.9510565162951535312, 1.000000000000000000, 0.9510565162951535312, 1.000000000000000000, 0.9510565162951535312, 1.000000000000000000, 0.9510565162951535312, 1.000000000000000000, 0.9510565162951535312, 1.000000000000000000, 0.9510565162951535312, 1.000000000000000000, 0.9510565162951535312, 1.000000000000000000, 0.9510565162951535312, 1.000000000000000000, 0.9510565162951535312, 1.000000000000000000, 0.9510565162951535312, 1.000000000000000000, 0.9510565162951535312, 1.000000000000000000, 0.9510565162951535312, 1.000000000000000000, 0.9510565162951535312, 1.000000000000000000, 0.9510565162951535312, 1.000000000000000000, 0.9510565162951535312, 1.000000000000000000, 0.9510565162951535312, 1.000000000000000000, 0.9510565162951535312, 1.000000000000000000, 0.9510565162951535312, 1.000000000000000000, 0.9510565162951535312, 1.000000000000000000, 0.9510565162951535312, 1.000000000000000000, 0.9510565162951535312, 1.000000000000000000, 0.9510565162951535312, 1.000000000000000000, 0.9510565162951535312, 1.000000000000000000, 0.9510565162951535312, 1.000000000000000000, 0.9510565162951535312, 1.000000000000000000, 0.9510565162951535312, 1.000000000000000000, 0.9510565162951535312, 1.000000000000000000, 0.9510565162951535312, 1.000000000000000000, 0.9510565162951535312, 1.000000000000000000, 0.9510565162951535312, 1.000000000000000000, 0.9510565162951535312, 1.000000000000000000, 0.9510565162951535312, 1.000000000000000000, 0.9510565162951535312, 1.000000000000000000, 0.9510565162951535312, 1.000000000000000000, 0.9510565162951535312, 1.000000000000000000, 0.9510565162951535312, 1.000000000000000000, 0.9510565162951535312, 1.000000000000000000, 0.9510565162951535312, 1.000000000000000000, 0.9510565162951535312, 1.000000000000000000, 0.9510565162951535312, 1.000000000000000000, 0.9510565162951535312, 1.000000000000000000, 0.9510565162951535312, 1.000000000000000000, 0.9510565162951535312, 1.000000000000000000, 0.9510565162951535312, 1.000000000000000000, 0.9510565162951535312, 1.000000000000000000, 0.9510565162951535312, 1.000000000000000000, 0.9510565162951535312, 1.000000000000000000, 0.9510565162951535312, 1.000000000000000000, 0.9510565162951535312, 1.000000000000000000, 0.9510565162951535312, 1.000000000000000000, 0.9510565162951535312, 1.000000000000000000, 0.9510565162951535312, 1.000000000000000000, 0.9510565162951535312, 1.000000000000000000, 0.9510565162951535312, 1.000000000000000000, 0.9510565162951535312, 1.000000000000000000, 0.9510565162951535312, 1.000000000000000000, 0.9510565162951535312, 1.000000000000000000, 0.9510565162951535312, 1.000000000000000000, 0.9510565162951535312, 1.000000000000000000, 0.9510565162951535312, 1.000000000000000000, 0.9510565162951535312, 1.000000000000000000, 0.9510565162951535312, 1.000000000000000000, 0.9510565162951535312, 1.000000000000000000, 0.9510565162951535312, 1.000000000000000000, 0.9510565162951535312, 1.000000000000000000, 0.9510565162951535312, 1.000000000000000000, 0.9510565162951535312, 1.000000000000000000, 0.9510565162951535312, 1.000000000000000000, 0.9510565162951535312, 1.000000000000000000, 0.9510565162951535312, 1.000000000000000000, 0.9510565162951535312, 1.000000000000000000, 0.9510565162951535312, 1.000000000000000000, 0.9510565162951535312, 1.000000000000000000, 0.9510565162951535312, 1.000000000000000000, 0.9510565162951535312, 1.000000000000000000, 0.9510565162951535312, 1.000000000000000000, 0.9510565162951535312, 1.000000000000000000, 0.9510565162951535312, 1.000000000000000000, 0.9510565162951535312, 1.000000000000000000, 0.9510565162951535312, 1.000000000000000000, 0.9510565162951535312, 1.000000000000000000, 0.9510565162951535312, 1.000000000000000000, 0.9510565162951535312, 1.000000000000000000, 0.9510565162951535312, 1.000000000000000000, 0.9510565162951535312, 1.000000000000000000, 0.9510565162951535312, 1.000000000000000000, 0.9510565162951535312, 1.000000000000000000, 0.9510565162951535312, 1.000000000000000000, 0.9510565162951535312, 1.000000000000000000, 0.9510565162951535312, 1.000000000000000000, 0.9510565162951535312, 1.000000000000000000, 0.9510565162951535312, 1.000000000000000000, 0.9510565162951535312, 1.000000000000000000, 0.9510565162951535312, 1.000000000000000000, 0.9510565162951535312, 1.000000000000000000, 0.9510565162951535312, 1.000000000000000000, 0.9510565162951535312, 1.000000000000000000, 0.9510565162951535312, 1.000000000000000000, 0.9510565162951535312, 1.000000000000000000, 0.9510565162951535312, 1.000000000000000000, 0.9510565162951535312, 1.000000000000000000, 0.9510565162951535312, 1.000000000000000000, 0.9510565162951535312, 1.000000000000000000, 0.9510565162951535312, 1.000000000000000000, 0.9510565162951535312, 1.000000000000000000, 0.9510565162951535312, 1.000000000000000000, 0.9510565162951535312, 1.000000000000000000, 0.9510565162951535312, 1.000000000000000000, 0.9510565162951535312, 1.000000000000000000, 0.9510565162951535312, 1.000000000000000000, 0.9510565162951535312, 1.000000000000000000, 0.9510565162951535312, 1.000000000000000000, 0.9510565162951535312, 1.000000000000000000, 0.9510565162951535312, 1.000000000000000000, 0.9510565162951535312, 1.000000000000000000, 0.9510565162951535312, 1.000000000000000000, 0.9510565162951535312, 1.000000000000000000, 0.9510565162951535312, 1.000000000000000000, 0.9510565162951535312, 1.000000000000000000, 0.9510565162951535312, 1.000000000000000000, 0.9510565162951535312, 1.000000000000000000, 0.9510565162951535312, 1.000000000000000000, 0.9510565162951535312, 1.000000000000000000, 0.9510565162951535312, 1.000000000000000000, 0.9510565162951535312, 1.000000000000000000, 0.9510565162951535312, 1.000000000000000000, 0.9510565162951535312, 1.000000000000000000, 0.9510565162951535312, 1.000000000000000000, 0.9510565162951535312, 1.000000000000000000, 0.9510565162951535312, 1.000000000000000000, 0.9510565162951535312, 1.000000000000000000, 0.9510565162951535312, 1.000000000000000000, 0.9510565162951535312, 1.000000000000000000, 0.9510565162951535312, 1.000000000000000000, 0.9510565162951535312, 1.000000000000000000, 0.9510565162951535312, 1.000000000000000000, 0.9510565162951535312, 1.000000000000000000, 0.9510565162951535312, 1.000000000000000000, 0.9510565162951535312, 1.000000000000000000, 0.9510565162951535312, 1.000000000000000000, 0.9510565162951535312, 1.000000000000000000, 0.9510565162951535312, 1.000000000000000000, 0.9510565162951535312, 1.000000000000000000, 0.9510565162951535312, 1.000000000000000000, 0.9510565162951535312, 1.000000000000000000, 0.9510565162951535312, 1.000000000000000000, 0.9510565162951535312, 1.000000000000000000, 0.9510565162951535312, 1.000000000000000000, 0.9510565162951535312, 1.000000000000000000, 0.9510565162951535312, 1.000000000000000000, 0.9510565162951535312, 1.000000000000000000, 0.9510565162951535312, 1.000000000000000000, 0.9510565162951535312, 1.000000000000000000, 0.9510565162951535312, 1.000000000000000000, 0.9510565162951535312, 1.000000000000000000, 0.9510565162951535312, 1.000000000000000000, 0.9510565162951535312, 1.000000000000000000, 0.9510565162951535312, 1.000000000000000000, 0.9510565162951535312, 1.000000000000000000, 0.9510565162951535312, 1.000000000000000000, 0.9510565162951535312, 1.000000000000000000, 0.9510565162951535312, 1.000000000000000000, 0.9510565162951535312, 1.000000000000000000, 0.9510565162951535312, 1.000000000000000000, 0.9510565162951535312, 1.000000000000000000, 0.9510565162951535312, 1.000000000000000000, 0.9510565162951535312, 1.000000000000000000, 0.9510565162951535312, 1.000000000000000000, 0.9510565162951535312, 1.000000000000000000, 0.9510565162951535312, 1.000000000000000000, 0.9510565162951535312, 1.000000000000000000, 0.9510565162951535312, 1.000000000000000000, 0.9510565162951535312, 1.000000000000000000, 0.9510565162951535312, 1.000000000000000000, 0.9510565162951535312, 1.000000000000000000, 0.9510565162951535312, 1.000000000000000000, 0.9510565162951535312, 1.000000000000000000, 0.9510565162951535312, 1.000000000000000000, 0.9510565162951535312, 1.000000000000000000, 0.9510565162951535312, 1.000000000000000000, 0.9510565162951535312, 1.000000000000000000, 0.9510565162951535312, 1.000000000000000000, 0.9510565162951535312, 1.000000000000000000, 0.9510565162951535312, 1.000000000000000000, 0.9510565162951535312, 1.000000000000000000, 0.9510565162951535312, 1.000000000000000000, 0.9510565162951535312, 1.000000000000000000, 0.9510565162951535312, 1.000000000000000000, 0.9510565162951535312, 1.000000000000000000, 0.9510565162951535312, 1.000000000000000000, 0.9510565162951535312, 1.000000000000000000, 0.9510565162951535312, 1.000000000000000000, 0.9510565162951535312, 1.000000000000000000, 0.9510565162951535312, 1.000000000000000000, 0.9510565162951535312, 1.000000000000000000, 0.9510565162951535312, 1.000000000000000000, 0.9510565162951535312, 1.000000000000000000, 0.9510565162951535312, 1.000000000000000000, 0.9510565162951535312, 1.000000000000000000, 0.9510565162951535312, 1.000000000000000000, 0.9510565162951535312, 1.000000000000000000, 0.9510565162951535312, 1.000000000000000000, 0.9510565162951535312, 1.000000000000000000, 0.9510565162951535312, 1.000000000000000000, 0.9510565162951535312, 1.000000000000000000, 0.9510565162951535312, 1.000000000000000000, 0.9510565162951535312, 1.000000000000000000, 0.9510565162951535312, 1.000000000000000000, 0.9510565162951535312, 1.000000000000000000, 0.9510565162951535312, 1.000000000000000000, 0.9510565162951535312, 1.000000000000000000, 0.9510565162951535312, 1.000000000000000000, 0.9510565162951535312, 1.000000000000000000, 0.9510565162951535312, 1.000000000000000000, 0.9510565162951535312, 1.000000000000000000, 0.9510565162951535312, 1.000000000000000000, 0.9510565162951535312, 1.000000000000000000, 0.9510565162951535312, 1.000000000000000000, 0.9510565162951535312, 1.000000000000000000, 0.9510565162951535312, 1.000000000000000000, 0.9510565162951535312, 1.000000000000000000, 0.9510565162951535312, 1.000000000000000000, 0.9510565162951535312, 1.000000000000000000, 0.9510565162951535312, 1.000000000000000000, 0.9510565162951535312, 1.000000000000000000, 0.9510565162951535312, 1.000000000000000000, 0.9510565162951535312, 1.000000000000000000, 0.9510565162951535312, 1.000000000000000000, 0.9510565162951535312, 1.000000000000000000, 0.9510565162951535312, 1.000000000000000000, 0.9510565162951535312, 1.000000000000000000, 0.9510565162951535312, 1.000000000000000000, 0.9510565162951535312, 1.000000000000000000, 0.9510565162951535312, 1.000000000000000000, 0.9510565162951535312, 1.000000000000000000, 0.9510565162951535312, 1.000000000000000000, 0.9510565162951535312, 1.000000000000000000, 0.9510565162951535312, 1.000000000000000000, 0.9510565162951535312, 1.000000000000000000, 0.9510565162951535312, 1.000000000000000000, 0.9510565162951535312, 1.000000000000000000, 0.9510565162951535312, 1.000000000000000000, 0.9510565162951535312, 1.000000000000000000, 0.9510565162951535312, 1.000000000000000000, 0.9510565162951535312, 1.000000000000000000, 0.9510565162951535312, 1.000000000000000000, 0.9510565162951535312, 1.000000000000000000, 0.9510565162951535312, 1.000000000000000000, 0.9510565162951535312, 1.000000000000000000, 0.9510565162951535312, 1.000000000000000000, 0.9510565162951535312, 1.000000000000000000, 0.9510565162951535312, 1.000000000000000000, 0.9510565162951535312, 1.000000000000000000, 0.9510565162951535312, 1.000000000000000000, 0.9510565162951535312, 1.000000000000000000, 0.9510565162951535312, 1.000000000000000000, 0.9510565162951535312, 1.000000000000000000, 0.9510565162951535312, 1.000000000000000000, 0.9510565162951535312, 1.000000000000000000, 0.9510565162951535312, 1.000000000000000000, 0.9510565162951535312, 1.000000000000000000, 0.9510565162951535312, 1.000000000000000000, 0.9510565162951535312, 1.000000000000000000, 0.9510565162951535312, 1.000000000000000000, 0.9510565162951535312, 1.000000000000000000, 0.9510565162951535312, 1.000000000000000000, 0.9510565162951535312, 1.000000000000000000, 0.9510565162951535312, 1.000000000000000000, 0.9510565162951535312, 1.000000000000000000, 0.9510565162951535312, 1.000000000000000000, 0.9510565162951535312, 1.000000000000000000, 0.9510565162951535312, 1.000000000000000000, 0.9510565162951535312, 1.000000000000000000, 0.9510565162951535312, 1.000000000000000000, 0.9510565162951535312, 1.000000000000000000, 0.9510565162951535312, 1.000000000000000000, 0.9510565162951535312, 1.000000000000000000, 0.9510565162951535312, 1.000000000000000000, 0.9510565162951535312, 1.000000000000000000, 0.9510565162951535312, 1.000000000000000000, 0.9510565162951535312, 1.000000000000000000, 0.9510565162951535312, 1.000000000000000000, 0.9510565162951535312, 1.000000000000000000, 0.9510565162951535312, 1.000000000000000000, 0.9510565162951535312, 1.000000000000000000, 0.9510565162951535312, 1.000000000000000000, 0.9510565162951535312, 1.000000000000000000, 0.9510565162951535312, 1.000000000000000000, 0.9510565162951535312, 1.000000000000000000, 0.9510565162951535312, 1.000000000000000000, 0.9510565162951535312, 1.000000000000000000, 0.9510565162951535312, 1.000000000000000000, 0.9510565162951535312, 1.000000000000000000, 0.9510565162951535312, 1.000000000000000000, 0.9510565162951535312, 1.000000000000000000, 0.9510565162951535312, 1.000000000000000000, 0.9510565162951535312, 1.000000000000000000, 0.9510565162951535312, 1.000000000000000000, 0.9510565162951535312, 1.000000000000000000, 0.9510565162951535312, 1.000000000000000000, 0.9510565162951535312, 1.000000000000000000, 0.9510565162951535312, 1.000000000000000000, 0.9510565162951535312, 1.000000000000000000, 0.9510565162951535312, 1.000000000000000000, 0.9510565162951535312, 1.000000000000000000, 0.9510565162951535312, 1.000000000000000000, 0.9510565162951535312, 1.000000000000000000, 0.9510565162951535312, 1.000000000000000000, 0.9510565162951535312, 1.000000000000000000, 0.9510565162951535312, 1.000000000000000000, 0.9510565162951535312, 1.000000000000000000, 0.9510565162951535312, 1.000000000000000000, 0.9510565162951535312, 1.000000000000000000, 0.9510565162951535312, 1.000000000000000000, 0.9510565162951535312, 1.000000000000000000, 0.9510565162951535312, 1.000000000000000000, 0.9510565162951535312, 1.000000000000000000, 0.9510565162951535312, 1.000000000000000000, 0.9510565162951535312, 1.000000000000000000, 0.9510565162951535312, 1.000000000000000000, 0.9510565162951535312, 1.000000000000000000, 0.9510565162951535312, 1.000000000000000000, 0.9510565162951535312, 1.000000000000000000, 0.9510565162951535312, 1.000000000000000000, 0.9510565162951535312, 1.000000000000000000, 0.9510565162951535312, 1.000000000000000000, 0.9510565162951535312, 1.000000000000000000, 0.9510565162951535312, 1.000000000000000000, 0.9510565162951535312, 1.000000000000000000, 0.9510565162951535312, 1.000000000000000000, 0.9510565162951535312, 1.000000000000000000, 0.9510565162951535312, 1.000000000000000000, 0.9510565162951535312, 1.000000000000000000, 0.9510565162951535312, 1.000000000000000000, 0.9510565162951535312, 1.000000000000000000, 0.9510565162951535312, 1.000000000000000000, 0.9510565162951535312, 1.000000000000000000, 0.9510565162951535312, 1.000000000000000000, 0.9510565162951535312, 1.000000000000000000, 0.9510565162951535312, 1.000000000000000000, 0.9510565162951535312, 1.000000000000000000, 0.9510565162951535312, 1.000000000000000000, 0.9510565162951535312, 1.000000000000000000, 0.9510565162951535312, 1.000000000000000000, 0.9510565162951535312, 1.000000000000000000, 0.9510565162951535312, 1.000000000000000000, 0.9510565162951535312, 1.000000000000000000, 0.9510565162951535312, 1.000000000000000000, 0.9510565162951535312, 1.000000000000000000, 0.9510565162951535312, 1.000000000000000000, 0.9510565162951535312, 1.000000000000000000, 0.9510565162951535312, 1.000000000000000000, 0.9510565162951535312, 1.000000000000000000),
 ( 1.000000000000000000, 0.9510565162951535312, 1.000000000000000000, 0.9510565162951535312, 1.000000000000000000, 0.9510565162951535312, 1.000000000000000000, 0.9510565162951535312, 1.000000000000000000, 0.9510565162951535312, 1.000000000000000000, 0.9510565162951535312, 1.000000000000000000, 0.9510565162951535312, 1.000000000000000000, 0.9510565162951535312, 1.000000000000000000, 0.9510565162951535312, 1.000000000000000000, 0.9510565162951535312, 1.000000000000000000, 0.9510565162951535312, 1.000000000000000000, 0.9510565162951535312, 1.000000000000000000, 0.9510565162951535312, 1.000000000000000000, 0.9510565162951535312, 1.000000000000000000, 0.9510565162951535312, 1.000000000000000000, 0.9510565162951535312, 1.000000000000000000, 0.9510565162951535312, 1.000000000000000000, 0.9510565162951535312, 1.000000000000000000, 0.9510565162951535312, 1.000000000000000000, 0.9510565162951535312, 1.000000000000000000, 0.9510565162951535312, 1.000000000000000000, 0.9510565162951535312, 1.000000000000000000, 0.9510565162951535312, 1.000000000000000000, 0.9510565162951535312, 1.000000000000000000, 0.9510565162951535312, 1.000000000000000000, 0.9510565162951535312, 1.000000000000000000, 0.9510565162951535312, 1.000000000000000000, 0.9510565162951535312, 1.000000000000000000, 0.9510565162951535312, 1.000000000000000000, 0.9510565162951535312, 1.000000000000000000, 0.9510565162951535312, 1.000000000000000000, 0.9510565162951535312, 1.000000000000000000, 0.9510565162951535312, 1.000000000000000000, 0.9510565162951535312, 1.000000000000000000, 0.9510565162951535312, 1.000000000000000000, 0.9510565162951535312, 1.000000000000000000, 0.9510565162951535312, 1.000000000000000000, 0.9510565162951535312, 1.000000000000000000, 0.9510565162951535312, 1.000000000000000000, 0.9510565162951535312, 1.000000000000000000, 0.9510565162951535312, 1.000000000000000000, 0.9510565162951535312, 1.000000000000000000, 0.9510565162951535312, 1.000000000000000000, 0.9510565162951535312, 1.000000000000000000, 0.9510565162951535312, 1.000000000000000000, 0.9510565162951535312, 1.000000000000000000, 0.9510565162951535312, 1.000000000000000000, 0.9510565162951535312, 1.000000000000000000, 0.9510565162951535312, 1.000000000000000000, 0.9510565162951535312, 1.000000000000000000, 0.9510565162951535312, 1.000000000000000000, 0.9510565162951535312, 1.000000000000000000, 0.9510565162951535312, 1.000000000000000000, 0.9510565162951535312, 1.000000000000000000, 0.9510565162951535312, 1.000000000000000000, 0.9510565162951535312, 1.000000000000000000, 0.9510565162951535312, 1.000000000000000000, 0.9510565162951535312, 1.000000000000000000, 0.9510565162951535312, 1.000000000000000000, 0.9510565162951535312, 1.000000000000000000, 0.9510565162951535312, 1.000000000000000000, 0.9510565162951535312, 1.000000000000000000, 0.9510565162951535312, 1.000000000000000000, 0.9510565162951535312, 1.000000000000000000, 0.9510565162951535312, 1.000000000000000000, 0.9510565162951535312, 1.000000000000000000, 0.9510565162951535312, 1.000000000000000000, 0.9510565162951535312, 1.000000000000000000, 0.9510565162951535312, 1.000000000000000000, 0.9510565162951535312, 1.000000000000000000, 0.9510565162951535312, 1.000000000000000000, 0.9510565162951535312, 1.000000000000000000, 0.9510565162951535312, 1.000000000000000000, 0.9510565162951535312, 1.000000000000000000, 0.9510565162951535312, 1.000000000000000000, 0.9510565162951535312, 1.000000000000000000, 0.9510565162951535312, 1.000000000000000000, 0.9510565162951535312, 1.000000000000000000, 0.9510565162951535312, 1.000000000000000000, 0.9510565162951535312, 1.000000000000000000, 0.9510565162951535312, 1.000000000000000000, 0.9510565162951535312, 1.000000000000000000, 0.9510565162951535312, 1.000000000000000000, 0.9510565162951535312, 1.000000000000000000, 0.9510565162951535312, 1.000000000000000000, 0.9510565162951535312, 1.000000000000000000, 0.9510565162951535312, 1.000000000000000000, 0.9510565162951535312, 1.000000000000000000, 0.9510565162951535312, 1.000000000000000000, 0.9510565162951535312, 1.000000000000000000, 0.9510565162951535312, 1.000000000000000000, 0.9510565162951535312, 1.000000000000000000, 0.9510565162951535312, 1.000000000000000000, 0.9510565162951535312, 1.000000000000000000, 0.9510565162951535312, 1.000000000000000000, 0.9510565162951535312, 1.000000000000000000, 0.9510565162951535312, 1.000000000000000000, 0.9510565162951535312, 1.000000000000000000, 0.9510565162951535312, 1.000000000000000000, 0.9510565162951535312, 1.000000000000000000, 0.9510565162951535312, 1.000000000000000000, 0.9510565162951535312, 1.000000000000000000, 0.9510565162951535312, 1.000000000000000000, 0.9510565162951535312, 1.000000000000000000, 0.9510565162951535312, 1.000000000000000000, 0.9510565162951535312, 1.000000000000000000, 0.9510565162951535312, 1.000000000000000000, 0.9510565162951535312, 1.000000000000000000, 0.9510565162951535312, 1.000000000000000000, 0.9510565162951535312, 1.000000000000000000, 0.9510565162951535312, 1.000000000000000000, 0.9510565162951535312, 1.000000000000000000, 0.9510565162951535312, 1.000000000000000000, 0.9510565162951535312, 1.000000000000000000, 0.9510565162951535312, 1.000000000000000000, 0.9510565162951535312, 1.000000000000000000, 0.9510565162951535312, 1.000000000000000000, 0.9510565162951535312, 1.000000000000000000, 0.9510565162951535312, 1.000000000000000000, 0.9510565162951535312, 1.000000000000000000, 0.9510565162951535312, 1.000000000000000000, 0.9510565162951535312, 1.000000000000000000, 0.9510565162951535312, 1.000000000000000000, 0.9510565162951535312, 1.000000000000000000, 0.9510565162951535312, 1.000000000000000000, 0.9510565162951535312, 1.000000000000000000, 0.9510565162951535312, 1.000000000000000000, 0.9510565162951535312, 1.000000000000000000, 0.9510565162951535312, 1.000000000000000000, 0.9510565162951535312, 1.000000000000000000, 0.9510565162951535312, 1.000000000000000000, 0.9510565162951535312, 1.000000000000000000, 0.9510565162951535312, 1.000000000000000000, 0.9510565162951535312, 1.000000000000000000, 0.9510565162951535312, 1.000000000000000000, 0.9510565162951535312, 1.000000000000000000, 0.9510565162951535312, 1.000000000000000000, 0.9510565162951535312, 1.000000000000000000, 0.9510565162951535312, 1.000000000000000000, 0.9510565162951535312, 1.000000000000000000, 0.9510565162951535312, 1.000000000000000000, 0.9510565162951535312, 1.000000000000000000, 0.9510565162951535312, 1.000000000000000000, 0.9510565162951535312, 1.000000000000000000, 0.9510565162951535312, 1.000000000000000000, 0.9510565162951535312, 1.000000000000000000, 0.9510565162951535312, 1.000000000000000000, 0.9510565162951535312, 1.000000000000000000, 0.9510565162951535312, 1.000000000000000000, 0.9510565162951535312, 1.000000000000000000, 0.9510565162951535312, 1.000000000000000000, 0.9510565162951535312, 1.000000000000000000, 0.9510565162951535312, 1.000000000000000000, 0.9510565162951535312, 1.000000000000000000, 0.9510565162951535312, 1.000000000000000000, 0.9510565162951535312, 1.000000000000000000, 0.9510565162951535312, 1.000000000000000000, 0.9510565162951535312, 1.000000000000000000, 0.9510565162951535312, 1.000000000000000000, 0.9510565162951535312, 1.000000000000000000, 0.9510565162951535312, 1.000000000000000000, 0.9510565162951535312, 1.000000000000000000, 0.9510565162951535312, 1.000000000000000000, 0.9510565162951535312, 1.000000000000000000, 0.9510565162951535312, 1.000000000000000000, 0.9510565162951535312, 1.000000000000000000, 0.9510565162951535312, 1.000000000000000000, 0.9510565162951535312, 1.000000000000000000, 0.9510565162951535312, 1.000000000000000000, 0.9510565162951535312, 1.000000000000000000, 0.9510565162951535312, 1.000000000000000000, 0.9510565162951535312, 1.000000000000000000, 0.9510565162951535312, 1.000000000000000000, 0.9510565162951535312, 1.000000000000000000, 0.9510565162951535312, 1.000000000000000000, 0.9510565162951535312, 1.000000000000000000, 0.9510565162951535312, 1.000000000000000000, 0.9510565162951535312, 1.000000000000000000, 0.9510565162951535312, 1.000000000000000000, 0.9510565162951535312, 1.000000000000000000, 0.9510565162951535312, 1.000000000000000000, 0.9510565162951535312, 1.000000000000000000, 0.9510565162951535312, 1.000000000000000000, 0.9510565162951535312, 1.000000000000000000, 0.9510565162951535312, 1.000000000000000000, 0.9510565162951535312, 1.000000000000000000, 0.9510565162951535312, 1.000000000000000000, 0.9510565162951535312, 1.000000000000000000, 0.9510565162951535312, 1.000000000000000000, 0.9510565162951535312, 1.000000000000000000, 0.9510565162951535312, 1.000000000000000000, 0.9510565162951535312, 1.000000000000000000, 0.9510565162951535312, 1.000000000000000000, 0.9510565162951535312, 1.000000000000000000, 0.9510565162951535312, 1.000000000000000000, 0.9510565162951535312, 1.000000000000000000, 0.9510565162951535312, 1.000000000000000000, 0.9510565162951535312, 1.000000000000000000, 0.9510565162951535312, 1.000000000000000000, 0.9510565162951535312, 1.000000000000000000, 0.9510565162951535312, 1.000000000000000000, 0.9510565162951535312, 1.000000000000000000, 0.9510565162951535312, 1.000000000000000000, 0.9510565162951535312, 1.000000000000000000, 0.9510565162951535312, 1.000000000000000000, 0.9510565162951535312, 1.000000000000000000, 0.9510565162951535312, 1.000000000000000000, 0.9510565162951535312, 1.000000000000000000, 0.9510565162951535312, 1.000000000000000000, 0.9510565162951535312, 1.000000000000000000, 0.9510565162951535312, 1.000000000000000000, 0.9510565162951535312, 1.000000000000000000, 0.9510565162951535312, 1.000000000000000000, 0.9510565162951535312, 1.000000000000000000, 0.9510565162951535312, 1.000000000000000000, 0.9510565162951535312, 1.000000000000000000, 0.9510565162951535312, 1.000000000000000000, 0.9510565162951535312, 1.000000000000000000, 0.9510565162951535312, 1.000000000000000000, 0.9510565162951535312, 1.000000000000000000, 0.9510565162951535312, 1.000000000000000000, 0.9510565162951535312, 1.000000000000000000, 0.9510565162951535312, 1.000000000000000000, 0.9510565162951535312, 1.000000000000000000, 0.9510565162951535312, 1.000000000000000000, 0.9510565162951535312, 1.000000000000000000, 0.9510565162951535312, 1.000000000000000000, 0.9510565162951535312, 1.000000000000000000, 0.9510565162951535312, 1.000000000000000000, 0.9510565162951535312, 1.000000000000000000, 0.9510565162951535312, 1.000000000000000000, 0.9510565162951535312, 1.000000000000000000, 0.9510565162951535312, 1.000000000000000000, 0.9510565162951535312, 1.000000000000000000, 0.9510565162951535312, 1.000000000000000000, 0.9510565162951535312, 1.000000000000000000, 0.9510565162951535312, 1.000000000000000000, 0.9510565162951535312, 1.000000000000000000, 0.9510565162951535312, 1.000000000000000000, 0.9510565162951535312, 1.000000000000000000, 0.9510565162951535312, 1.000000000000000000, 0.9510565162951535312, 1.000000000000000000, 0.9510565162951535312, 1.000000000000000000, 0.9510565162951535312, 1.000000000000000000, 0.9510565162951535312, 1.000000000000000000, 0.9510565162951535312, 1.000000000000000000, 0.9510565162951535312, 1.000000000000000000, 0.9510565162951535312, 1.000000000000000000, 0.9510565162951535312, 1.000000000000000000, 0.9510565162951535312, 1.000000000000000000, 0.9510565162951535312, 1.000000000000000000, 0.9510565162951535312, 1.000000000000000000, 0.9510565162951535312, 1.000000000000000000, 0.9510565162951535312, 1.000000000000000000, 0.9510565162951535312, 1.000000000000000000, 0.9510565162951535312, 1.000000000000000000, 0.9510565162951535312, 1.000000000000000000, 0.9510565162951535312, 1.000000000000000000, 0.9510565162951535312, 1.000000000000000000, 0.9510565162951535312, 1.000000000000000000, 0.9510565162951535312, 1.000000000000000000, 0.9510565162951535312, 1.000000000000000000, 0.9510565162951535312, 1.000000000000000000, 0.9510565162951535312, 1.000000000000000000, 0.9510565162951535312, 1.000000000000000000, 0.9510565162951535312, 1.000000000000000000, 0.9510565162951535312, 1.000000000000000000, 0.9510565162951535312, 1.000000000000000000, 0.9510565162951535312, 1.000000000000000000, 0.9510565162951535312, 1.000000000000000000, 0.9510565162951535312, 1.000000000000000000, 0.9510565162951535312, 1.000000000000000000, 0.9510565162951535312, 1.000000000000000000, 0.9510565162951535312, 1.000000000000000000, 0.9510565162951535312, 1.000000000000000000, 0.9510565162951535312, 1.000000000000000000, 0.9510565162951535312, 1.000000000000000000, 0.9510565162951535312, 1.000000000000000000, 0.9510565162951535312, 1.000000000000000000, 0.9510565162951535312, 1.000000000000000000, 0.9510565162951535312, 1.000000000000000000, 0.9510565162951535312, 1.000000000000000000, 0.9510565162951535312, 1.000000000000000000, 0.9510565162951535312, 1.000000000000000000, 0.9510565162951535312, 1.000000000000000000, 0.9510565162951535312, 1.000000000000000000, 0.9510565162951535312, 1.000000000000000000, 0.9510565162951535312, 1.000000000000000000, 0.9510565162951535312, 1.000000000000000000, 0.9510565162951535312, 1.000000000000000000, 0.9510565162951535312, 1.000000000000000000, 0.9510565162951535312, 1.000000000000000000, 0.9510565162951535312, 1.000000000000000000, 0.9510565162951535312, 1.000000000000000000, 0.9510565162951535312, 1.000000000000000000, 0.9510565162951535312, 1.000000000000000000, 0.9510565162951535312, 1.000000000000000000, 0.9510565162951535312, 1.000000000000000000, 0.9510565162951535312, 1.000000000000000000, 0.9510565162951535312, 1.000000000000000000, 0.9510565162951535312, 1.000000000000000000, 0.9510565162951535312, 1.000000000000000000, 0.9510565162951535312, 1.000000000000000000, 0.9510565162951535312, 1.000000000000000000, 0.9510565162951535312, 1.000000000000000000, 0.9510565162951535312, 1.000000000000000000, 0.9510565162951535312, 1.000000000000000000, 0.9510565162951535312, 1.000000000000000000, 0.9510565162951535312, 1.000000000000000000, 0.9510565162951535312, 1.000000000000000000, 0.9510565162951535312, 1.000000000000000000, 0.9510565162951535312, 1.000000000000000000, 0.9510565162951535312, 1.000000000000000000, 0.9510565162951535312, 1.000000000000000000, 0.9510565162951535312, 1.000000000000000000, 0.9510565162951535312, 1.000000000000000000, 0.9510565162951535312, 1.000000000000000000, 0.9510565162951535312, 1.000000000000000000, 0.9510565162951535312, 1.000000000000000000, 0.9510565162951535312, 1.000000000000000000, 0.9510565162951535312, 1.000000000000000000, 0.9510565162951535312, 1.000000000000000000, 0.9510565162951535312, 1.000000000000000000, 0.9510565162951535312, 1.000000000000000000, 0.9510565162951535312, 1.000000000000000000, 0.9510565162951535312, 1.000000000000000000, 0.9510565162951535312, 1.000000000000000000, 0.9510565162951535312, 1.000000000000000000, 0.9510565162951535312, 1.000000000000000000, 0.9510565162951535312, 1.000000000000000000, 0.9510565162951535312, 1.000000000000000000, 0.9510565162951535312, 1.000000000000000000, 0.9510565162951535312, 1.000000000000000000, 0.9510565162951535312, 1.000000000000000000, 0.9510565162951535312, 1.000000000000000000, 0.9510565162951535312, 1.000000000000000000, 0.9510565162951535312, 1.000000000000000000, 0.9510565162951535312, 1.000000000000000000, 0.9510565162951535312, 1.000000000000000000, 0.9510565162951535312, 1.000000000000000000, 0.9510565162951535312, 1.000000000000000000, 0.9510565162951535312, 1.000000000000000000, 0.9510565162951535312, 1.000000000000000000, 0.9510565162951535312, 1.000000000000000000, 0.9510565162951535312, 1.000000000000000000, 0.9510565162951535312, 1.000000000000000000, 0.9510565162951535312, 1.000000000000000000, 0.9510565162951535312, 1.000000000000000000, 0.9510565162951535312, 1.000000000000000000, 0.9510565162951535312, 1.000000000000000000, 0.9510565162951535312, 1.000000000000000000, 0.9510565162951535312, 1.000000000000000000, 0.9510565162951535312, 1.000000000000000000, 0.9510565162951535312, 1.000000000000000000, 0.9510565162951535312, 1.000000000000000000, 0.9510565162951535312, 1.000000000000000000, 0.9510565162951535312, 1.000000000000000000, 0.9510565162951535312, 1.000000000000000000, 0.9510565162951535312, 1.000000000000000000, 0.9510565162951535312, 1.000000000000000000, 0.9510565162951535312, 1.000000000000000000, 0.9510565162951535312, 1.000000000000000000, 0.9510565162951535312, 1.000000000000000000, 0.9510565162951535312, 1.000000000000000000, 0.9510565162951535312, 1.000000000000000000, 0.9510565162951535312, 1.000000000000000000, 0.9510565162951535312, 1.000000000000000000, 0.9510565162951535312, 1.000000000000000000, 0.9510565162951535312, 1.000000000000000000, 0.9510565162951535312, 1.000000000000000000, 0.9510565162951535312, 1.000000000000000000, 0.9510565162951535312, 1.000000000000000000, 0.9510565162951535312, 1.000000000000000000, 0.9510565162951535312, 1.000000000000000000, 0.9510565162951535312, 1.000000000000000000, 0.9510565162951535312, 1.000000000000000000, 0.9510565162951535312, 1.000000000000000000, 0.9510565162951535312, 1.000000000000000000, 0.9510565162951535312, 1.000000000000000000, 0.9510565162951535312, 1.000000000000000000, 0.9510565162951535312, 1.000000000000000000, 0.9510565162951535312, 1.000000000000000000, 0.9510565162951535312, 1.000000000000000000, 0.9510565162951535312, 1.000000000000000000, 0.9510565162951535312, 1.000000000000000000, 0.9510565162951535312, 1.000000000000000000, 0.9510565162951535312, 1.000000000000000000, 0.9510565162951535312, 1.000000000000000000, 0.9510565162951535312, 1.000000000000000000, 0.9510565162951535312, 1.000000000000000000) ) ) 
 REPRESENTATION_ITEM ( '' )  SURFACE ( )  );
#20825=CYLINDRICAL_SURFACE ( 'NONE', #10747, 32.50000000000000000 ) ;
#20830=CARTESIAN_POINT ( 'NONE',  ( -20.75514604977248112, 73.67500000273120975, 28.56700777964554661 ) ) ;
#20834=CARTESIAN_POINT ( 'NONE',  ( -27.16883889988623935, 55.32500000273120122, 19.73931689729374739 ) ) ;
#20835=CARTESIAN_POINT ( 'NONE',  ( 10.37757302488624056, 18.77500000273117564, -31.93888565452638417 ) ) ;
#20836=CARTESIAN_POINT ( 'NONE',  ( 27.16883889988623935, 4.575000002731186122, -19.73931689729374384 ) ) ;
#20840=CARTESIAN_POINT ( 'NONE',  ( -20.08610463437157989, 76.20000000546235697, -27.64615127144129758 ) ) ;
#20841=CARTESIAN_POINT ( 'NONE',  ( 14.41072458151315594, 52.00000000000000000, -29.41684567868830769 ) ) ;
#20846=CARTESIAN_POINT ( 'NONE',  ( 33.58253175000000113, 52.47500000273117138, -10.91162601494193751 ) ) ;
#20850=VERTEX_POINT ( 'NONE', #27291 ) ;
#20851=CARTESIAN_POINT ( 'NONE',  ( -33.58253175000000113, 23.22500000273117138, 10.91162601494193929 ) ) ;
#20864=CARTESIAN_POINT ( 'NONE',  ( -26.29305231718579350, 59.80000000000000426, -19.10302069950537884 ) ) ;
#20865=CARTESIAN_POINT ( 'NONE',  ( 26.29305231718578995, 17.19999999999997797, -19.10302069950538240 ) ) ;
#20872=CARTESIAN_POINT ( 'NONE',  ( 20.75514604977248467, 70.42500000273119554, -28.56700777964554305 ) ) ;
#20873=CARTESIAN_POINT ( 'NONE',  ( -20.75514604977248112, 33.67500000273119554, 28.56700777964554661 ) ) ;
#20879=CARTESIAN_POINT ( 'NONE',  ( -32.50000000000000000, 59.89999999999999858, -10.55989012756945478 ) ) ;
#20883=CARTESIAN_POINT ( 'NONE',  ( -10.37757302488623701, 71.77500000273118985, 31.93888565452638417 ) ) ;
#20888=CARTESIAN_POINT ( 'NONE',  ( 10.37757302488624767, 43.72500000273120691, 31.93888565452638417 ) ) ;
#20892=CARTESIAN_POINT ( 'NONE',  ( -2.092463501923844636E-15, 2.000000005462382102, -34.17252228774368916 ) ) ;
#20909=CARTESIAN_POINT ( 'NONE',  ( -27.16883889988623935, 57.57500000273117990, 19.73931689729374739 ) ) ;
#20917=CARTESIAN_POINT ( 'NONE',  ( 20.75514604977249178, 17.82500000273120122, 28.56700777964553950 ) ) ;
#20923=CARTESIAN_POINT ( 'NONE',  ( 6.277390505771533514E-15, 35.00000000546237544, 34.17252228774368916 ) ) ;
#20930=CARTESIAN_POINT ( 'NONE',  ( 20.75514604977249178, 63.82500000273119412, 28.56700777964553950 ) ) ;
#20931=ADVANCED_FACE ( 'NONE', ( #16496 ), #5858, .F. ) ;
#20936=CARTESIAN_POINT ( 'NONE',  ( -27.16883889988623935, 7.325000002731188786, 19.73931689729374739 ) ) ;
#20946=CARTESIAN_POINT ( 'NONE',  ( -10.04305231718579172, 27.59999999999999787, -30.90933677959248982 ) ) ;
#20958=CARTESIAN_POINT ( 'NONE',  ( 20.75514604977249178, 31.82500000273119056, 28.56700777964553950 ) ) ;
#20963=CARTESIAN_POINT ( 'NONE',  ( -10.04305231718579172, 56.10000000546237686, -30.90933677959248982 ) ) ;
#20969=CARTESIAN_POINT ( 'NONE',  ( 20.75514604977249178, 36.07500000273117990, 28.56700777964553950 ) ) ;
#20973=VECTOR ( 'NONE', #3042, 1000.000000000000000 ) ;
#20974=CARTESIAN_POINT ( 'NONE',  ( -2.092463501923844636E-15, 18.00000000546237189, -34.17252228774368916 ) ) ;
#20985=CARTESIAN_POINT ( 'NONE',  ( 6.486482029760648627E-15, 61.62500000273118417, 35.31076352940722529 ) ) ;
#20990=AXIS2_PLACEMENT_3D ( 'NONE', #33647, #7563, #26095 ) ;
#20991=LINE ( 'NONE', #28864, #24427 ) ;
#20996=CARTESIAN_POINT ( 'NONE',  ( 10.37757302488624767, 73.97500000273120691, 31.93888565452638417 ) ) ;
#21000=CARTESIAN_POINT ( 'NONE',  ( 33.58253175000000823, 54.02500000273118275, 10.91162601494192863 ) ) ;
#21001=CARTESIAN_POINT ( 'NONE',  ( 33.58253175000000113, 20.47500000273120335, -10.91162601494193751 ) ) ;
#21002=CARTESIAN_POINT ( 'NONE',  ( 20.75514604977248467, 6.675000002731186655, -28.56700777964554305 ) ) ;
#21006=CARTESIAN_POINT ( 'NONE',  ( 10.04305231718579705, 71.10000000546239107, 30.90933677959248982 ) ) ;
#21007=CARTESIAN_POINT ( 'NONE',  ( 5.393181536354239469, 52.00000000000000711, -32.17179393301736923 ) ) ;
#21012=ORIENTED_EDGE ( 'NONE', *, *, #19074, .F. ) ;
#21013=CARTESIAN_POINT ( 'NONE',  ( -27.16883889988623935, 55.57500000273117280, 19.73931689729374739 ) ) ;
#21018=CARTESIAN_POINT ( 'NONE',  ( -33.58253175000000113, 23.12500000273119838, 0.000000000000000000 ) ) ;
#21023=DIRECTION ( 'NONE',  ( 0.000000000000000000, 1.000000000000000000, 0.000000000000000000 ) ) ;
#21035=CARTESIAN_POINT ( 'NONE',  ( -20.08610463437156923, 16.29999999999997584, 27.64615127144130113 ) ) ;
#21041=CARTESIAN_POINT ( 'NONE',  ( -33.58253175000000113, 73.02500000273120406, -10.91162601494193218 ) ) ;
#21042=CARTESIAN_POINT ( 'NONE',  ( -2.162160676586881955E-15, 38.87500000273120548, -35.31076352940723240 ) ) ;
#21049=CARTESIAN_POINT ( 'NONE',  ( 32.50000000000000711, 56.90000000000001279, 10.55989012756945122 ) ) ;
#21053=VERTEX_POINT ( 'NONE', #25398 ) ;
#21054=CARTESIAN_POINT ( 'NONE',  ( 33.58253175000000113, 74.37500000273118417, -4.112674001490185761E-15 ) ) ;
#21059=CARTESIAN_POINT ( 'NONE',  ( -20.75514604977248112, 43.42500000273117422, 28.56700777964554661 ) ) ;
#21063=CARTESIAN_POINT ( 'NONE',  ( 32.50000000000000000, 3.600000005462375086, -10.55989012756945833 ) ) ;
#21083=CARTESIAN_POINT ( 'NONE',  ( 27.16883889988624290, 58.17500000273119554, 19.73931689729373673 ) ) ;
#21091=CARTESIAN_POINT ( 'NONE',  ( 32.50000000000000000, 71.10000000000000853, -10.55989012756945833 ) ) ;
#21092=CARTESIAN_POINT ( 'NONE',  ( 10.37757302488624056, 16.52500000273120051, -31.93888565452638417 ) ) ;
#21096=CARTESIAN_POINT ( 'NONE',  ( -32.50000000000000000, 38.50000000546237544, 0.000000000000000000 ) ) ;
#21101=CARTESIAN_POINT ( 'NONE',  ( 33.58253175000000823, 62.02500000273116143, 10.91162601494192863 ) ) ;
#21105=CARTESIAN_POINT ( 'NONE',  ( -20.75514604977248823, 4.825000002731186122, -28.56700777964554305 ) ) ;
#21115=CARTESIAN_POINT ( 'NONE',  ( 10.04305231718579705, 20.59999999999999432, 30.90933677959248982 ) ) ;
#21119=CARTESIAN_POINT ( 'NONE',  ( -32.46390416700894122, 67.00000000000000000, -8.309214287527556309 ) ) ;
#21127=CARTESIAN_POINT ( 'NONE',  ( -20.75514604977248823, 32.82500000273118701, -28.56700777964554305 ) ) ;
#21130=EDGE_CURVE ( 'NONE', #15118, #13792, #2218, .T. ) ;
#21133=CARTESIAN_POINT ( 'NONE',  ( 20.08610463437157279, 51.80000000546238681, -27.64615127144129758 ) ) ;
#21141=CARTESIAN_POINT ( 'NONE',  ( 10.37757302488624056, 26.77500000273118275, -31.93888565452638417 ) ) ;
#21145=CARTESIAN_POINT ( 'NONE',  ( -26.29305231718579350, 14.30000000546237438, -19.10302069950537884 ) ) ;
#21155=CARTESIAN_POINT ( 'NONE',  ( 27.16883889988623935, 60.32500000273120833, -19.73931689729374384 ) ) ;
#21166=CARTESIAN_POINT ( 'NONE',  ( -10.37757302488623701, 75.77500000273117564, 31.93888565452638417 ) ) ;
#21171=CARTESIAN_POINT ( 'NONE',  ( 20.75514604977248467, 56.42500000273120264, -28.56700777964554305 ) ) ;
#21172=CARTESIAN_POINT ( 'NONE',  ( -33.58253175000000113, 19.37500000273119483, 0.000000000000000000 ) ) ;
#21173=CARTESIAN_POINT ( 'NONE',  ( -20.75514604977248823, 3.075000002731183901, -28.56700777964554305 ) ) ;
#21177=CARTESIAN_POINT ( 'NONE',  ( -20.08610463437156923, 70.80000000546235128, 27.64615127144130113 ) ) ;
#21178=CARTESIAN_POINT ( 'NONE',  ( 31.04172217648528687, 52.00000000000000711, 12.81397374188273908 ) ) ;
#21184=CARTESIAN_POINT ( 'NONE',  ( 10.37757302488624056, 48.77500000273120406, -31.93888565452638417 ) ) ;
#21188=ORIENTED_EDGE ( 'NONE', *, *, #19956, .T. ) ;
#21189=CARTESIAN_POINT ( 'NONE',  ( 10.37757302488624767, 25.72500000273118914, 31.93888565452638417 ) ) ;
#21192=CARTESIAN_POINT ( 'NONE',  ( 2.205017735002230837E-13, 57.49999999999998579, -32.50000000000000000 ) ) ;
#21202=CARTESIAN_POINT ( 'NONE',  ( -10.04305231718578462, 60.39999999999999858, 30.90933677959249337 ) ) ;
#21203=CARTESIAN_POINT ( 'NONE',  ( -26.29305231718579350, 19.79999999999999716, -19.10302069950537884 ) ) ;
#21209=CARTESIAN_POINT ( 'NONE',  ( 10.37757302488624056, 72.52500000273118985, -31.93888565452638417 ) ) ;
#21210=CARTESIAN_POINT ( 'NONE',  ( 10.37757302488624767, 35.97500000273119980, 31.93888565452638417 ) ) ;
#21217=CARTESIAN_POINT ( 'NONE',  ( -26.29305231718578995, 56.20000000000001705, 19.10302069950538595 ) ) ;
#21224=CARTESIAN_POINT ( 'NONE',  ( 10.37757302488624056, 72.77500000273118985, -31.93888565452638417 ) ) ;
#21229=CARTESIAN_POINT ( 'NONE',  ( -27.16883889988623935, 43.32500000273119412, 19.73931689729374739 ) ) ;
#21233=CARTESIAN_POINT ( 'NONE',  ( -11.66012699757880355, 66.98735890369596291, -31.52215860731681119 ) ) ;
#21234=CARTESIAN_POINT ( 'NONE',  ( 10.04305231718579705, 7.100000005462389296, 30.90933677959248982 ) ) ;
#21253=CARTESIAN_POINT ( 'NONE',  ( -33.58253175000000113, 55.37500000273119838, 0.000000000000000000 ) ) ;
#21257=CARTESIAN_POINT ( 'NONE',  ( -1.778240108872766143E-15, 55.49999999999999289, -32.49999999999999289 ) ) ;
#21259=CARTESIAN_POINT ( 'NONE',  ( -26.29305231718579350, 73.80000000000001137, -19.10302069950537884 ) ) ;
#21260=CARTESIAN_POINT ( 'NONE',  ( 33.58253175000000113, 16.22500000273118914, -10.91162601494193751 ) ) ;
#21265=CARTESIAN_POINT ( 'NONE',  ( 32.50000000000000000, 35.50000000546236834, -3.980102097228898626E-15 ) ) ;
#21270=EDGE_LOOP ( 'NONE', ( #27873, #26577, #24583, #28086 ) ) ;
#21271=CARTESIAN_POINT ( 'NONE',  ( 10.37757302488624767, 65.72500000273119269, 31.93888565452638417 ) ) ;
#21275=CARTESIAN_POINT ( 'NONE',  ( 27.16883889988624290, 5.925000002731190207, 19.73931689729373673 ) ) ;
#21287=CARTESIAN_POINT ( 'NONE',  ( 32.50000000000000000, 23.00000000000000711, -3.980102097228898626E-15 ) ) ;
#21291=CARTESIAN_POINT ( 'NONE',  ( -21.77128556259171788, 66.99999999999998579, 24.67464075869981244 ) ) ;
#21300=CARTESIAN_POINT ( 'NONE',  ( 27.16883889988623935, 36.32500000273118701, -19.73931689729374384 ) ) ;
#21305=CARTESIAN_POINT ( 'NONE',  ( -2.092463501923844636E-15, 54.00000000546236834, -34.17252228774368916 ) ) ;
#21310=CARTESIAN_POINT ( 'NONE',  ( 20.75514604977249178, 26.07500000273119767, 28.56700777964553950 ) ) ;
#21314=CARTESIAN_POINT ( 'NONE',  ( -20.08610463437157989, 14.20000000546237295, -27.64615127144129758 ) ) ;
#21318=( BOUNDED_CURVE ( )  B_SPLINE_CURVE ( 2, ( #9731, #27585, #4413, #4586, #27756, #17295, #14890 ),
 .UNSPECIFIED., .F., .T. ) 
 B_SPLINE_CURVE_WITH_KNOTS ( ( 3, 2, 2, 3 ),
 ( 0.1666666666666667962, 0.1692307692307693234, 0.1717948717948718229, 0.1730769230769230727 ),
 .UNSPECIFIED. ) 
 CURVE ( )  GEOMETRIC_REPRESENTATION_ITEM ( )  RATIONAL_B_SPLINE_CURVE ( ( 0.9999999999999974465, 0.9510565162951561957, 1.000000000000000000, 0.9510565162951535312, 1.000000000000000000, 0.9755282581475768211, 0.9755282581475768211 ) ) 
 REPRESENTATION_ITEM ( '' )  );
#21323=CARTESIAN_POINT ( 'NONE',  ( 10.37757302488624056, 52.52500000273117564, -31.93888565452638417 ) ) ;
#21328=DIRECTION ( 'NONE',  ( 0.000000000000000000, 1.000000000000000000, 0.000000000000000000 ) ) ;
#21333=CARTESIAN_POINT ( 'NONE',  ( 10.37757302488624056, 66.77500000273118985, -31.93888565452638417 ) ) ;
#21337=CARTESIAN_POINT ( 'NONE',  ( 20.75514604977249178, 53.82500000273119412, 28.56700777964553950 ) ) ;
#21338=CARTESIAN_POINT ( 'NONE',  ( 10.37757302488624056, 16.77500000273117564, -31.93888565452638417 ) ) ;
#21339=CARTESIAN_POINT ( 'NONE',  ( -10.37757302488624411, 78.72500000273117848, -31.93888565452638417 ) ) ;
#21343=CARTESIAN_POINT ( 'NONE',  ( -20.08610463437156923, 76.80000000546239391, 27.64615127144130113 ) ) ;
#21345=CARTESIAN_POINT ( 'NONE',  ( 29.06502868860493294, 52.00000000000000000, -15.87274502311855251 ) ) ;
#21351=CARTESIAN_POINT ( 'NONE',  ( 20.75514604977248467, 48.67500000273117422, -28.56700777964554305 ) ) ;
#21356=CARTESIAN_POINT ( 'NONE',  ( -27.16883889988624290, 18.92500000273118843, -19.73931689729374028 ) ) ;
#21370=CARTESIAN_POINT ( 'NONE',  ( -32.50000000000000000, 11.99999999999999645, 0.000000000000000000 ) ) ;
#21376=CARTESIAN_POINT ( 'NONE',  ( -2.162160676586881955E-15, 74.62500000273116996, -35.31076352940723240 ) ) ;
#21377=CARTESIAN_POINT ( 'NONE',  ( 27.16883889988624290, 38.17500000273120264, 19.73931689729373673 ) ) ;
#21382=CARTESIAN_POINT ( 'NONE',  ( 10.04305231718578817, 55.39999999999999147, -30.90933677959249337 ) ) ;
#21387=CARTESIAN_POINT ( 'NONE',  ( -10.37757302488624411, 64.97500000273119269, -31.93888565452638417 ) ) ;
#21392=CARTESIAN_POINT ( 'NONE',  ( 27.16883889988624290, 39.92500000273118133, 19.73931689729373673 ) ) ;
#21396=CARTESIAN_POINT ( 'NONE',  ( -10.04305231718578462, 60.90000000546237402, 30.90933677959249337 ) ) ;
#21402=EDGE_CURVE ( 'NONE', #29266, #927, #14087, .T. ) ;
#21409=EDGE_CURVE ( 'NONE', #10580, #6717, #31222, .T. ) ;
#21417=CARTESIAN_POINT ( 'NONE',  ( 10.37757302488624767, 57.97500000273118559, 31.93888565452638417 ) ) ;
#21419=( BOUNDED_CURVE ( )  B_SPLINE_CURVE ( 2, ( #16180, #2623, #18919, #13086, #29365, #5865, #13428, #23896, #26799, #23560, #24, #5702, #10513 ),
 .UNSPECIFIED., .F., .F. ) 
 B_SPLINE_CURVE_WITH_KNOTS ( ( 3, 2, 2, 2, 2, 2, 3 ),
 ( 0.1474358975042141251, 0.1487179487179487170, 0.1512820512820512719, 0.1538461538461538547, 0.1564102564102564097, 0.1589743589743589647, 0.1602564102564102699 ),
 .UNSPECIFIED. ) 
 CURVE ( )  GEOMETRIC_REPRESENTATION_ITEM ( )  RATIONAL_B_SPLINE_CURVE ( ( 0.9755282581475768211, 0.9755282594516028194, 1.000000000000000000, 0.9510565162951535312, 1.000000000000000000, 0.9510565162951535312, 1.000000000000000000, 0.9510565162951535312, 1.000000000000000000, 0.9510565162951535312, 1.000000000000000000, 0.9755282581475764880, 0.9755282581475768211 ) ) 
 REPRESENTATION_ITEM ( '' )  );
#21425=CARTESIAN_POINT ( 'NONE',  ( 10.04305231718579705, 72.59999999999998010, 30.90933677959248982 ) ) ;
#21426=CARTESIAN_POINT ( 'NONE',  ( 20.75514604977248467, 8.425000002731186655, -28.56700777964554305 ) ) ;
#21433=CARTESIAN_POINT ( 'NONE',  ( 33.58253175000000113, 64.22500000273117848, -10.91162601494193751 ) ) ;
#21437=CARTESIAN_POINT ( 'NONE',  ( 33.58253175000000823, 4.025000002731196957, 10.91162601494192863 ) ) ;
#21438=ORIENTED_EDGE ( 'NONE', *, *, #25716, .T. ) ;
#21447=CARTESIAN_POINT ( 'NONE',  ( -26.29305231718579350, 23.80000000000000071, -19.10302069950537884 ) ) ;
#21459=CARTESIAN_POINT ( 'NONE',  ( -7.689115195225046939, 52.00000000000003553, 32.34176759466017614 ) ) ;
#21460=CARTESIAN_POINT ( 'NONE',  ( 10.37757302488624056, 28.52500000273118630, -31.93888565452638417 ) ) ;
#21462=CARTESIAN_POINT ( 'NONE',  ( 26.29305231718578995, 65.20000000000001705, -19.10302069950538240 ) ) ;
#21467=CARTESIAN_POINT ( 'NONE',  ( -32.50000000000000000, 54.60000000546237686, 10.55989012756946366 ) ) ;
#21475=CARTESIAN_POINT ( 'NONE',  ( 26.29305231718578995, 17.70000000546238894, -19.10302069950538240 ) ) ;
#21485=CARTESIAN_POINT ( 'NONE',  ( -10.37757302488624411, 54.72500000273118559, -31.93888565452638417 ) ) ;
#21490=CARTESIAN_POINT ( 'NONE',  ( 0.000000000000000000, 52.00000000000000711, 0.000000000000000000 ) ) ;
#21494=CARTESIAN_POINT ( 'NONE',  ( 27.16883889988624290, 66.17500000273116711, 19.73931689729373673 ) ) ;
#21498=CARTESIAN_POINT ( 'NONE',  ( -10.37757302488624411, 50.72500000273118559, -31.93888565452638417 ) ) ;
#21499=CARTESIAN_POINT ( 'NONE',  ( 10.37757302488624056, 12.77500000273117031, -31.93888565452638417 ) ) ;
#21500=CARTESIAN_POINT ( 'NONE',  ( 27.16883889988623935, 64.57500000273118701, -19.73931689729374384 ) ) ;
#21504=CARTESIAN_POINT ( 'NONE',  ( -10.04305231718579172, 74.10000000546239107, -30.90933677959248982 ) ) ;
#21511=CARTESIAN_POINT ( 'NONE',  ( 33.58253175000000113, 50.37500000273119127, -4.112674001490185761E-15 ) ) ;
#21517=CARTESIAN_POINT ( 'NONE',  ( -20.75514604977248823, 18.82500000273119767, -28.56700777964554305 ) ) ;
#21532=CARTESIAN_POINT ( 'NONE',  ( 32.50000000000000711, 8.900000000000011013, 10.55989012756945122 ) ) ;
#21538=CARTESIAN_POINT ( 'NONE',  ( 33.58253175000000823, 74.02500000273120406, 10.91162601494192863 ) ) ;
#21539=CARTESIAN_POINT ( 'NONE',  ( -20.75514604977248823, 31.07500000273118701, -28.56700777964554305 ) ) ;
#21547=VECTOR ( 'NONE', #33470, 1000.000000000000000 ) ;
#21548=CARTESIAN_POINT ( 'NONE',  ( 6.277390505771533514E-15, 54.49999999999999289, 34.17252228774368916 ) ) ;
#21555=ORIENTED_EDGE ( 'NONE', *, *, #13790, .F. ) ;
#21556=CARTESIAN_POINT ( 'NONE',  ( -2.162160676586881955E-15, 64.87500000273119838, -35.31076352940723240 ) ) ;
#21560=CARTESIAN_POINT ( 'NONE',  ( -27.16883889988623935, 39.32500000273118701, 19.73931689729374739 ) ) ;
#21564=CARTESIAN_POINT ( 'NONE',  ( -20.08610463437157989, 60.20000000546237828, -27.64615127144129758 ) ) ;
#21576=VECTOR ( 'NONE', #22801, 999.9999999999998863 ) ;
#21578=CARTESIAN_POINT ( 'NONE',  ( -20.08610463437157989, 54.20000000546236407, -27.64615127144129758 ) ) ;
#21582=CARTESIAN_POINT ( 'NONE',  ( -27.16883889988624290, 49.17500000273118843, -19.73931689729374028 ) ) ;
#21588=CARTESIAN_POINT ( 'NONE',  ( -2.092463501923844636E-15, 71.50000000000001421, -34.17252228774368916 ) ) ;
#21589=CARTESIAN_POINT ( 'NONE',  ( -10.37757302488623701, 11.52500000273119696, 31.93888565452638417 ) ) ;
#21596=VECTOR ( 'NONE', #20055, 1000.000000000000000 ) ;
#21598=AXIS2_PLACEMENT_3D ( 'NONE', #27855, #30583, #1749 ) ;
#21600=CARTESIAN_POINT ( 'NONE',  ( -10.37757302488623701, 57.52500000273118275, 31.93888565452638417 ) ) ;
#21614=CARTESIAN_POINT ( 'NONE',  ( 10.04305231718579705, 22.59999999999999432, 30.90933677959248982 ) ) ;
#21625=PLANE ( 'NONE',  #10240 ) ;
#21627=CARTESIAN_POINT ( 'NONE',  ( 33.58253175000000113, 28.22500000273119269, -10.91162601494193751 ) ) ;
#21628=CARTESIAN_POINT ( 'NONE',  ( 32.50000000000000711, 64.89999999999999147, 10.55989012756945122 ) ) ;
#21632=CARTESIAN_POINT ( 'NONE',  ( -20.08610463437157989, 50.20000000546237118, -27.64615127144129758 ) ) ;
#21638=CARTESIAN_POINT ( 'NONE',  ( -27.16883889988623935, 73.32500000273118701, 19.73931689729374739 ) ) ;
#21643=CARTESIAN_POINT ( 'NONE',  ( -32.50000000000000000, 18.60000000546238041, 10.55989012756946366 ) ) ;
#21660=CARTESIAN_POINT ( 'NONE',  ( -33.58253175000000113, 71.27500000273118985, -10.91162601494193218 ) ) ;
#21661=ORIENTED_EDGE ( 'NONE', *, *, #10556, .F. ) ;
#21666=CARTESIAN_POINT ( 'NONE',  ( 10.37757302488624767, 47.72500000273117848, 31.93888565452638417 ) ) ;
#21667=CARTESIAN_POINT ( 'NONE',  ( 33.58253175000000823, 12.27500000273118452, 10.91162601494192863 ) ) ;
#21668=CARTESIAN_POINT ( 'NONE',  ( -27.16883889988624290, 65.17500000273116711, -19.73931689729374028 ) ) ;
#21672=CARTESIAN_POINT ( 'NONE',  ( -26.29305231718579350, 70.30000000546236549, -19.10302069950537884 ) ) ;
#21681=CARTESIAN_POINT ( 'NONE',  ( 10.37757302488624767, 45.97500000273117848, 31.93888565452638417 ) ) ;
#21685=VERTEX_POINT ( 'NONE', #27929 ) ;
#21686=CARTESIAN_POINT ( 'NONE',  ( -33.58253175000000113, 17.12500000273119127, 0.000000000000000000 ) ) ;
#21696=EDGE_CURVE ( 'NONE', #21685, #2770, #21318, .T. ) ;
#21699=CARTESIAN_POINT ( 'NONE',  ( -32.50000000000000000, 64.10000000000000853, 10.55989012756946366 ) ) ;
#21703=CARTESIAN_POINT ( 'NONE',  ( -26.29305231718578995, 8.199999999999999289, 19.10302069950538595 ) ) ;
#21709=CARTESIAN_POINT ( 'NONE',  ( -33.58253175000000113, 69.02500000273118985, -10.91162601494193218 ) ) ;
#21710=CARTESIAN_POINT ( 'NONE',  ( -10.37757302488624411, 26.97500000273118914, -31.93888565452638417 ) ) ;
#21711=CARTESIAN_POINT ( 'NONE',  ( 27.16883889988623935, 14.57500000273119412, -19.73931689729374384 ) ) ;
#21719=CARTESIAN_POINT ( 'NONE',  ( 20.08610463437157279, 55.29999999999999716, -27.64615127144129758 ) ) ;
#21724=CARTESIAN_POINT ( 'NONE',  ( 10.37757302488624767, 67.97500000273119269, 31.93888565452638417 ) ) ;
#21730=CARTESIAN_POINT ( 'NONE',  ( -2.162160676586881955E-15, 38.62500000273118417, -35.31076352940723240 ) ) ;
#21731=DIRECTION ( 'NONE',  ( 0.000000000000000000, 0.000000000000000000, 1.000000000000000000 ) ) ;
#21734=CARTESIAN_POINT ( 'NONE',  ( 33.58253175000000113, 66.37500000273121259, -4.112674001490185761E-15 ) ) ;
#21735=CARTESIAN_POINT ( 'NONE',  ( 20.08610463437158344, 58.70000000000000995, 27.64615127144129403 ) ) ;
#21748=CARTESIAN_POINT ( 'NONE',  ( -32.50000000000000000, 54.50000000546238965, 0.000000000000000000 ) ) ;
#21752=CARTESIAN_POINT ( 'NONE',  ( -33.58253175000000113, 47.27500000273116143, -10.91162601494193218 ) ) ;
#21754=EDGE_CURVE ( 'NONE', #17565, #1221, #20515, .T. ) ;
#21758=( BOUNDED_CURVE ( )  B_SPLINE_CURVE ( 2, ( #17212, #19953, #4498, #33143, #33497, #32800, #30400, #1404, #19614, #9649, #30060, #9472, #1570, #6900, #3990, #14463, #24919, #27670, #25092, #12047, #17381, #27845, #4329, #25267, #1740, #12220, #18412, #20655, #26461, #33848, #5356, #31095, #10172, #7592, #13081, #31263, #7758, #18244, #20473, #28691, #18069, #5188, #26121, #23891, #10507, #2618, #20819, #15672, #18583, #17903, #28518, #23555, #7927, #28859, #19, #20985, #5013, #31435, #15495, #15836, #26293, #2782, #28356, #13248, #23386, #23721, #188, #10675, #21155, #31597, #7417, #4842, #8096, #10343, #33674, #2953, #29023, #25950, #15324, #13423, #5526, #16006, #10000, #2444, #30924, #25780, #2268, #12741, #23214, #12911, #11801, #24061, #3912, #22279, #30320, #32722, #528, #6651, #17132, #27588, #14381, #1148, #13596, #4077, #27759, #9057, #10847, #24674, #9218, #31932, #24840, #14552, #19537, #19866, #6817, #19702, #14218, #26630, #11630, #11015, #22114, #26795, #17298, #1318, #21485, #25011, #27421, #8425, #29985, #30147, #5697, #1493, #11967, #18914, #4247, #32558, #22438, #29360, #5861, #16339, #32885, #3288, #9384, #6490, #14721, #362, #21323, #16963, #31764, #8257, #18749, #29191, #16174 ),
 .UNSPECIFIED., .F., .F. ) 
 B_SPLINE_CURVE_WITH_KNOTS ( ( 3, 2, 2, 2, 2, 2, 2, 2, 2, 2, 2, 2, 2, 2, 2, 2, 2, 2, 2, 2, 2, 2, 2, 2, 2, 2, 2, 2, 2, 2, 2, 2, 2, 2, 2, 2, 2, 2, 2, 2, 2, 2, 2, 2, 2, 2, 2, 2, 2, 2, 2, 2, 2, 2, 2, 2, 2, 2, 2, 2, 2, 2, 2, 2, 2, 2, 2, 2, 2, 2, 2, 2, 2, 2, 2, 2, 3 ),
 ( 0.1554413423931151617, 0.1564102564102564097, 0.1589743589743589647, 0.1615384615384615474, 0.1641025641025641024, 0.1666666666666666574, 0.1692307692307692402, 0.1717948717948717952, 0.1743589743589743501, 0.1769230769230769329, 0.1794871794871794879, 0.1820512820512820429, 0.1846153846153846256, 0.1871794871794871806, 0.1897435897435897356, 0.1923076923076923184, 0.1948717948717948734, 0.1974358974358974284, 0.2000000000000000111, 0.2025641025641025661, 0.2051282051282051211, 0.2076923076923077038, 0.2102564102564102588, 0.2128205128205128138, 0.2153846153846153966, 0.2179487179487179516, 0.2205128205128205066, 0.2230769230769230893, 0.2256410256410256443, 0.2282051282051281993, 0.2307692307692307820, 0.2333333333333333370, 0.2358974358974358920, 0.2384615384615384470, 0.2410256410256410298, 0.2435897435897435848, 0.2461538461538461675, 0.2487179487179487225, 0.2512820512820512775, 0.2538461538461538325, 0.2564102564102563875, 0.2589743589743589980, 0.2615384615384615530, 0.2641025641025641080, 0.2666666666666666630, 0.2692307692307692180, 0.2717948717948717730, 0.2743589743589743835, 0.2769230769230769384, 0.2794871794871794934, 0.2820512820512820484, 0.2846153846153846034, 0.2871794871794871584, 0.2897435897435897689, 0.2923076923076923239, 0.2948717948717948789, 0.2974358974358974339, 0.2999999999999999889, 0.3025641025641025439, 0.3051282051282051544, 0.3076923076923077094, 0.3102564102564102644, 0.3128205128205128194, 0.3153846153846153744, 0.3179487179487179294, 0.3205128205128205399, 0.3230769230769230949, 0.3256410256410256499, 0.3282051282051281493, 0.3307692307692307598, 0.3333333333333333148, 0.3358974358974358698, 0.3384615384615384803, 0.3410256410256410353, 0.3435897435897435903, 0.3461538461538461453, 0.3477490347008075355 ),
 .UNSPECIFIED. ) 
 CURVE ( )  GEOMETRIC_REPRESENTATION_ITEM ( )  RATIONAL_B_SPLINE_CURVE ( ( 0.9769881597858880440, 0.9815054093103534605, 1.000000000000000000, 0.9510565162951535312, 1.000000000000000000, 0.9510565162951535312, 1.000000000000000000, 0.9510565162951535312, 1.000000000000000000, 0.9510565162951535312, 1.000000000000000000, 0.9510565162951535312, 1.000000000000000000, 0.9510565162951535312, 1.000000000000000000, 0.9510565162951535312, 1.000000000000000000, 0.9510565162951535312, 1.000000000000000000, 0.9510565162951535312, 1.000000000000000000, 0.9510565162951535312, 1.000000000000000000, 0.9510565162951535312, 1.000000000000000000, 0.9510565162951535312, 1.000000000000000000, 0.9510565162951535312, 1.000000000000000000, 0.9510565162951535312, 1.000000000000000000, 0.9510565162951535312, 1.000000000000000000, 0.9510565162951535312, 1.000000000000000000, 0.9510565162951535312, 1.000000000000000000, 0.9510565162951535312, 1.000000000000000000, 0.9510565162951535312, 1.000000000000000000, 0.9510565162951535312, 1.000000000000000000, 0.9510565162951535312, 1.000000000000000000, 0.9510565162951535312, 1.000000000000000000, 0.9510565162951535312, 1.000000000000000000, 0.9510565162951535312, 1.000000000000000000, 0.9510565162951535312, 1.000000000000000000, 0.9510565162951535312, 1.000000000000000000, 0.9510565162951535312, 1.000000000000000000, 0.9510565162951535312, 1.000000000000000000, 0.9510565162951535312, 1.000000000000000000, 0.9510565162951535312, 1.000000000000000000, 0.9510565162951535312, 1.000000000000000000, 0.9510565162951535312, 1.000000000000000000, 0.9510565162951535312, 1.000000000000000000, 0.9510565162951535312, 1.000000000000000000, 0.9510565162951535312, 1.000000000000000000, 0.9510565162951535312, 1.000000000000000000, 0.9510565162951535312, 1.000000000000000000, 0.9510565162951535312, 1.000000000000000000, 0.9510565162951535312, 1.000000000000000000, 0.9510565162951535312, 1.000000000000000000, 0.9510565162951535312, 1.000000000000000000, 0.9510565162951535312, 1.000000000000000000, 0.9510565162951535312, 1.000000000000000000, 0.9510565162951535312, 1.000000000000000000, 0.9510565162951535312, 1.000000000000000000, 0.9510565162951535312, 1.000000000000000000, 0.9510565162951535312, 1.000000000000000000, 0.9510565162951535312, 1.000000000000000000, 0.9510565162951535312, 1.000000000000000000, 0.9510565162951535312, 1.000000000000000000, 0.9510565162951535312, 1.000000000000000000, 0.9510565162951535312, 1.000000000000000000, 0.9510565162951535312, 1.000000000000000000, 0.9510565162951535312, 1.000000000000000000, 0.9510565162951535312, 1.000000000000000000, 0.9510565162951535312, 1.000000000000000000, 0.9510565162951535312, 1.000000000000000000, 0.9510565162951535312, 1.000000000000000000, 0.9510565162951535312, 1.000000000000000000, 0.9510565162951535312, 1.000000000000000000, 0.9510565162951535312, 1.000000000000000000, 0.9510565162951535312, 1.000000000000000000, 0.9510565162951535312, 1.000000000000000000, 0.9510565162951535312, 1.000000000000000000, 0.9510565162951535312, 1.000000000000000000, 0.9510565162951535312, 1.000000000000000000, 0.9510565162951535312, 1.000000000000000000, 0.9510565162951535312, 1.000000000000000000, 0.9510565162951535312, 1.000000000000000000, 0.9510565162951535312, 1.000000000000000000, 0.9510565162951535312, 1.000000000000000000, 0.9510565162951535312, 1.000000000000000000, 0.9510565162951535312, 1.000000000000000000, 0.9510565162951535312, 1.000000000000000000, 0.9695511069847985164, 0.9769881597858887101 ) ) 
 REPRESENTATION_ITEM ( '' )  );
#21760=CARTESIAN_POINT ( 'NONE',  ( -32.50000000000000000, 72.09999999999999432, 10.55989012756946366 ) ) ;
#21761=CARTESIAN_POINT ( 'NONE',  ( 20.75514604977248467, 10.42500000273120087, -28.56700777964554305 ) ) ;
#21771=CARTESIAN_POINT ( 'NONE',  ( 27.16883889988624290, 55.92500000273119554, 19.73931689729373673 ) ) ;
#21783=CARTESIAN_POINT ( 'NONE',  ( 32.50000000000000711, 22.90000000000000568, 10.55989012756945122 ) ) ;
#21793=CARTESIAN_POINT ( 'NONE',  ( -10.28315354913682711, 52.00000000000000000, 31.56665548893541029 ) ) ;
#21794=CARTESIAN_POINT ( 'NONE',  ( -10.37757302488624411, 26.72500000273118914, -31.93888565452638417 ) ) ;
#21795=CARTESIAN_POINT ( 'NONE',  ( 20.08610463437157279, 61.80000000546237970, -27.64615127144129758 ) ) ;
#21798=CARTESIAN_POINT ( 'NONE',  ( -26.29305231718579350, 50.30000000546237970, -19.10302069950537884 ) ) ;
#21800=CARTESIAN_POINT ( 'NONE',  ( -32.50000000000000000, 58.60000000546236265, 10.55989012756946366 ) ) ;
#21803=CARTESIAN_POINT ( 'NONE',  ( -27.16883889988624290, 72.92500000273120975, -19.73931689729374028 ) ) ;
#21806=ORIENTED_EDGE ( 'NONE', *, *, #13556, .F. ) ;
#21808=CARTESIAN_POINT ( 'NONE',  ( 10.04305231718579705, 13.10000000546239463, 30.90933677959248982 ) ) ;
#21818=DIRECTION ( 'NONE',  ( 1.000000000000000000, 0.000000000000000000, 0.000000000000000000 ) ) ;
#21827=ADVANCED_FACE ( 'NONE', ( #7841 ), #31181, .F. ) ;
#21828=CARTESIAN_POINT ( 'NONE',  ( -27.16883889988624290, 67.17500000273118133, -19.73931689729374028 ) ) ;
#21834=CARTESIAN_POINT ( 'NONE',  ( -27.16883889988623935, 49.32500000273120122, 19.73931689729374739 ) ) ;
#21835=CARTESIAN_POINT ( 'NONE',  ( -20.75514604977248112, 13.67500000273118133, 28.56700777964554661 ) ) ;
#21836=CARTESIAN_POINT ( 'NONE',  ( -10.37757302488624411, 62.97500000273119269, -31.93888565452638417 ) ) ;
#21840=CARTESIAN_POINT ( 'NONE',  ( 32.50000000000000000, 69.50000000546239676, -3.980102097228898626E-15 ) ) ;
#21845=ORIENTED_EDGE ( 'NONE', *, *, #15985, .T. ) ;
#21846=CARTESIAN_POINT ( 'NONE',  ( 33.58253175000000823, 50.27500000273118985, 10.91162601494192863 ) ) ;
#21851=CARTESIAN_POINT ( 'NONE',  ( -27.16883889988624290, 16.92500000273118488, -19.73931689729374028 ) ) ;
#21865=CARTESIAN_POINT ( 'NONE',  ( -10.04305231718579172, 11.59999999999998543, -30.90933677959248982 ) ) ;
#21871=CARTESIAN_POINT ( 'NONE',  ( 10.37757302488624056, 68.52500000273118985, -31.93888565452638417 ) ) ;
#21872=CARTESIAN_POINT ( 'NONE',  ( -33.58253175000000113, 29.27500000273118630, -10.91162601494193218 ) ) ;
#21873=CARTESIAN_POINT ( 'NONE',  ( -27.16883889988624290, 19.17500000273118843, -19.73931689729374028 ) ) ;
#21879=CARTESIAN_POINT ( 'NONE',  ( 10.04305231718579705, 46.60000000000001563, 30.90933677959248982 ) ) ;
#21884=CARTESIAN_POINT ( 'NONE',  ( -27.16883889988623935, 67.57500000273118701, 19.73931689729374739 ) ) ;
#21889=CARTESIAN_POINT ( 'NONE',  ( 27.16883889988623935, 36.32500000273118701, -19.73931689729374384 ) ) ;
#21911=CARTESIAN_POINT ( 'NONE',  ( 6.486482029760649416E-15, 47.87500000273117706, 35.31076352940723240 ) ) ;
#21915=DIRECTION ( 'NONE',  ( 0.000000000000000000, 1.000000000000000000, 0.000000000000000000 ) ) ;
#21917=CARTESIAN_POINT ( 'NONE',  ( 32.50000000000000000, 65.10000000000000853, -10.55989012756945833 ) ) ;
#21918=CARTESIAN_POINT ( 'NONE',  ( -20.75514604977248823, 8.825000002731190563, -28.56700777964554305 ) ) ;
#21927=CARTESIAN_POINT ( 'NONE',  ( 10.37757302488624767, 53.72500000273118559, 31.93888565452638417 ) ) ;
#21928=CARTESIAN_POINT ( 'NONE',  ( 6.486482029760649416E-15, 27.87500000273120193, 35.31076352940723240 ) ) ;
#21932=CARTESIAN_POINT ( 'NONE',  ( -10.37757302488623701, 1.525000002731188964, 31.93888565452638417 ) ) ;
#21955=CARTESIAN_POINT ( 'NONE',  ( 32.50000000000000000, 66.99999999999998579, -3.980102097228898626E-15 ) ) ;
#21958=CARTESIAN_POINT ( 'NONE',  ( -20.75514604977248112, 27.42500000273118488, 28.56700777964554661 ) ) ;
#21959=CARTESIAN_POINT ( 'NONE',  ( 5.147494310547434893, 56.55125428154684641, 32.49999999999999289 ) ) ;
#21963=CARTESIAN_POINT ( 'NONE',  ( -10.04305231718578462, 46.90000000546238823, 30.90933677959249337 ) ) ;
#21965=CARTESIAN_POINT ( 'NONE',  ( 40.00000000000000000, 66.99999999999998579, 23.09401076758503990 ) ) ;
#21968=CARTESIAN_POINT ( 'NONE',  ( -2.162160676586881955E-15, 72.62500000273118417, -35.31076352940723240 ) ) ;
#21970=CARTESIAN_POINT ( 'NONE',  ( 40.00000000000000000, 52.00000000000000711, 23.09401076758503990 ) ) ;
#21973=CARTESIAN_POINT ( 'NONE',  ( -20.08610463437156923, 12.80000000546237615, 27.64615127144130113 ) ) ;
#21983=CARTESIAN_POINT ( 'NONE',  ( 32.50000000000000711, 38.89999999999999147, 10.55989012756945122 ) ) ;
#21991=CARTESIAN_POINT ( 'NONE',  ( 6.486482029760649416E-15, 65.87500000273119838, 35.31076352940723240 ) ) ;
#21996=CARTESIAN_POINT ( 'NONE',  ( 33.58253175000000113, 48.12500000273119127, -4.112674001490185761E-15 ) ) ;
#21997=CARTESIAN_POINT ( 'NONE',  ( 10.37757302488624767, 11.97500000273120335, 31.93888565452638417 ) ) ;
#21998=CARTESIAN_POINT ( 'NONE',  ( 33.58253175000000823, 60.27500000273116143, 10.91162601494192685 ) ) ;
#22002=CARTESIAN_POINT ( 'NONE',  ( -26.29305231718578995, 68.70000000546237118, 19.10302069950538595 ) ) ;
#22003=AXIS2_PLACEMENT_3D ( 'NONE', #16336, #13752, #24222 ) ;
#22010=CARTESIAN_POINT ( 'NONE',  ( 20.75514604977248467, 42.67500000273119554, -28.56700777964554305 ) ) ;
#22013=CARTESIAN_POINT ( 'NONE',  ( -20.08610463437157989, 28.20000000546236762, -27.64615127144129758 ) ) ;
#22015=CARTESIAN_POINT ( 'NONE',  ( 10.37757302488624056, 20.52500000273117919, -31.93888565452638417 ) ) ;
#22032=CARTESIAN_POINT ( 'NONE',  ( -26.29305231718578995, 10.20000000000000107, 19.10302069950538595 ) ) ;
#22038=CARTESIAN_POINT ( 'NONE',  ( 27.16883889988623935, 68.32500000273118701, -19.73931689729374384 ) ) ;
#22039=CARTESIAN_POINT ( 'NONE',  ( -33.58253175000000113, 31.47500000273117493, 10.91162601494193929 ) ) ;
#22040=CARTESIAN_POINT ( 'NONE',  ( -2.162160676586881955E-15, 14.87500000273120193, -35.31076352940723240 ) ) ;
#22046=CARTESIAN_POINT ( 'NONE',  ( 6.277390505771533514E-15, 50.50000000000000000, 34.17252228774368916 ) ) ;
#22052=CARTESIAN_POINT ( 'NONE',  ( 10.37757302488624767, 63.97500000273119269, 31.93888565452638417 ) ) ;
#22058=CARTESIAN_POINT ( 'NONE',  ( -10.37757302488624411, 36.72500000273119980, -31.93888565452638417 ) ) ;
#22080=CARTESIAN_POINT ( 'NONE',  ( -33.58253175000000113, 49.47500000273118559, 10.91162601494193929 ) ) ;
#22087=CARTESIAN_POINT ( 'NONE',  ( 10.04305231718578817, 67.40000000000000568, -30.90933677959249337 ) ) ;
#22088=CARTESIAN_POINT ( 'NONE',  ( 33.58253175000000823, 6.025000002731191628, 10.91162601494192863 ) ) ;
#22098=CARTESIAN_POINT ( 'NONE',  ( 33.58253175000000113, 58.22500000273116427, -10.91162601494193751 ) ) ;
#22099=CARTESIAN_POINT ( 'NONE',  ( 33.58253175000000113, 30.47500000273117493, -10.91162601494193751 ) ) ;
#22114=CARTESIAN_POINT ( 'NONE',  ( -33.58253175000000113, 55.12500000273119838, 0.000000000000000000 ) ) ;
#22119=EDGE_CURVE ( 'NONE', #15118, #13108, #12649, .T. ) ;
#22129=CARTESIAN_POINT ( 'NONE',  ( 6.486482029760649416E-15, 25.62500000273118772, 35.31076352940723240 ) ) ;
#22135=CARTESIAN_POINT ( 'NONE',  ( -10.04305231718578462, 50.90000000546239534, 30.90933677959249337 ) ) ;
#22138=CARTESIAN_POINT ( 'NONE',  ( 27.16883889988623935, 78.32500000273120122, -19.73931689729374384 ) ) ;
#22140=FACE_OUTER_BOUND ( 'NONE', #14434, .T. ) ;
#22143=CARTESIAN_POINT ( 'NONE',  ( 20.08610463437158344, 13.20000000546237651, 27.64615127144129403 ) ) ;
#22155=CARTESIAN_POINT ( 'NONE',  ( 32.50000000000000711, 34.89999999999999858, 10.55989012756945122 ) ) ;
#22168=CARTESIAN_POINT ( 'NONE',  ( -27.16883889988623935, 47.32500000273119412, 19.73931689729374739 ) ) ;
#22169=CARTESIAN_POINT ( 'NONE',  ( -33.58253175000000113, 7.375000002731183280, 0.000000000000000000 ) ) ;
#22170=CARTESIAN_POINT ( 'NONE',  ( 20.75514604977249178, 60.07500000273120122, 28.56700777964553950 ) ) ;
#22174=CARTESIAN_POINT ( 'NONE',  ( -10.04305231718578462, 68.90000000546238823, 30.90933677959249337 ) ) ;
#22177=CARTESIAN_POINT ( 'NONE',  ( 5.779280353836490358E-15, 54.49999999999999289, 32.49999999999999289 ) ) ;
#22178=CARTESIAN_POINT ( 'NONE',  ( 1.093617666956751375E-13, 66.00000000546238255, -32.50000000000000711 ) ) ;
#22180=CARTESIAN_POINT ( 'NONE',  ( 10.37757302488624056, 42.77500000273119696, -31.93888565452638417 ) ) ;
#22182=CARTESIAN_POINT ( 'NONE',  ( -26.29305231718578995, 32.70000000546237118, 19.10302069950538595 ) ) ;
#22191=CYLINDRICAL_SURFACE ( 'NONE', #17417, 32.50000000000000000 ) ;
#22198=CARTESIAN_POINT ( 'NONE',  ( -32.50000000000000000, 56.00000000000000711, 0.000000000000000000 ) ) ;
#22200=CARTESIAN_POINT ( 'NONE',  ( -32.50000000000000000, 5.999999999999991118, 0.000000000000000000 ) ) ;
#22205=CARTESIAN_POINT ( 'NONE',  ( 20.75514604977249178, 63.82500000273119412, 28.56700777964553950 ) ) ;
#22206=CARTESIAN_POINT ( 'NONE',  ( 10.37757302488624056, 28.77500000273118630, -31.93888565452638417 ) ) ;
#22207=CARTESIAN_POINT ( 'NONE',  ( -10.37757302488623701, 13.77500000273117209, 31.93888565452638417 ) ) ;
#22213=CARTESIAN_POINT ( 'NONE',  ( 32.50000000000000000, 49.09999999999999432, -10.55989012756945833 ) ) ;
#22218=CARTESIAN_POINT ( 'NONE',  ( 33.58253175000000823, 58.27500000273116854, 10.91162601494192863 ) ) ;
#22223=CARTESIAN_POINT ( 'NONE',  ( -20.75514604977248823, 30.82500000273119767, -28.56700777964554305 ) ) ;
#22225=ORIENTED_EDGE ( 'NONE', *, *, #18697, .T. ) ;
#22240=CARTESIAN_POINT ( 'NONE',  ( 32.50000000000000000, 53.50000000546238965, -3.980102097228898626E-15 ) ) ;
#22247=CARTESIAN_POINT ( 'NONE',  ( 20.75514604977249178, 48.07500000273120122, 28.56700777964553950 ) ) ;
#22254=CARTESIAN_POINT ( 'NONE',  ( -10.04305231718578462, 64.40000000000000568, 30.90933677959249337 ) ) ;
#22264=CARTESIAN_POINT ( 'NONE',  ( -10.37757302488623701, 53.52500000273118275, 31.93888565452638417 ) ) ;
#22265=CARTESIAN_POINT ( 'NONE',  ( -2.162160676586881955E-15, 28.87500000273119838, -35.31076352940723240 ) ) ;
#22269=CARTESIAN_POINT ( 'NONE',  ( -33.58253175000000113, 1.125000002731191273, 0.000000000000000000 ) ) ;
#22279=CARTESIAN_POINT ( 'NONE',  ( 20.75514604977249178, 57.82500000273119412, 28.56700777964553950 ) ) ;
#22294=CARTESIAN_POINT ( 'NONE',  ( -10.37757302488623701, 19.52500000273120406, 31.93888565452638417 ) ) ;
#22299=CARTESIAN_POINT ( 'NONE',  ( -20.08610463437156923, 48.80000000546235128, 27.64615127144130113 ) ) ;
#22303=CARTESIAN_POINT ( 'NONE',  ( -27.16883889988624290, 76.92500000273120975, -19.73931689729374028 ) ) ;
#22306=FACE_OUTER_BOUND ( 'NONE', #5431, .T. ) ;
#22309=CARTESIAN_POINT ( 'NONE',  ( 32.50000000000000711, 13.40000000546237047, 10.55989012756945122 ) ) ;
#22320=CARTESIAN_POINT ( 'NONE',  ( 10.04305231718578817, 33.39999999999999858, -30.90933677959249337 ) ) ;
#22332=CARTESIAN_POINT ( 'NONE',  ( -27.16883889988624290, 46.92500000273118133, -19.73931689729374028 ) ) ;
#22333=CARTESIAN_POINT ( 'NONE',  ( -33.58253175000000113, 7.275000002731196957, -10.91162601494193218 ) ) ;
#22334=CARTESIAN_POINT ( 'NONE',  ( 33.58253175000000823, 54.27500000273118985, 10.91162601494192685 ) ) ;
#22338=CARTESIAN_POINT ( 'NONE',  ( -2.092463501923844636E-15, 66.00000000546239676, -34.17252228774368916 ) ) ;
#22343=CARTESIAN_POINT ( 'NONE',  ( 10.37757302488624056, 40.77500000273119696, -31.93888565452638417 ) ) ;
#22345=CARTESIAN_POINT ( 'NONE',  ( -26.29305231718578995, 30.70000000546237118, 19.10302069950538595 ) ) ;
#22363=CARTESIAN_POINT ( 'NONE',  ( -20.75514604977248823, 79.07500000273121543, -28.56700777964554305 ) ) ;
#22369=CARTESIAN_POINT ( 'NONE',  ( 20.75514604977248467, 66.42500000273120975, -28.56700777964554305 ) ) ;
#22370=CARTESIAN_POINT ( 'NONE',  ( -20.75514604977248112, 21.67500000273119554, 28.56700777964554661 ) ) ;
#22371=CARTESIAN_POINT ( 'NONE',  ( 10.37757302488624767, 15.97500000273120691, 31.93888565452638417 ) ) ;
#22376=CARTESIAN_POINT ( 'NONE',  ( -26.29305231718578995, 46.20000000000000284, 19.10302069950538595 ) ) ;
#22381=CARTESIAN_POINT ( 'NONE',  ( -2.162160676586881955E-15, 60.87500000273116996, -35.31076352940723240 ) ) ;
#22386=CARTESIAN_POINT ( 'NONE',  ( -33.58253175000000113, 33.02500000273118275, -10.91162601494193218 ) ) ;
#22407=CARTESIAN_POINT ( 'NONE',  ( 33.58253175000000823, 44.27500000273120406, 10.91162601494192863 ) ) ;
#22412=CARTESIAN_POINT ( 'NONE',  ( 20.08610463437158344, 68.70000000000001705, 27.64615127144129403 ) ) ;
#22421=CARTESIAN_POINT ( 'NONE',  ( -20.75514604977248823, 46.82500000273117990, -28.56700777964554305 ) ) ;
#22422=CARTESIAN_POINT ( 'NONE',  ( -2.162160676586881955E-15, 24.87500000273117351, -35.31076352940723240 ) ) ;
#22438=CARTESIAN_POINT ( 'NONE',  ( -10.37757302488623701, 53.52500000273118275, 31.93888565452638417 ) ) ;
#22450=CARTESIAN_POINT ( 'NONE',  ( -1.778240108872766143E-15, 64.00000000546238255, -32.49999999999999289 ) ) ;
#22452=CARTESIAN_POINT ( 'NONE',  ( -33.58253175000000113, 25.02500000273117209, -10.91162601494193218 ) ) ;
#22456=CARTESIAN_POINT ( 'NONE',  ( -26.29305231718579350, 44.30000000546237260, -19.10302069950537884 ) ) ;
#22461=CARTESIAN_POINT ( 'NONE',  ( -20.75514604977248112, 71.42500000273119554, 28.56700777964554661 ) ) ;
#22468=CARTESIAN_POINT ( 'NONE',  ( 10.04305231718579705, 57.10000000546237686, 30.90933677959248982 ) ) ;
#22469=CARTESIAN_POINT ( 'NONE',  ( 26.29305231718578995, 9.700000005462380059, -19.10302069950538240 ) ) ;
#22479=CARTESIAN_POINT ( 'NONE',  ( -32.50000000000000000, 37.89999999999999858, -10.55989012756945478 ) ) ;
#22491=CARTESIAN_POINT ( 'NONE',  ( 20.75514604977249178, 41.82500000273119412, 28.56700777964553950 ) ) ;
#22492=CARTESIAN_POINT ( 'NONE',  ( 20.75514604977249178, 4.075000002731181681, 28.56700777964553950 ) ) ;
#22493=CARTESIAN_POINT ( 'NONE',  ( 10.37757302488624056, 54.77500000273121117, -31.93888565452638417 ) ) ;
#22497=CARTESIAN_POINT ( 'NONE',  ( 10.04305231718579705, 63.10000000546238397, 30.90933677959248982 ) ) ;
#22499=( BOUNDED_CURVE ( )  B_SPLINE_CURVE ( 2, ( #66, #10552, #31483, #18459, #12615, #31645, #906, #31812, #3497, #29068, #32146, #26838, #10723 ),
 .UNSPECIFIED., .F., .T. ) 
 B_SPLINE_CURVE_WITH_KNOTS ( ( 3, 2, 2, 2, 2, 2, 3 ),
 ( 0.1602564102564102699, 0.1615384615384615474, 0.1641025641025641024, 0.1666666666666666574, 0.1692307692307692402, 0.1717948717948717952, 0.1730769230769230727 ),
 .UNSPECIFIED. ) 
 CURVE ( )  GEOMETRIC_REPRESENTATION_ITEM ( )  RATIONAL_B_SPLINE_CURVE ( ( 0.9755282581475768211, 0.9755282581475770431, 1.000000000000000000, 0.9510565162951535312, 1.000000000000000000, 0.9510565162951535312, 1.000000000000000000, 0.9510565162951535312, 1.000000000000000000, 0.9510565162951535312, 1.000000000000000000, 0.9755282581475768211, 0.9755282581475768211 ) ) 
 REPRESENTATION_ITEM ( '' )  );
#22501=CARTESIAN_POINT ( 'NONE',  ( -5.147494310547430452, 53.55125428154685352, -32.49999999999999289 ) ) ;
#22503=CARTESIAN_POINT ( 'NONE',  ( -33.58253175000000113, 39.47500000273117848, 10.91162601494193929 ) ) ;
#22505=VERTEX_POINT ( 'NONE', #30230 ) ;
#22506=CARTESIAN_POINT ( 'NONE',  ( -20.08610463437156923, 28.80000000546238326, 27.64615127144130113 ) ) ;
#22507=ORIENTED_EDGE ( 'NONE', *, *, #23495, .T. ) ;
#22512=VECTOR ( 'NONE', #18202, 1000.000000000000114 ) ;
#22527=CARTESIAN_POINT ( 'NONE',  ( -32.50000000000000000, 2.100000000000006306, 10.55989012756946366 ) ) ;
#22533=CARTESIAN_POINT ( 'NONE',  ( 20.75514604977249178, 61.82500000273116569, 28.56700777964553950 ) ) ;
#22534=CARTESIAN_POINT ( 'NONE',  ( 33.58253175000000113, 24.47500000273118914, -10.91162601494193751 ) ) ;
#22535=CARTESIAN_POINT ( 'NONE',  ( 10.37757302488624767, 7.975000002731199800, 31.93888565452638417 ) ) ;
#22540=CARTESIAN_POINT ( 'NONE',  ( 32.50000000000000711, 44.90000000000001279, 10.55989012756945122 ) ) ;
#22545=CARTESIAN_POINT ( 'NONE',  ( 6.486482029760649416E-15, 61.87500000273117706, 35.31076352940723240 ) ) ;
#22549=CARTESIAN_POINT ( 'NONE',  ( 20.75514604977248467, 32.42500000273116711, -28.56700777964554305 ) ) ;
#22574=CARTESIAN_POINT ( 'NONE',  ( 33.58253175000000113, 40.37500000273118417, -4.112674001490185761E-15 ) ) ;
#22580=CARTESIAN_POINT ( 'NONE',  ( 6.277390505771533514E-15, 66.49999999999998579, 34.17252228774368916 ) ) ;
#22590=CARTESIAN_POINT ( 'NONE',  ( -10.37757302488623701, 51.52500000273117564, 31.93888565452638417 ) ) ;
#22591=CARTESIAN_POINT ( 'NONE',  ( 10.37757302488624767, 19.97500000273118204, 31.93888565452638417 ) ) ;
#22596=DIRECTION ( 'NONE',  ( 0.000000000000000000, 1.000000000000000000, 0.000000000000000000 ) ) ;
#22609=AXIS2_PLACEMENT_3D ( 'NONE', #18106, #21023, #26162 ) ;
#22610=CARTESIAN_POINT ( 'NONE',  ( 40.00000000000000000, 66.99999999999998579, 23.09401076758503990 ) ) ;
#22615=CARTESIAN_POINT ( 'NONE',  ( -27.16883889988623935, 59.57500000273117990, 19.73931689729374739 ) ) ;
#22624=CARTESIAN_POINT ( 'NONE',  ( 27.16883889988623935, 22.32500000273117280, -19.73931689729374384 ) ) ;
#22626=CARTESIAN_POINT ( 'NONE',  ( 2.205017735002230837E-13, 56.00000000546238255, -32.50000000000000000 ) ) ;
#22629=CARTESIAN_POINT ( 'NONE',  ( 26.29305231718579350, 43.30000000546237260, 19.10302069950537529 ) ) ;
#22637=CARTESIAN_POINT ( 'NONE',  ( -2.162160676586881955E-15, 68.62500000273119838, -35.31076352940723240 ) ) ;
#22643=CARTESIAN_POINT ( 'NONE',  ( 27.16883889988624290, 11.92500000273118133, 19.73931689729373673 ) ) ;
#22651=CARTESIAN_POINT ( 'NONE',  ( 20.08610463437158344, 38.70000000000000284, 27.64615127144129403 ) ) ;
#22666=CARTESIAN_POINT ( 'NONE',  ( -33.58253175000000113, 41.02500000273118985, -10.91162601494193218 ) ) ;
#22667=CARTESIAN_POINT ( 'NONE',  ( -27.16883889988623935, 7.575000002731188786, 19.73931689729374739 ) ) ;
#22668=CARTESIAN_POINT ( 'NONE',  ( 10.37757302488624056, 52.77500000273120406, -31.93888565452638417 ) ) ;
#22672=CARTESIAN_POINT ( 'NONE',  ( -2.092463501923844636E-15, 60.00000000546238255, -34.17252228774368916 ) ) ;
#22678=CARTESIAN_POINT ( 'NONE',  ( 20.75514604977249178, 42.07500000273117990, 28.56700777964553950 ) ) ;
#22683=CARTESIAN_POINT ( 'NONE',  ( -26.29305231718578995, 28.70000000546237118, 19.10302069950538595 ) ) ;
#22688=VERTEX_POINT ( 'NONE', #33677 ) ;
#22702=CARTESIAN_POINT ( 'NONE',  ( 26.72982461517084474, 52.00000000000001421, 20.44820386143251767 ) ) ;
#22703=( BOUNDED_CURVE ( )  B_SPLINE_CURVE ( 2, ( #32335, #19312, #16076, #5425, #15905, #2850, #29428, #32000, #8496, #3025, #5931, #13321, #31668 ),
 .UNSPECIFIED., .F., .T. ) 
 B_SPLINE_CURVE_WITH_KNOTS ( ( 3, 2, 2, 2, 2, 2, 3 ),
 ( 0.2243589743589743668, 0.2256410256410256443, 0.2282051282051281993, 0.2307692307692307820, 0.2333333333333333370, 0.2358974358974358920, 0.2371794871794871973 ),
 .UNSPECIFIED. ) 
 CURVE ( )  GEOMETRIC_REPRESENTATION_ITEM ( )  RATIONAL_B_SPLINE_CURVE ( ( 0.9755282581475768211, 0.9755282581475768211, 1.000000000000000000, 0.9510565162951535312, 1.000000000000000000, 0.9510565162951535312, 1.000000000000000000, 0.9510565162951535312, 1.000000000000000000, 0.9510565162951535312, 1.000000000000000000, 0.9755282581475764880, 0.9755282581475768211 ) ) 
 REPRESENTATION_ITEM ( '' )  );
#22704=CARTESIAN_POINT ( 'NONE',  ( 27.16883889988623935, 78.57500000273120122, -19.73931689729374384 ) ) ;
#22710=( BOUNDED_CURVE ( )  B_SPLINE_CURVE ( 2, ( #14851, #27721, #12616, #27893, #33373, #28402, #28061, #7117, #22917, #2141, #25142, #20528, #25317 ),
 .UNSPECIFIED., .F., .F. ) 
 B_SPLINE_CURVE_WITH_KNOTS ( ( 3, 2, 2, 2, 2, 2, 3 ),
 ( 0.3141025641025640969, 0.3153846153846153744, 0.3179487179487179294, 0.3205128205128205399, 0.3230769230769230949, 0.3256410256410256499, 0.3269230769230769273 ),
 .UNSPECIFIED. ) 
 CURVE ( )  GEOMETRIC_REPRESENTATION_ITEM ( )  RATIONAL_B_SPLINE_CURVE ( ( 0.9755282581475768211, 0.9755282581475768211, 1.000000000000000000, 0.9510565162951535312, 1.000000000000000000, 0.9510565162951535312, 1.000000000000000000, 0.9510565162951535312, 1.000000000000000000, 0.9510565162951535312, 1.000000000000000000, 0.9755282581475768211, 0.9755282581475768211 ) ) 
 REPRESENTATION_ITEM ( '' )  );
#22711=CARTESIAN_POINT ( 'NONE',  ( 33.58253175000000823, 58.02500000273117564, 10.91162601494192863 ) ) ;
#22712=CARTESIAN_POINT ( 'NONE',  ( -33.58253175000000113, 25.27500000273119696, -10.91162601494193218 ) ) ;
#22713=CARTESIAN_POINT ( 'NONE',  ( -27.16883889988623935, 9.575000002731190563, 19.73931689729374739 ) ) ;
#22719=CARTESIAN_POINT ( 'NONE',  ( -20.75514604977248112, 1.425000002731191984, 28.56700777964554661 ) ) ;
#22721=CARTESIAN_POINT ( 'NONE',  ( -10.04305231718578462, 40.40000000000000568, 30.90933677959249337 ) ) ;
#22726=CARTESIAN_POINT ( 'NONE',  ( 20.75514604977249178, 62.07500000273118701, 28.56700777964553950 ) ) ;
#22731=CARTESIAN_POINT ( 'NONE',  ( -27.16883889988623935, 33.32500000273118701, 19.73931689729374739 ) ) ;
#22749=CARTESIAN_POINT ( 'NONE',  ( 10.37757302488624056, 78.52500000273120406, -31.93888565452638417 ) ) ;
#22750=CARTESIAN_POINT ( 'NONE',  ( 10.37757302488624056, 42.77500000273119696, -31.93888565452638417 ) ) ;
#22756=CARTESIAN_POINT ( 'NONE',  ( 32.50000000000000000, 62.99999999999998579, -3.980102097228898626E-15 ) ) ;
#22766=CARTESIAN_POINT ( 'NONE',  ( -33.58253175000000113, 49.02500000273116854, -10.91162601494193218 ) ) ;
#22767=CARTESIAN_POINT ( 'NONE',  ( -33.58253175000000113, 23.27500000273116854, -10.91162601494193218 ) ) ;
#22771=DIRECTION ( 'NONE',  ( 0.000000000000000000, 1.000000000000000000, 0.000000000000000000 ) ) ;
#22791=CARTESIAN_POINT ( 'NONE',  ( -20.75514604977248112, 59.67500000273118133, 28.56700777964554661 ) ) ;
#22799=CARTESIAN_POINT ( 'NONE',  ( -20.75514604977248823, 24.82500000273117635, -28.56700777964554305 ) ) ;
#22801=DIRECTION ( 'NONE',  ( 0.8660254037844387076, 0.000000000000000000, 0.5000000000000001110 ) ) ;
#22804=CARTESIAN_POINT ( 'NONE',  ( 26.29305231718579350, 39.30000000546239391, 19.10302069950537529 ) ) ;
#22805=( BOUNDED_CURVE ( )  B_SPLINE_CURVE ( 2, ( #17433, #25663, #27894, #14852, #25318, #2142, #12617 ),
 .UNSPECIFIED., .F., .T. ) 
 B_SPLINE_CURVE_WITH_KNOTS ( ( 3, 2, 2, 3 ),
 ( 0.3525641025641025883, 0.3538461538461538658, 0.3564102564102563653, 0.3589743589743589203 ),
 .UNSPECIFIED. ) 
 CURVE ( )  GEOMETRIC_REPRESENTATION_ITEM ( )  RATIONAL_B_SPLINE_CURVE ( ( 0.9755282581475768211, 0.9755282581475772652, 1.000000000000000000, 0.9510565162951535312, 1.000000000000000000, 0.9510565162951546414, 0.9999999999999988898 ) ) 
 REPRESENTATION_ITEM ( '' )  );
#22809=CARTESIAN_POINT ( 'NONE',  ( -10.37757302488623701, 71.52500000273118985, 31.93888565452638417 ) ) ;
#22815=CARTESIAN_POINT ( 'NONE',  ( -20.75514604977248823, 10.82500000273118701, -28.56700777964554305 ) ) ;
#22824=CARTESIAN_POINT ( 'NONE',  ( 10.04305231718578817, 29.39999999999999503, -30.90933677959249337 ) ) ;
#22837=CARTESIAN_POINT ( 'NONE',  ( 33.58253175000000113, 44.22500000273117138, -10.91162601494193751 ) ) ;
#22838=CARTESIAN_POINT ( 'NONE',  ( -20.75514604977248112, 7.675000002731199089, 28.56700777964554661 ) ) ;
#22839=CARTESIAN_POINT ( 'NONE',  ( -10.37757302488623701, 55.77500000273121117, 31.93888565452638417 ) ) ;
#22845=CARTESIAN_POINT ( 'NONE',  ( -32.50000000000000000, 62.50000000546239676, 0.000000000000000000 ) ) ;
#22852=CARTESIAN_POINT ( 'NONE',  ( -2.162160676586881955E-15, 34.87500000273117706, -35.31076352940723240 ) ) ;
#22856=CARTESIAN_POINT ( 'NONE',  ( -26.29305231718578995, 24.70000000546239249, 19.10302069950538595 ) ) ;
#22874=CARTESIAN_POINT ( 'NONE',  ( -20.08610463437157989, 55.69999999999998863, -27.64615127144129758 ) ) ;
#22877=CARTESIAN_POINT ( 'NONE',  ( -10.04305231718579172, 3.599999999999992095, -30.90933677959248982 ) ) ;
#22882=CARTESIAN_POINT ( 'NONE',  ( 10.37757302488624056, 60.52500000273118275, -31.93888565452638417 ) ) ;
#22883=CARTESIAN_POINT ( 'NONE',  ( -20.75514604977248823, 21.07500000273118346, -28.56700777964554305 ) ) ;
#22884=CARTESIAN_POINT ( 'NONE',  ( -33.58253175000000113, 13.27500000273118097, -10.91162601494193218 ) ) ;
#22889=CARTESIAN_POINT ( 'NONE',  ( 27.16883889988623935, 4.325000002731186122, -19.73931689729374384 ) ) ;
#22891=CARTESIAN_POINT ( 'NONE',  ( -32.50000000000000000, 41.99999999999999289, 0.000000000000000000 ) ) ;
#22896=CARTESIAN_POINT ( 'NONE',  ( -27.16883889988624290, 51.17500000273118843, -19.73931689729374028 ) ) ;
#22901=CARTESIAN_POINT ( 'NONE',  ( 27.16883889988623935, 32.32500000273117990, -19.73931689729374384 ) ) ;
#22917=CARTESIAN_POINT ( 'NONE',  ( 26.29305231718579350, 54.80000000000000426, 19.10302069950537529 ) ) ;
#22924=CARTESIAN_POINT ( 'NONE',  ( 33.58253175000000823, 42.27500000273118275, 10.91162601494192863 ) ) ;
#22929=CARTESIAN_POINT ( 'NONE',  ( 10.04305231718578817, 59.39999999999999147, -30.90933677959249337 ) ) ;
#22934=CARTESIAN_POINT ( 'NONE',  ( -20.75514604977248823, 79.07500000273121543, -28.56700777964554305 ) ) ;
#22939=CARTESIAN_POINT ( 'NONE',  ( -2.162160676586881955E-15, 48.62500000273118417, -35.31076352940723240 ) ) ;
#22940=CARTESIAN_POINT ( 'NONE',  ( -33.58253175000000113, 21.47500000273119980, 10.91162601494193929 ) ) ;
#22952=CARTESIAN_POINT ( 'NONE',  ( -14.93337011119329993, 67.00000000000000000, -30.15969763299878892 ) ) ;
#22963=CARTESIAN_POINT ( 'NONE',  ( -33.58253175000000113, 63.47500000273117138, 10.91162601494193929 ) ) ;
#22968=CARTESIAN_POINT ( 'NONE',  ( 5.147494310547380714, 63.05125428700923607, 32.50000000000002132 ) ) ;
#22970=CARTESIAN_POINT ( 'NONE',  ( -33.58253175000000113, 23.22500000273117138, 10.91162601494193929 ) ) ;
#22975=CARTESIAN_POINT ( 'NONE',  ( -32.50000000000000000, 40.50000000546237544, 0.000000000000000000 ) ) ;
#22981=CARTESIAN_POINT ( 'NONE',  ( 33.58253175000000113, 72.12500000273118417, -4.112674001490185761E-15 ) ) ;
#22988=CARTESIAN_POINT ( 'NONE',  ( 33.58253175000000823, 10.02500000273118275, 10.91162601494192863 ) ) ;
#22999=CARTESIAN_POINT ( 'NONE',  ( 20.08610463437157279, 31.30000000000000071, -27.64615127144129758 ) ) ;
#23014=CARTESIAN_POINT ( 'NONE',  ( 33.58253175000000113, 44.12500000273119127, -4.112674001490185761E-15 ) ) ;
#23016=CARTESIAN_POINT ( 'NONE',  ( 6.486482029760648627E-15, 53.87500000273119127, 35.31076352940722529 ) ) ;
#23020=CARTESIAN_POINT ( 'NONE',  ( 10.04305231718578817, 59.90000000546237402, -30.90933677959249337 ) ) ;
#23027=CARTESIAN_POINT ( 'NONE',  ( 10.37757302488624767, 37.97500000273119980, 31.93888565452638417 ) ) ;
#23031=CARTESIAN_POINT ( 'NONE',  ( -32.50000000000000000, 22.40000000546237402, -10.55989012756945478 ) ) ;
#23048=CARTESIAN_POINT ( 'NONE',  ( 33.58253175000000823, 76.27500000273118985, 10.91162601494192863 ) ) ;
#23053=CARTESIAN_POINT ( 'NONE',  ( -33.58253175000000113, 61.12500000273117706, 0.000000000000000000 ) ) ;
#23054=CARTESIAN_POINT ( 'NONE',  ( 27.16883889988623935, 26.57500000273120477, -19.73931689729374384 ) ) ;
#23055=CARTESIAN_POINT ( 'NONE',  ( 10.37757302488624767, 9.975000002731201576, 31.93888565452638417 ) ) ;
#23059=CARTESIAN_POINT ( 'NONE',  ( -33.58253175000000113, 3.125000002731193049, 0.000000000000000000 ) ) ;
#23062=CARTESIAN_POINT ( 'NONE',  ( 32.50000000000000000, 39.10000000000002274, -10.55989012756945833 ) ) ;
#23067=CARTESIAN_POINT ( 'NONE',  ( 27.16883889988624290, 56.17500000273119554, 19.73931689729373673 ) ) ;
#23072=CARTESIAN_POINT ( 'NONE',  ( 33.58253175000000823, 26.02500000273120406, 10.91162601494192863 ) ) ;
#23074=EDGE_LOOP ( 'NONE', ( #31544, #15335, #23845, #7964, #20097, #23108, #20513, #15396, #12212, #5708, #10331, #11492, #20466, #23543, #18695, #20551, #16080, #23960 ) ) ;
#23089=CARTESIAN_POINT ( 'NONE',  ( 6.486482029760649416E-15, 77.62500000273121259, 35.31076352940723240 ) ) ;
#23091=CARTESIAN_POINT ( 'NONE',  ( 27.16883889988624290, 42.17500000273118133, 19.73931689729373673 ) ) ;
#23097=CARTESIAN_POINT ( 'NONE',  ( -26.29305231718578995, 62.20000000000001705, 19.10302069950538595 ) ) ;
#23102=CARTESIAN_POINT ( 'NONE',  ( 33.58253175000000113, 70.47500000273117848, -10.91162601494193751 ) ) ;
#23107=CARTESIAN_POINT ( 'NONE',  ( -33.58253175000000113, 47.22500000273117138, 10.91162601494193929 ) ) ;
#23108=ORIENTED_EDGE ( 'NONE', *, *, #13369, .T. ) ;
#23111=CARTESIAN_POINT ( 'NONE',  ( -20.08610463437156923, 2.800000005462385477, 27.64615127144130113 ) ) ;
#23130=CARTESIAN_POINT ( 'NONE',  ( -33.58253175000000113, 61.27500000273118985, -10.91162601494193218 ) ) ;
#23136=CARTESIAN_POINT ( 'NONE',  ( 20.08610463437158344, 78.70000000000000284, 27.64615127144129403 ) ) ;
#23137=CARTESIAN_POINT ( 'NONE',  ( 33.58253175000000113, 18.22500000273118559, -10.91162601494193751 ) ) ;
#23143=CARTESIAN_POINT ( 'NONE',  ( -10.04305231718579172, 40.10000000546236265, -30.90933677959248982 ) ) ;
#23144=CARTESIAN_POINT ( 'NONE',  ( 5.779280353836490358E-15, 66.49999999999998579, 32.49999999999999289 ) ) ;
#23149=CARTESIAN_POINT ( 'NONE',  ( -33.58253175000000113, 67.02500000273117564, -10.91162601494193218 ) ) ;
#23157=CARTESIAN_POINT ( 'NONE',  ( -33.58253175000000113, 9.125000002731184168, 0.000000000000000000 ) ) ;
#23167=CARTESIAN_POINT ( 'NONE',  ( -32.50000000000000000, 52.60000000546235555, 10.55989012756946366 ) ) ;
#23170=CARTESIAN_POINT ( 'NONE',  ( -26.29305231718579350, 31.80000000000000782, -19.10302069950537884 ) ) ;
#23174=CARTESIAN_POINT ( 'NONE',  ( 5.147494310547426899, 63.44874571845314648, -32.50000000000000000 ) ) ;
#23182=CARTESIAN_POINT ( 'NONE',  ( 4.374313548017275011, 67.00000000000000000, -33.03144926559789241 ) ) ;
#23184=CARTESIAN_POINT ( 'NONE',  ( 6.486482029760649416E-15, 43.62500000273116285, 35.31076352940723240 ) ) ;
#23189=CARTESIAN_POINT ( 'NONE',  ( -32.50000000000000000, 62.40000000546235981, -10.55989012756945478 ) ) ;
#23196=CARTESIAN_POINT ( 'NONE',  ( 33.58253175000000113, 34.47500000273119980, -10.91162601494193751 ) ) ;
#23200=CARTESIAN_POINT ( 'NONE',  ( -26.29305231718578995, 22.70000000546239249, 19.10302069950538595 ) ) ;
#23212=VECTOR ( 'NONE', #29748, 1000.000000000000227 ) ;
#23214=CARTESIAN_POINT ( 'NONE',  ( 27.16883889988623935, 58.32500000273120833, -19.73931689729374384 ) ) ;
#23225=CARTESIAN_POINT ( 'NONE',  ( 10.37757302488624767, 71.97500000273120691, 31.93888565452638417 ) ) ;
#23230=CARTESIAN_POINT ( 'NONE',  ( -20.75514604977248112, 57.42500000273118843, 28.56700777964554661 ) ) ;
#23231=CARTESIAN_POINT ( 'NONE',  ( -27.16883889988624290, 17.17500000273118488, -19.73931689729374028 ) ) ;
#23232=CARTESIAN_POINT ( 'NONE',  ( -20.75514604977248823, 9.075000002731183457, -28.56700777964554305 ) ) ;
#23237=CARTESIAN_POINT ( 'NONE',  ( 33.58253175000000113, 2.125000002731192161, -4.112674001490185761E-15 ) ) ;
#23239=CARTESIAN_POINT ( 'NONE',  ( 32.50000000000000000, 40.99999999999999289, -3.980102097228898626E-15 ) ) ;
#23244=ORIENTED_EDGE ( 'NONE', *, *, #23644, .T. ) ;
#23245=CARTESIAN_POINT ( 'NONE',  ( -27.16883889988623935, 51.57500000273117280, 19.73931689729374739 ) ) ;
#23250=CARTESIAN_POINT ( 'NONE',  ( 20.75514604977249178, 25.82500000273117280, 28.56700777964553950 ) ) ;
#23265=CARTESIAN_POINT ( 'NONE',  ( -2.092463501923844636E-15, 15.50000000000000533, -34.17252228774368916 ) ) ;
#23271=CARTESIAN_POINT ( 'NONE',  ( 33.58253175000000823, 34.27500000273116854, 10.91162601494192863 ) ) ;
#23276=CARTESIAN_POINT ( 'NONE',  ( 26.29305231718578995, 61.20000000000001705, -19.10302069950538240 ) ) ;
#23280=CARTESIAN_POINT ( 'NONE',  ( -33.58253175000000113, 71.27500000273118985, -10.91162601494193218 ) ) ;
#23285=CARTESIAN_POINT ( 'NONE',  ( -20.75514604977248112, 41.42500000273118133, 28.56700777964554661 ) ) ;
#23290=CARTESIAN_POINT ( 'NONE',  ( -32.50000000000000000, 2.600000005462363095, 10.55989012756946366 ) ) ;
#23304=ADVANCED_FACE ( 'NONE', ( #31692 ), #18676, .F. ) ;
#23312=CARTESIAN_POINT ( 'NONE',  ( 27.16883889988623935, 64.57500000273118701, -19.73931689729374384 ) ) ;
#23318=CARTESIAN_POINT ( 'NONE',  ( -32.50000000000000000, 79.90000000000001990, -10.55989012756945478 ) ) ;
#23319=CARTESIAN_POINT ( 'NONE',  ( -10.37757302488623701, 17.52500000273120406, 31.93888565452638417 ) ) ;
#23324=CARTESIAN_POINT ( 'NONE',  ( 32.50000000000000000, 33.50000000546236834, -3.980102097228898626E-15 ) ) ;
#23330=CARTESIAN_POINT ( 'NONE',  ( 33.58253175000000113, 64.12500000273118417, -4.112674001490185761E-15 ) ) ;
#23337=CARTESIAN_POINT ( 'NONE',  ( -20.75514604977248823, 8.825000002731190563, -28.56700777964554305 ) ) ;
#23346=CARTESIAN_POINT ( 'NONE',  ( -32.50000000000000000, 52.40000000546238823, -10.55989012756945300 ) ) ;
#23348=CARTESIAN_POINT ( 'NONE',  ( 10.04305231718579705, 30.60000000000000142, 30.90933677959248982 ) ) ;
#23352=CARTESIAN_POINT ( 'NONE',  ( -29.06502868860481215, 67.00000000000000000, 15.87274502311879232 ) ) ;
#23358=CARTESIAN_POINT ( 'NONE',  ( 5.714234795769584707, 66.99999999999998579, -32.80324308525973720 ) ) ;
#23359=CARTESIAN_POINT ( 'NONE',  ( 10.37757302488624767, 33.72500000273119269, 31.93888565452638417 ) ) ;
#23360=CARTESIAN_POINT ( 'NONE',  ( 40.00000000000000000, 52.00000000000000711, 23.09401076758503990 ) ) ;
#23364=CARTESIAN_POINT ( 'NONE',  ( -2.092463501923844636E-15, 56.00000000546236123, -34.17252228774368916 ) ) ;
#23371=CARTESIAN_POINT ( 'NONE',  ( 20.75514604977249178, 38.07500000273116569, 28.56700777964553950 ) ) ;
#23375=CARTESIAN_POINT ( 'NONE',  ( -10.04305231718578462, 20.90000000546236691, 30.90933677959249337 ) ) ;
#23386=CARTESIAN_POINT ( 'NONE',  ( -10.37757302488624411, 60.72500000273119269, -31.93888565452638417 ) ) ;
#23395=DIRECTION ( 'NONE',  ( 0.8660254037844387076, 0.000000000000000000, 0.5000000000000001110 ) ) ;
#23396=CARTESIAN_POINT ( 'NONE',  ( -20.75514604977248823, 75.07500000273118701, -28.56700777964554305 ) ) ;
#23402=CARTESIAN_POINT ( 'NONE',  ( -2.162160676586881955E-15, 56.62500000273116996, -35.31076352940723240 ) ) ;
#23403=CARTESIAN_POINT ( 'NONE',  ( 33.58253175000000113, 20.37500000273119483, -4.112674001490185761E-15 ) ) ;
#23404=CARTESIAN_POINT ( 'NONE',  ( -10.37757302488624411, 4.975000002731183812, -31.93888565452638417 ) ) ;
#23408=CARTESIAN_POINT ( 'NONE',  ( -20.08610463437157989, 78.20000000546235697, -27.64615127144129758 ) ) ;
#23409=CARTESIAN_POINT ( 'NONE',  ( 13.17636326499326671, 51.99999999999998579, -29.96527208688312527 ) ) ;
#23414=CARTESIAN_POINT ( 'NONE',  ( 20.75514604977249178, 54.07500000273118701, 28.56700777964553950 ) ) ;
#23418=CARTESIAN_POINT ( 'NONE',  ( -27.16883889988623935, 23.32500000273117635, 19.73931689729374739 ) ) ;
#23429=EDGE_CURVE ( 'NONE', #52, #32793, #25912, .T. ) ;
#23435=CARTESIAN_POINT ( 'NONE',  ( -20.08610463437157989, 19.69999999999998863, -27.64615127144129758 ) ) ;
#23442=CARTESIAN_POINT ( 'NONE',  ( -10.37757302488624411, 36.97500000273119980, -31.93888565452638417 ) ) ;
#23449=CARTESIAN_POINT ( 'NONE',  ( 20.08610463437158344, 60.70000000000000284, 27.64615127144129403 ) ) ;
#23453=CARTESIAN_POINT ( 'NONE',  ( -10.37757302488624411, 74.97500000273120691, -31.93888565452638417 ) ) ;
#23458=CARTESIAN_POINT ( 'NONE',  ( -20.75514604977248823, 42.82500000273119412, -28.56700777964554305 ) ) ;
#23462=CARTESIAN_POINT ( 'NONE',  ( -26.29305231718578995, 2.700000005462374730, 19.10302069950538595 ) ) ;
#23481=CARTESIAN_POINT ( 'NONE',  ( -33.58253175000000113, 53.27500000273117564, -10.91162601494193218 ) ) ;
#23485=VECTOR ( 'NONE', #31862, 1000.000000000000000 ) ;
#23487=CARTESIAN_POINT ( 'NONE',  ( -20.08610463437157989, 79.70000000000000284, -27.64615127144129758 ) ) ;
#23489=CARTESIAN_POINT ( 'NONE',  ( 10.37757302488624767, 17.72500000273118204, 31.93888565452638417 ) ) ;
#23494=CARTESIAN_POINT ( 'NONE',  ( 26.29305231718579350, 37.30000000546239391, 19.10302069950537529 ) ) ;
#23495=EDGE_CURVE ( 'NONE', #7658, #11742, #11430, .T. ) ;
#23501=CARTESIAN_POINT ( 'NONE',  ( 27.16883889988623935, 60.32500000273120833, -19.73931689729374384 ) ) ;
#23506=CARTESIAN_POINT ( 'NONE',  ( -33.58253175000000113, 3.225000002731179372, 10.91162601494193929 ) ) ;
#23514=CARTESIAN_POINT ( 'NONE',  ( -20.08610463437156923, 28.30000000000000782, 27.64615127144130113 ) ) ;
#23525=CARTESIAN_POINT ( 'NONE',  ( -3.724851327375141796, 66.99999999999997158, -33.24794091741932789 ) ) ;
#23527=CARTESIAN_POINT ( 'NONE',  ( -10.37757302488623701, 37.52500000273118985, 31.93888565452638417 ) ) ;
#23532=CARTESIAN_POINT ( 'NONE',  ( 32.50000000000000000, 55.50000000546238965, -3.980102097228898626E-15 ) ) ;
#23541=CARTESIAN_POINT ( 'NONE',  ( 20.75514604977248467, 34.67500000273118843, -28.56700777964554305 ) ) ;
#23543=ORIENTED_EDGE ( 'NONE', *, *, #13660, .T. ) ;
#23545=CARTESIAN_POINT ( 'NONE',  ( -10.04305231718579172, 26.10000000546238041, -30.90933677959248982 ) ) ;
#23555=CARTESIAN_POINT ( 'NONE',  ( 33.58253175000000823, 62.02500000273116854, 10.91162601494192685 ) ) ;
#23560=CARTESIAN_POINT ( 'NONE',  ( -20.08610463437157989, 66.20000000546238539, -27.64615127144129758 ) ) ;
#23565=CARTESIAN_POINT ( 'NONE',  ( 20.75514604977249178, 78.07500000273117280, 28.56700777964553950 ) ) ;
#23569=CARTESIAN_POINT ( 'NONE',  ( 33.58253175000000113, 56.12500000273119838, -4.112674001490185761E-15 ) ) ;
#23570=CARTESIAN_POINT ( 'NONE',  ( 33.58253175000000113, 14.47500000273118737, -10.91162601494193751 ) ) ;
#23571=CARTESIAN_POINT ( 'NONE',  ( 10.37757302488624767, 5.975000002731184701, 31.93888565452638417 ) ) ;
#23575=CARTESIAN_POINT ( 'NONE',  ( 32.50000000000000711, 71.40000000546241665, 10.55989012756945122 ) ) ;
#23583=CARTESIAN_POINT ( 'NONE',  ( -33.58253175000000113, 53.37500000273119838, 0.000000000000000000 ) ) ;
#23588=CARTESIAN_POINT ( 'NONE',  ( -2.162160676586881955E-15, 26.62500000273118417, -35.31076352940723240 ) ) ;
#23591=PLANE ( 'NONE',  #22609 ) ;
#23601=CARTESIAN_POINT ( 'NONE',  ( 6.277390505771533514E-15, 14.50000000000000888, 34.17252228774368916 ) ) ;
#23607=CARTESIAN_POINT ( 'NONE',  ( -27.16883889988623935, 75.32500000273118701, 19.73931689729374739 ) ) ;
#23608=CARTESIAN_POINT ( 'NONE',  ( -2.162160676586881955E-15, 34.87500000273117706, -35.31076352940723240 ) ) ;
#23614=CARTESIAN_POINT ( 'NONE',  ( -26.29305231718578995, 52.20000000000000995, 19.10302069950538595 ) ) ;
#23619=CARTESIAN_POINT ( 'NONE',  ( 20.75514604977249178, 72.07500000273120122, 28.56700777964553950 ) ) ;
#23626=CARTESIAN_POINT ( 'NONE',  ( 20.75514604977249178, 43.82500000273119412, 28.56700777964553950 ) ) ;
#23629=CARTESIAN_POINT ( 'NONE',  ( -26.29305231718578995, 60.70000000546237118, 19.10302069950538595 ) ) ;
#23630=CARTESIAN_POINT ( 'NONE',  ( -10.04305231718578462, 4.900000005462382013, 30.90933677959249337 ) ) ;
#23644=EDGE_CURVE ( 'NONE', #23797, #9681, #4174, .T. ) ;
#23651=CARTESIAN_POINT ( 'NONE',  ( 20.75514604977248467, 52.67500000273116711, -28.56700777964554305 ) ) ;
#23658=CARTESIAN_POINT ( 'NONE',  ( -2.092463501923844636E-15, 77.50000000000000000, -34.17252228774368916 ) ) ;
#23659=CARTESIAN_POINT ( 'NONE',  ( -33.58253175000000113, 17.12500000273119127, 0.000000000000000000 ) ) ;
#23663=CARTESIAN_POINT ( 'NONE',  ( 26.29305231718578995, 33.70000000546237118, -19.10302069950538240 ) ) ;
#23669=CARTESIAN_POINT ( 'NONE',  ( -2.162160676586881955E-15, 62.62500000273116996, -35.31076352940723240 ) ) ;
#23673=CARTESIAN_POINT ( 'NONE',  ( 33.58253175000000113, 4.225000002731190030, -10.91162601494193751 ) ) ;
#23681=CARTESIAN_POINT ( 'NONE',  ( 20.08610463437158344, 20.69999999999998508, 27.64615127144129403 ) ) ;
#23694=CARTESIAN_POINT ( 'NONE',  ( 6.486482029760649416E-15, 33.62500000273119127, 35.31076352940723240 ) ) ;
#23695=CYLINDRICAL_SURFACE ( 'NONE', #16068, 32.50000000000000000 ) ;
#23699=CARTESIAN_POINT ( 'NONE',  ( 26.29305231718579350, 55.30000000546237970, 19.10302069950537529 ) ) ;
#23706=CARTESIAN_POINT ( 'NONE',  ( 27.16883889988623935, 26.57500000273120477, -19.73931689729374384 ) ) ;
#23710=CARTESIAN_POINT ( 'NONE',  ( 32.50000000000000000, 15.50000000546238077, -3.980102097228898626E-15 ) ) ;
#23721=CARTESIAN_POINT ( 'NONE',  ( -2.162160676586882350E-15, 60.62500000273118417, -35.31076352940722529 ) ) ;
#23734=CARTESIAN_POINT ( 'NONE',  ( 27.16883889988624290, 74.17500000273118133, 19.73931689729373673 ) ) ;
#23738=CARTESIAN_POINT ( 'NONE',  ( -10.37757302488623701, 53.52500000273118275, 31.93888565452638417 ) ) ;
#23739=CARTESIAN_POINT ( 'NONE',  ( 33.58253175000000113, 18.47500000273117848, -10.91162601494193751 ) ) ;
#23740=CARTESIAN_POINT ( 'NONE',  ( -10.37757302488623701, 3.775000002731190740, 31.93888565452638417 ) ) ;
#23744=CARTESIAN_POINT ( 'NONE',  ( -10.04305231718578462, 70.90000000546238823, 30.90933677959249337 ) ) ;
#23745=CARTESIAN_POINT ( 'NONE',  ( 32.79451539931730508, 52.00000000000002842, -5.771861194046441490 ) ) ;
#23751=CARTESIAN_POINT ( 'NONE',  ( -10.37757302488624411, 46.97500000273117848, -31.93888565452638417 ) ) ;
#23756=CARTESIAN_POINT ( 'NONE',  ( -33.58253175000000113, 23.02500000273117919, -10.91162601494193218 ) ) ;
#23772=CARTESIAN_POINT ( 'NONE',  ( 10.04305231718578817, 19.40000000000001279, -30.90933677959249337 ) ) ;
#23780=CARTESIAN_POINT ( 'NONE',  ( 20.75514604977249178, 75.82500000273118701, 28.56700777964553950 ) ) ;
#23781=CARTESIAN_POINT ( 'NONE',  ( 20.75514604977249178, 36.07500000273117990, 28.56700777964553950 ) ) ;
#23787=CARTESIAN_POINT ( 'NONE',  ( 10.04305231718579705, 56.59999999999999432, 30.90933677959248982 ) ) ;
#23793=CARTESIAN_POINT ( 'NONE',  ( -2.162160676586881955E-15, 74.87500000273116996, -35.31076352940723240 ) ) ;
#23797=VERTEX_POINT ( 'NONE', #4002 ) ;
#23798=CARTESIAN_POINT ( 'NONE',  ( 33.58253175000000823, 44.02500000273118275, 10.91162601494192863 ) ) ;
#23803=CARTESIAN_POINT ( 'NONE',  ( -26.29305231718579350, 4.300000005462378816, -19.10302069950537884 ) ) ;
#23822=CARTESIAN_POINT ( 'NONE',  ( 10.37757302488624056, 58.77500000273121117, -31.93888565452638417 ) ) ;
#23829=( BOUNDED_SURFACE ( )  B_SPLINE_SURFACE ( 1, 2, ( 
 ( #9529, #25498, #12276, #27900, #7295, #7643, #22749, #1978, #12453, #4382, #25668, #18128, #2147, #28572, #12622, #23089, #33553, #10053, #33200, #20534, #5069, #30978, #17959, #26006, #9703, #25833, #2323, #2499, #20010, #29246, #247, #582, #31319, #23780, #26685, #31986, #8483, #18468, #23607, #23948, #16231, #15891, #13812, #7811, #18970, #21376, #13483, #29415, #13650, #24115, #5243, #21538, #5581, #10732, #13305, #33902, #8151, #18300, #29077, #5916, #3011, #21041, #31821, #8311, #16062, #28911, #21209, #5412, #26517, #31654, #18802, #18640, #2836, #15725, #5750, #26180, #2675, #417, #10393, #10562, #3181, #11072, #74, #16393, #3343, #10904, #26846, #20872, #28745, #13133, #7981, #31491, #26347, #29739, #6071, #11233, #24602, #1419, #16555, #915, #19295, #21709, #14146, #4004, #6243, #32815, #21871, #32321, #22038, #11394, #27008, #27351, #9308, #14311, #16888, #19793, #3505, #16724, #27179, #1244, #17226, #19629, #1076, #24934, #32155, #11556, #17055, #22369, #30241, #8812, #13975, #24766, #6580, #3672, #4176, #8648, #6746, #11722, #3836, #27686, #14477, #11897, #29570, #24280, #29914, #32482, #8983, #748, #19465, #6416, #9147, #27517, #30074, #22205, #19133, #24438, #32652, #17920, #1586, #14989, #25283, #28371, #20145, #19970, #1934, #25794, #12412, #12062, #30589, #4859, #33339, #12583, #4514, #22533, #33161, #32983, #31111, #20672, #2283, #6915, #23053, #30416, #7605, #10017, #9664, #25110, #22882, #9487, #17740, #33512, #1755, #20314, #20488, #9836, #15339, #30763, #17397, #27861, #28200, #4343, #14650, #7085, #14818, #7253, #4686, #18085, #25631, #12758, #15165, #12235, #2110, #22711, #17569, #30939, #28027, #7434, #25459, #23230, #33690, #10189, #28533, #2459, #31778, #2633, #31613, #23402, #13096, #21171, #31946, #2796, #23569, #7942, #15514, #8439, #10523, #18762, #8110, #29206, #20834, #377, #15687, #18930, #5540, #18259, #13263, #10863, #16021, #34, #15851, #25965, #29037, #21000, #26136, #21337, #31449, #10356, #23738, #31279, #18429, #12925, #26476, #7772, #28874, #8270, #5028, #5370, #541, #26307, #202, #28705, #24076, #10690, #5712, #18597, #2969, #16190, #13439, #33863, #23906, #5203, #26644, #3138, #13611, #11029, #21498, #3965, #27308, #24563, #3799, #876, #16513, #1036, #6373, #3466, #1203, #6543, #19590, #1379, #21834, #3632, #8772, #9271, #27476, #14271, #32279, #17016, #11684, #14438, #11516, #19423, #21996, #27138, #709, #24893, #21666, #24728, #11195, #11853, #22168, #13936, #26808, #32444, #22332, #8945, #26965, #16851, #32612, #29873, #24400, #6201, #11356, #9109, #19255, #30038, #14106, #29696, #32112, #32777, #8610, #19093, #29376, #5875, #6034, #16353, #3303, #29531, #13768, #24238, #16681, #22837, #23014, #25415, #30895, #27818, #9969, #23184, #25241, #1546, #6706, #20102, #7389, #12022, #30373, #14776, #17188, #9621, #33469, #1716, #28326, #17354, #4301, #17526, #6874, #22491, #33297, #4814, #9797, #12369, #15293, #32942, #12195, #22666, #30720, #12712, #15124, #30548, #20445, #27646, #7044, #12543, #17874, #25753, #33118, #9443, #20273, #2067, #27987, #33646, #4134, #2237, #7215, #17698, #19755, #30204, #14609, #25065, #19927, #1893, #4474, #14949, #28158, #4644, #25587, #28998, #13397, #15977, #23527, #23867, #5498, #7562, #334, #31067, #10480, #20793, #10820, #15643, #15468, #31407, #21300, #7900, #18046, #26094, #31740, #28831, #8068, #33987, #28490, #28663, #4987, #26603, #16150, #25922, #20626, #18385, #2416, #13218, #18553, #31237, #15810, #26434, #5329, #8231, #26265, #12883, #23359, #23694, #33820, #10143, #5158, #10314, #2753, #160, #3101, #21127, #18725, #10650, #7730, #31570, #18219, #2591, #2926, #13054, #29161, #20958, #5668, #13571, #24035, #8901, #31904, #27268, #32072, #27099, #18886, #8572, #16644, #27435, #32243, #19054, #3426, #10989, #3926, #5997, #14233, #3591, #24690, #16314, #29834, #11156, #14400, #997, #13730, #8735, #6335, #11481, #29494, #11316, #21460, #24527, #16473, #21627, #16813, #26927, #5836, #19219, #26771, #13898, #8398, #21958, #3261, #24365, #3762, #503, #835, #30000, #21794, #29655, #24198, #19553, #6160, #1164, #14065, #32405, #11646, #19385, #29334, #22129, #668, #32573, #9072, #6505, #16978, #22452, #33429, #22799, #20060, #33254, #30335, #11983, #30505, #1850, #32900, #30676, #2028, #15080, #30854, #17314, #33076, #4262, #4774, #22970, #9750, #27776, #12502, #7174, #9926, #7005, #14907, #17487, #22624, #25548, #6667, #20236, #1507, #24855, #25371, #4093, #9582, #17655, #12329, #9399, #1675, #1336, #28116, #6832, #19882, #4603, #14736, #30163, #27949, #17148, #25197, #11818, #20402, #27602, #12150, #7345, #22294, #4431, #17830, #28287, #32739, #14567, #9232, #19716, #25027, #10276, #12845, #18518, #13017, #23137, #18176, #29127, #15252, #20917, #23489, #18688, #23319, #23831, #13181, #10441, #23659, #20756, #2372, #31367, #26229, #33784, #21092, #26397, #5460, #21260, #7691, #33949, #28620, #25713, #13356, #120, #5118, #2890, #31538, #296, #7858, #5291, #18348, #28792, #20582, #2194, #15773, #10102, #2718, #10612, #31200, #8032, #28964, #15941, #10783, #31705, #12669, #31027, #8197, #7524, #33604, #15602, #18008, #28454, #4944, #15426, #25879, #26057, #2550, #16277, #29619, #26735, #5630, #24488, #11121, #11441, #21589, #14025, #19019, #801, #961, #3062, #32368, #3228, #32204, #23996, #13696, #21761, #32532, #3392, #24161, #8533, #16114, #9032, #32035, #19347, #8698, #631, #16441, #26566, #6122, #29460, #5963, #21918, #26893, #10950, #13862, #21426, #24327, #13533, #16606, #31867, #11283, #8862, #19976, #19181, #1121, #27059, #3552, #8361, #24647, #29789, #6293, #16769, #27228, #3722, #14192, #467, #11606, #18849, #29297, #22088, #5795, #33869, #28034, #5035, #28377, #25637, #4865, #1943, #17575, #2116, #7442, #4521, #2290, #7611, #20678, #2465, #22889, #4692, #9843, #10362, #28539, #15346, #33346, #18092, #12764, #15520, #12589, #20496, #23059, #28206, #1761, #6921, #15172, #25289, #33519, #25800, #14996, #10023, #23237, #30945, #31118, #17926, #17403, #12241, #33697, #22719, #30422, #25466, #27867 ),
 ( #14825, #12419, #10198, #23408, #25972, #20321, #30770, #4349, #33167, #7260, #12932, #9670, #20151, #30595, #7091, #17746, #715, #21343, #40, #18604, #26650, #31785, #208, #20840, #18937, #5718, #13269, #8445, #3145, #31953, #2976, #10869, #13445, #29043, #26143, #31285, #5546, #15693, #23912, #18768, #7948, #26482, #29212, #16027, #21504, #384, #7778, #2639, #8276, #13102, #18265, #5378, #28711, #16196, #13617, #13774, #24082, #548, #11035, #31455, #29382, #18436, #5209, #5882, #26313, #16359, #2802, #26814, #10696, #3310, #24244, #23575, #10529, #28880, #21006, #15857, #23744, #21177, #31619, #8116, #19261, #14112, #21672, #14615, #16687, #24900, #27315, #1386, #26971, #6549, #21840, #25071, #11690, #24406, #8951, #17023, #22174, #8778, #22002, #32120, #1209, #27144, #32285, #27482, #29703, #16519, #19429, #3472, #6207, #8617, #32618, #13942, #1042, #14444, #11201, #24570, #6713, #3638, #29879, #882, #30211, #32450, #11860, #11522, #6379, #22338, #16857, #19099, #3806, #29537, #6040, #14277, #24734, #11364, #9115, #19761, #19596, #30044, #3972, #32783, #9277, #17194, #27652, #4140, #7395, #12718, #25759, #7568, #27993, #9803, #4820, #20451, #32947, #15299, #22497, #1900, #12200, #2244, #7050, #6879, #22845, #23189, #33303, #9450, #17532, #33651, #20279, #33475, #25421, #19932, #20108, #30378, #18051, #28495, #10148, #27824, #9975, #17360, #4992, #30902, #30554, #4306, #30726, #20630, #4650, #22672, #23020, #17880, #17705, #4480, #12375, #14956, #7220, #28164, #28334, #15131, #25594, #14781, #31073, #25246, #1721, #2073, #1552, #33123, #15474, #12028, #9626, #12549, #29339, #5334, #29003, #29167, #31575, #3106, #22468, #16155, #5841, #31413, #7734, #12888, #26270, #13577, #18224, #2596, #20963, #23364, #15815, #5675, #7906, #509, #23532, #10485, #23699, #13059, #28670, #5504, #10994, #15984, #18559, #21467, #5163, #18390, #28836, #2932, #18892, #21305, #2758, #26608, #33825, #13224, #18730, #24040, #31909, #165, #15648, #26440, #8236, #10655, #25927, #10319, #8404, #13402, #23872, #2421, #20798, #31242, #26099, #21133, #8073, #340, #10825, #31745, #24531, #26933, #1172, #19558, #22135, #29662, #3266, #16650, #3431, #30005, #21798, #21632, #3596, #27440, #14070, #13735, #32249, #6510, #1002, #14238, #6166, #24204, #840, #673, #32744, #22299, #3932, #8576, #24695, #32078, #9237, #11651, #11322, #11162, #11486, #14407, #19391, #13904, #3767, #32578, #32411, #8741, #27104, #19225, #21963, #8906, #9077, #29838, #6340, #19059, #16983, #29499, #6003, #16818, #16319, #24370, #24861, #1341, #16477, #11822, #19721, #27273, #30168, #26777, #12334, #17835, #14741, #30858, #10108, #12155, #22456, #27611, #7009, #28291, #32905, #17319, #1680, #4098, #30510, #20407, #22629, #15257, #4267, #25202, #4436, #27781, #9405, #9755, #25719, #30681, #33261, #2199, #19887, #33083, #9586, #17660, #33608, #2033, #17492, #7351, #14572, #27954, #33434, #4779, #12674, #20066, #30341, #7179, #22975, #14912, #20587, #25032, #23143, #28121, #20241, #6672, #17153, #1512, #11987, #6839, #22804, #25376, #1857, #4608, #15085, #25553, #12508, #9931, #21096, #2555, #18522, #10617, #28459, #28968, #13022, #26401, #25884, #20761, #28625, #18012, #23494, #5464, #5123, #13361, #31205, #7696, #10446, #18182, #12850, #5296, #23835, #26234, #28798, #300, #2378, #15608, #26062, #13186, #21265, #31541, #33953, #15945, #4950, #20923, #2894, #10787, #31709, #31372, #33789, #2723, #8036, #7863, #8201, #15431, #31032, #126, #23663, #7529, #23324, #10281, #18354, #15778, #24910, #1050, #17202, #1731, #22182, #1396, #11530, #25256, #17031, #6890, #1218, #3814, #9460, #3980, #14122, #9123, #20120, #6217, #11870, #14453, #9637, #14286, #14792, #4150, #22345, #14623, #11698, #27326, #32792, #27661, #24743, #12036, #17371, #30388, #12211, #32627, #9285, #19605, #16698, #4317, #25079, #30052, #27834, #22506, #22683, #19769, #30220, #6720, #1560, #22013, #27154, #32958, #32458, #19942, #33134, #6556, #3646, #24579, #8958, #19439, #29887, #6388, #16865, #27491, #25433, #30564, #15142, #7061, #2256, #4831, #23545, #7582, #33836, #25770, #7230, #20642, #17716, #17543, #15485, #2085, #12387, #4662, #28003, #18060, #22856, #4490, #15311, #1910, #28505, #26110, #12560, #12730, #33314, #15660, #7407, #31253, #25606, #28175, #10333, #28346, #14966, #33488, #10496, #9813, #23200, #33663, #7, #23031, #5177, #5002, #10160, #25939, #9989, #20462, #31085, #2432, #30913, #12900, #7745, #20809, #2608, #17893, #23375, #18234, #20290, #28680, #13069, #30737, #8585, #3276, #32089, #3115, #11005, #13587, #18739, #26281, #31424, #29181, #15827, #24049, #18903, #8086, #26619, #29350, #5686, #21643, #16164, #7917, #2772, #518, #13236, #20974, #5514, #18401, #21475, #31922, #13913, #8414, #24214, #5850, #31586, #16329, #18573, #28847, #26785, #26451, #13744, #2942, #686, #352, #11172, #19069, #5346, #29509, #29014, #6013, #23710, #15995, #16487, #24380, #26943, #13413, #23881, #176, #853, #10835, #3443, #10666, #21145, #21314, #31755, #8246, #25687, #11832, #24540, #9087, #17166, #22309, #8917, #22143, #21808, #1352, #27284, #21973, #6682, #29850, #16659, #19568, #32755, #27451, #6350, #32588, #16828, #6521, #24704, #19734, #30017, #14247, #27116, #9248, #3609, #14081, #16992, #11332, #32421, #30179, #4110, #1011, #27623, #15224, #1181, #14417, #14583, #3942, #22469, #19400, #1525, #32257, #3776, #11494, #8750, #11662, #32918, #24870, #25043, #11999, #19234, #9417, #19902, #30825, #7318, #17803, #28261, #4745, #29671, #6177, #5264, #10756, #26201, #28768, #21234, #17979, #18150, #5091, #13155, #29099, #31513, #2522, #2860, #33575, #26030, #28935, #269, #31677, #20731, #25854, #2695, #18492, #28593, #16086, #10073, #8170, #23630, #15746, #18661, #15915, #26371, #7498, #23803, #97, #15576, #8007, #31341, #10414, #12817, #21063, #5434, #13330, #12991, #5604, #2167, #20554, #12641, #23111, #23462, #23290, #31000, #7663, #28429, #33924, #4919, #20892, #15399, #7833, #2345, #18322, #10586, #33758, #10250, #31171, #23970, #9008, #32507, #14169, #18826, #24463, #31843 ) ),
 .UNSPECIFIED., .F., .F., .T. ) 
 B_SPLINE_SURFACE_WITH_KNOTS ( ( 2, 2 ),
 ( 3, 2, 2, 2, 2, 2, 2, 2, 2, 2, 2, 2, 2, 2, 2, 2, 2, 2, 2, 2, 2, 2, 2, 2, 2, 2, 2, 2, 2, 2, 2, 2, 2, 2, 2, 2, 2, 2, 2, 2, 2, 2, 2, 2, 2, 2, 2, 2, 2, 2, 2, 2, 2, 2, 2, 2, 2, 2, 2, 2, 2, 2, 2, 2, 2, 2, 2, 2, 2, 2, 2, 2, 2, 2, 2, 2, 2, 2, 2, 2, 2, 2, 2, 2, 2, 2, 2, 2, 2, 2, 2, 2, 2, 2, 2, 2, 2, 2, 2, 2, 2, 2, 2, 2, 2, 2, 2, 2, 2, 2, 2, 2, 2, 2, 2, 2, 2, 2, 2, 2, 2, 2, 2, 2, 2, 2, 2, 2, 2, 2, 2, 2, 2, 2, 2, 2, 2, 2, 2, 2, 2, 2, 2, 2, 2, 2, 2, 2, 2, 2, 2, 2, 2, 2, 2, 2, 2, 2, 2, 2, 2, 2, 2, 2, 2, 2, 2, 2, 2, 2, 2, 2, 2, 2, 2, 2, 2, 2, 2, 2, 2, 2, 2, 2, 2, 2, 2, 2, 2, 2, 2, 2, 2, 2, 2, 2, 2, 2, 2, 2, 2, 2, 2, 2, 2, 2, 2, 2, 2, 2, 2, 2, 2, 2, 2, 2, 2, 2, 2, 2, 2, 2, 2, 2, 2, 2, 2, 2, 2, 2, 2, 2, 2, 2, 2, 2, 2, 2, 2, 2, 2, 2, 2, 2, 2, 2, 2, 2, 2, 2, 2, 2, 2, 2, 2, 2, 2, 2, 2, 2, 2, 2, 2, 2, 2, 2, 2, 2, 2, 2, 2, 2, 2, 2, 2, 2, 2, 2, 2, 2, 2, 2, 2, 2, 2, 2, 2, 2, 2, 2, 2, 2, 2, 2, 2, 2, 2, 2, 2, 2, 2, 2, 2, 2, 2, 2, 2, 2, 2, 2, 2, 2, 2, 2, 2, 2, 2, 2, 2, 2, 2, 2, 2, 2, 2, 2, 2, 2, 2, 2, 2, 2, 2, 2, 2, 2, 2, 2, 2, 2, 2, 2, 2, 2, 2, 2, 2, 2, 2, 2, 2, 2, 2, 2, 2, 2, 2, 2, 2, 2, 2, 2, 2, 2, 2, 2, 2, 2, 2, 2, 2, 2, 2, 2, 2, 2, 2, 2, 2, 2, 2, 2, 2, 2, 2, 2, 2, 2, 2, 2, 3 ),
 ( 0.000000000000000000, 1.000000000000000000 ),
 ( 0.000000000000000000, 0.002564102564102564100, 0.005128205128205128201, 0.007692307692307692735, 0.01025641025641025640, 0.01282051282051282007, 0.01538461538461538547, 0.01794871794871794740, 0.02051282051282051280, 0.02307692307692307820, 0.02564102564102564014, 0.02820512820512820554, 0.03076923076923077094, 0.03333333333333333287, 0.03589743589743589480, 0.03846153846153846367, 0.04102564102564102561, 0.04358974358974358754, 0.04615384615384615641, 0.04871794871794871834, 0.05128205128205128027, 0.05384615384615384914, 0.05641025641025641107, 0.05897435897435897301, 0.06153846153846154188, 0.06410256410256409687, 0.06666666666666666574, 0.06923076923076923461, 0.07179487179487178961, 0.07435897435897435848, 0.07692307692307692735, 0.07948717948717948234, 0.08205128205128205121, 0.08461538461538462008, 0.08717948717948717507, 0.08974358974358974395, 0.09230769230769231282, 0.09487179487179486781, 0.09743589743589743668, 0.1000000000000000056, 0.1025641025641025605, 0.1051282051282051294, 0.1076923076923076983, 0.1102564102564102533, 0.1128205128205128221, 0.1153846153846153910, 0.1179487179487179460, 0.1205128205128205149, 0.1230769230769230838, 0.1256410256410256387, 0.1282051282051281937, 0.1307692307692307765, 0.1333333333333333315, 0.1358974358974358865, 0.1384615384615384692, 0.1410256410256410242, 0.1435897435897435792, 0.1461538461538461620, 0.1487179487179487170, 0.1512820512820512719, 0.1538461538461538547, 0.1564102564102564097, 0.1589743589743589647, 0.1615384615384615474, 0.1641025641025641024, 0.1666666666666666574, 0.1692307692307692402, 0.1717948717948717952, 0.1743589743589743501, 0.1769230769230769329, 0.1794871794871794879, 0.1820512820512820429, 0.1846153846153846256, 0.1871794871794871806, 0.1897435897435897356, 0.1923076923076923184, 0.1948717948717948734, 0.1974358974358974284, 0.2000000000000000111, 0.2025641025641025661, 0.2051282051282051211, 0.2076923076923077038, 0.2102564102564102588, 0.2128205128205128138, 0.2153846153846153966, 0.2179487179487179516, 0.2205128205128205066, 0.2230769230769230893, 0.2256410256410256443, 0.2282051282051281993, 0.2307692307692307820, 0.2333333333333333370, 0.2358974358974358920, 0.2384615384615384748, 0.2410256410256410298, 0.2435897435897435848, 0.2461538461538461675, 0.2487179487179487225, 0.2512820512820512775, 0.2538461538461538325, 0.2564102564102563875, 0.2589743589743589980, 0.2615384615384615530, 0.2641025641025641080, 0.2666666666666666630, 0.2692307692307692180, 0.2717948717948717730, 0.2743589743589743835, 0.2769230769230769384, 0.2794871794871794934, 0.2820512820512820484, 0.2846153846153846034, 0.2871794871794871584, 0.2897435897435897689, 0.2923076923076923239, 0.2948717948717948789, 0.2974358974358974339, 0.2999999999999999889, 0.3025641025641025439, 0.3051282051282051544, 0.3076923076923077094, 0.3102564102564102644, 0.3128205128205128194, 0.3153846153846153744, 0.3179487179487179294, 0.3205128205128205399, 0.3230769230769230949, 0.3256410256410256499, 0.3282051282051282048, 0.3307692307692307598, 0.3333333333333333148, 0.3358974358974358698, 0.3384615384615384803, 0.3410256410256410353, 0.3435897435897435903, 0.3461538461538461453, 0.3487179487179487003, 0.3512820512820512553, 0.3538461538461538658, 0.3564102564102564208, 0.3589743589743589758, 0.3615384615384615308, 0.3641025641025640858, 0.3666666666666666408, 0.3692307692307692513, 0.3717948717948718063, 0.3743589743589743613, 0.3769230769230769162, 0.3794871794871794712, 0.3820512820512820262, 0.3846153846153846367, 0.3871794871794871917, 0.3897435897435897467, 0.3923076923076923017, 0.3948717948717948567, 0.3974358974358974117, 0.4000000000000000222, 0.4025641025641025772, 0.4051282051282051322, 0.4076923076923076872, 0.4102564102564102422, 0.4128205128205127972, 0.4153846153846154077, 0.4179487179487179627, 0.4205128205128205177, 0.4230769230769230727, 0.4256410256410256276, 0.4282051282051281826, 0.4307692307692307931, 0.4333333333333333481, 0.4358974358974359031, 0.4384615384615384581, 0.4410256410256410131, 0.4435897435897435681, 0.4461538461538461786, 0.4487179487179487336, 0.4512820512820512886, 0.4538461538461538436, 0.4564102564102563986, 0.4589743589743589536, 0.4615384615384615641, 0.4641025641025641191, 0.4666666666666666741, 0.4692307692307692291, 0.4717948717948717841, 0.4743589743589743390, 0.4769230769230769496, 0.4794871794871795045, 0.4820512820512820595, 0.4846153846153846145, 0.4871794871794871695, 0.4897435897435897245, 0.4923076923076923350, 0.4948717948717948900, 0.4974358974358974450, 0.5000000000000000000, 0.5025641025641025550, 0.5051282051282051100, 0.5076923076923076650, 0.5102564102564102200, 0.5128205128205127750, 0.5153846153846153300, 0.5179487179487179960, 0.5205128205128205510, 0.5230769230769231060, 0.5256410256410256610, 0.5282051282051282159, 0.5307692307692307709, 0.5333333333333333259, 0.5358974358974358809, 0.5384615384615384359, 0.5410256410256409909, 0.5435897435897435459, 0.5461538461538461009, 0.5487179487179487669, 0.5512820512820513219, 0.5538461538461538769, 0.5564102564102564319, 0.5589743589743589869, 0.5615384615384615419, 0.5641025641025640969, 0.5666666666666666519, 0.5692307692307692069, 0.5717948717948717618, 0.5743589743589743168, 0.5769230769230768718, 0.5794871794871795379, 0.5820512820512820928, 0.5846153846153846478, 0.5871794871794872028, 0.5897435897435897578, 0.5923076923076923128, 0.5948717948717948678, 0.5974358974358974228, 0.5999999999999999778, 0.6025641025641025328, 0.6051282051282050878, 0.6076923076923076428, 0.6102564102564103088, 0.6128205128205128638, 0.6153846153846154188, 0.6179487179487179738, 0.6205128205128205288, 0.6230769230769230838, 0.6256410256410256387, 0.6282051282051281937, 0.6307692307692307487, 0.6333333333333333037, 0.6358974358974358587, 0.6384615384615384137, 0.6410256410256410797, 0.6435897435897436347, 0.6461538461538461897, 0.6487179487179487447, 0.6512820512820512997, 0.6538461538461538547, 0.6564102564102564097, 0.6589743589743589647, 0.6615384615384615197, 0.6641025641025640747, 0.6666666666666666297, 0.6692307692307691847, 0.6717948717948717396, 0.6743589743589744057, 0.6769230769230769607, 0.6794871794871795156, 0.6820512820512820706, 0.6846153846153846256, 0.6871794871794871806, 0.6897435897435897356, 0.6923076923076922906, 0.6948717948717948456, 0.6974358974358974006, 0.6999999999999999556, 0.7025641025641025106, 0.7051282051282051766, 0.7076923076923077316, 0.7102564102564102866, 0.7128205128205128416, 0.7153846153846153966, 0.7179487179487179516, 0.7205128205128205066, 0.7230769230769230616, 0.7256410256410256165, 0.7282051282051281715, 0.7307692307692307265, 0.7333333333333332815, 0.7358974358974359475, 0.7384615384615385025, 0.7410256410256410575, 0.7435897435897436125, 0.7461538461538461675, 0.7487179487179487225, 0.7512820512820512775, 0.7538461538461538325, 0.7564102564102563875, 0.7589743589743589425, 0.7615384615384614975, 0.7641025641025640525, 0.7666666666666667185, 0.7692307692307692735, 0.7717948717948718285, 0.7743589743589743835, 0.7769230769230769384, 0.7794871794871794934, 0.7820512820512820484, 0.7846153846153846034, 0.7871794871794871584, 0.7897435897435897134, 0.7923076923076922684, 0.7948717948717948234, 0.7974358974358974894, 0.8000000000000000444, 0.8025641025641025994, 0.8051282051282051544, 0.8076923076923077094, 0.8102564102564102644, 0.8128205128205128194, 0.8153846153846153744, 0.8179487179487179294, 0.8205128205128204844, 0.8230769230769230393, 0.8256410256410255943, 0.8282051282051282604, 0.8307692307692308153, 0.8333333333333333703, 0.8358974358974359253, 0.8384615384615384803, 0.8410256410256410353, 0.8435897435897435903, 0.8461538461538461453, 0.8487179487179487003, 0.8512820512820512553, 0.8538461538461538103, 0.8564102564102563653, 0.8589743589743589203, 0.8615384615384615863, 0.8641025641025641413, 0.8666666666666666963, 0.8692307692307692513, 0.8717948717948718063, 0.8743589743589743613, 0.8769230769230769162, 0.8794871794871794712, 0.8820512820512820262, 0.8846153846153845812, 0.8871794871794871362, 0.8897435897435896912, 0.8923076923076923572, 0.8948717948717949122, 0.8974358974358974672, 0.9000000000000000222, 0.9025641025641025772, 0.9051282051282051322, 0.9076923076923076872, 0.9102564102564102422, 0.9128205128205127972, 0.9153846153846153522, 0.9179487179487179072, 0.9205128205128204621, 0.9230769230769231282, 0.9256410256410256832, 0.9282051282051282382, 0.9307692307692307931, 0.9333333333333333481, 0.9358974358974359031, 0.9384615384615384581, 0.9410256410256410131, 0.9435897435897435681, 0.9461538461538461231, 0.9487179487179486781, 0.9512820512820512331, 0.9538461538461538991, 0.9564102564102564541, 0.9589743589743590091, 0.9615384615384615641, 0.9641025641025641191, 0.9666666666666666741, 0.9692307692307692291, 0.9717948717948717841, 0.9743589743589743390, 0.9769230769230768940, 0.9794871794871794490, 0.9820512820512820040, 0.9846153846153846700, 0.9871794871794872250, 0.9897435897435897800, 0.9923076923076923350, 0.9948717948717948900, 0.9974358974358974450, 1.000000000000000000 ),
 .UNSPECIFIED. ) 
 GEOMETRIC_REPRESENTATION_ITEM ( )  RATIONAL_B_SPLINE_SURFACE ( (
 ( 1.000000000000000000, 0.9510565162951535312, 1.000000000000000000, 0.9510565162951535312, 1.000000000000000000, 0.9510565162951535312, 1.000000000000000000, 0.9510565162951535312, 1.000000000000000000, 0.9510565162951535312, 1.000000000000000000, 0.9510565162951535312, 1.000000000000000000, 0.9510565162951535312, 1.000000000000000000, 0.9510565162951535312, 1.000000000000000000, 0.9510565162951535312, 1.000000000000000000, 0.9510565162951535312, 1.000000000000000000, 0.9510565162951535312, 1.000000000000000000, 0.9510565162951535312, 1.000000000000000000, 0.9510565162951535312, 1.000000000000000000, 0.9510565162951535312, 1.000000000000000000, 0.9510565162951535312, 1.000000000000000000, 0.9510565162951535312, 1.000000000000000000, 0.9510565162951535312, 1.000000000000000000, 0.9510565162951535312, 1.000000000000000000, 0.9510565162951535312, 1.000000000000000000, 0.9510565162951535312, 1.000000000000000000, 0.9510565162951535312, 1.000000000000000000, 0.9510565162951535312, 1.000000000000000000, 0.9510565162951535312, 1.000000000000000000, 0.9510565162951535312, 1.000000000000000000, 0.9510565162951535312, 1.000000000000000000, 0.9510565162951535312, 1.000000000000000000, 0.9510565162951535312, 1.000000000000000000, 0.9510565162951535312, 1.000000000000000000, 0.9510565162951535312, 1.000000000000000000, 0.9510565162951535312, 1.000000000000000000, 0.9510565162951535312, 1.000000000000000000, 0.9510565162951535312, 1.000000000000000000, 0.9510565162951535312, 1.000000000000000000, 0.9510565162951535312, 1.000000000000000000, 0.9510565162951535312, 1.000000000000000000, 0.9510565162951535312, 1.000000000000000000, 0.9510565162951535312, 1.000000000000000000, 0.9510565162951535312, 1.000000000000000000, 0.9510565162951535312, 1.000000000000000000, 0.9510565162951535312, 1.000000000000000000, 0.9510565162951535312, 1.000000000000000000, 0.9510565162951535312, 1.000000000000000000, 0.9510565162951535312, 1.000000000000000000, 0.9510565162951535312, 1.000000000000000000, 0.9510565162951535312, 1.000000000000000000, 0.9510565162951535312, 1.000000000000000000, 0.9510565162951535312, 1.000000000000000000, 0.9510565162951535312, 1.000000000000000000, 0.9510565162951535312, 1.000000000000000000, 0.9510565162951535312, 1.000000000000000000, 0.9510565162951535312, 1.000000000000000000, 0.9510565162951535312, 1.000000000000000000, 0.9510565162951535312, 1.000000000000000000, 0.9510565162951535312, 1.000000000000000000, 0.9510565162951535312, 1.000000000000000000, 0.9510565162951535312, 1.000000000000000000, 0.9510565162951535312, 1.000000000000000000, 0.9510565162951535312, 1.000000000000000000, 0.9510565162951535312, 1.000000000000000000, 0.9510565162951535312, 1.000000000000000000, 0.9510565162951535312, 1.000000000000000000, 0.9510565162951535312, 1.000000000000000000, 0.9510565162951535312, 1.000000000000000000, 0.9510565162951535312, 1.000000000000000000, 0.9510565162951535312, 1.000000000000000000, 0.9510565162951535312, 1.000000000000000000, 0.9510565162951535312, 1.000000000000000000, 0.9510565162951535312, 1.000000000000000000, 0.9510565162951535312, 1.000000000000000000, 0.9510565162951535312, 1.000000000000000000, 0.9510565162951535312, 1.000000000000000000, 0.9510565162951535312, 1.000000000000000000, 0.9510565162951535312, 1.000000000000000000, 0.9510565162951535312, 1.000000000000000000, 0.9510565162951535312, 1.000000000000000000, 0.9510565162951535312, 1.000000000000000000, 0.9510565162951535312, 1.000000000000000000, 0.9510565162951535312, 1.000000000000000000, 0.9510565162951535312, 1.000000000000000000, 0.9510565162951535312, 1.000000000000000000, 0.9510565162951535312, 1.000000000000000000, 0.9510565162951535312, 1.000000000000000000, 0.9510565162951535312, 1.000000000000000000, 0.9510565162951535312, 1.000000000000000000, 0.9510565162951535312, 1.000000000000000000, 0.9510565162951535312, 1.000000000000000000, 0.9510565162951535312, 1.000000000000000000, 0.9510565162951535312, 1.000000000000000000, 0.9510565162951535312, 1.000000000000000000, 0.9510565162951535312, 1.000000000000000000, 0.9510565162951535312, 1.000000000000000000, 0.9510565162951535312, 1.000000000000000000, 0.9510565162951535312, 1.000000000000000000, 0.9510565162951535312, 1.000000000000000000, 0.9510565162951535312, 1.000000000000000000, 0.9510565162951535312, 1.000000000000000000, 0.9510565162951535312, 1.000000000000000000, 0.9510565162951535312, 1.000000000000000000, 0.9510565162951535312, 1.000000000000000000, 0.9510565162951535312, 1.000000000000000000, 0.9510565162951535312, 1.000000000000000000, 0.9510565162951535312, 1.000000000000000000, 0.9510565162951535312, 1.000000000000000000, 0.9510565162951535312, 1.000000000000000000, 0.9510565162951535312, 1.000000000000000000, 0.9510565162951535312, 1.000000000000000000, 0.9510565162951535312, 1.000000000000000000, 0.9510565162951535312, 1.000000000000000000, 0.9510565162951535312, 1.000000000000000000, 0.9510565162951535312, 1.000000000000000000, 0.9510565162951535312, 1.000000000000000000, 0.9510565162951535312, 1.000000000000000000, 0.9510565162951535312, 1.000000000000000000, 0.9510565162951535312, 1.000000000000000000, 0.9510565162951535312, 1.000000000000000000, 0.9510565162951535312, 1.000000000000000000, 0.9510565162951535312, 1.000000000000000000, 0.9510565162951535312, 1.000000000000000000, 0.9510565162951535312, 1.000000000000000000, 0.9510565162951535312, 1.000000000000000000, 0.9510565162951535312, 1.000000000000000000, 0.9510565162951535312, 1.000000000000000000, 0.9510565162951535312, 1.000000000000000000, 0.9510565162951535312, 1.000000000000000000, 0.9510565162951535312, 1.000000000000000000, 0.9510565162951535312, 1.000000000000000000, 0.9510565162951535312, 1.000000000000000000, 0.9510565162951535312, 1.000000000000000000, 0.9510565162951535312, 1.000000000000000000, 0.9510565162951535312, 1.000000000000000000, 0.9510565162951535312, 1.000000000000000000, 0.9510565162951535312, 1.000000000000000000, 0.9510565162951535312, 1.000000000000000000, 0.9510565162951535312, 1.000000000000000000, 0.9510565162951535312, 1.000000000000000000, 0.9510565162951535312, 1.000000000000000000, 0.9510565162951535312, 1.000000000000000000, 0.9510565162951535312, 1.000000000000000000, 0.9510565162951535312, 1.000000000000000000, 0.9510565162951535312, 1.000000000000000000, 0.9510565162951535312, 1.000000000000000000, 0.9510565162951535312, 1.000000000000000000, 0.9510565162951535312, 1.000000000000000000, 0.9510565162951535312, 1.000000000000000000, 0.9510565162951535312, 1.000000000000000000, 0.9510565162951535312, 1.000000000000000000, 0.9510565162951535312, 1.000000000000000000, 0.9510565162951535312, 1.000000000000000000, 0.9510565162951535312, 1.000000000000000000, 0.9510565162951535312, 1.000000000000000000, 0.9510565162951535312, 1.000000000000000000, 0.9510565162951535312, 1.000000000000000000, 0.9510565162951535312, 1.000000000000000000, 0.9510565162951535312, 1.000000000000000000, 0.9510565162951535312, 1.000000000000000000, 0.9510565162951535312, 1.000000000000000000, 0.9510565162951535312, 1.000000000000000000, 0.9510565162951535312, 1.000000000000000000, 0.9510565162951535312, 1.000000000000000000, 0.9510565162951535312, 1.000000000000000000, 0.9510565162951535312, 1.000000000000000000, 0.9510565162951535312, 1.000000000000000000, 0.9510565162951535312, 1.000000000000000000, 0.9510565162951535312, 1.000000000000000000, 0.9510565162951535312, 1.000000000000000000, 0.9510565162951535312, 1.000000000000000000, 0.9510565162951535312, 1.000000000000000000, 0.9510565162951535312, 1.000000000000000000, 0.9510565162951535312, 1.000000000000000000, 0.9510565162951535312, 1.000000000000000000, 0.9510565162951535312, 1.000000000000000000, 0.9510565162951535312, 1.000000000000000000, 0.9510565162951535312, 1.000000000000000000, 0.9510565162951535312, 1.000000000000000000, 0.9510565162951535312, 1.000000000000000000, 0.9510565162951535312, 1.000000000000000000, 0.9510565162951535312, 1.000000000000000000, 0.9510565162951535312, 1.000000000000000000, 0.9510565162951535312, 1.000000000000000000, 0.9510565162951535312, 1.000000000000000000, 0.9510565162951535312, 1.000000000000000000, 0.9510565162951535312, 1.000000000000000000, 0.9510565162951535312, 1.000000000000000000, 0.9510565162951535312, 1.000000000000000000, 0.9510565162951535312, 1.000000000000000000, 0.9510565162951535312, 1.000000000000000000, 0.9510565162951535312, 1.000000000000000000, 0.9510565162951535312, 1.000000000000000000, 0.9510565162951535312, 1.000000000000000000, 0.9510565162951535312, 1.000000000000000000, 0.9510565162951535312, 1.000000000000000000, 0.9510565162951535312, 1.000000000000000000, 0.9510565162951535312, 1.000000000000000000, 0.9510565162951535312, 1.000000000000000000, 0.9510565162951535312, 1.000000000000000000, 0.9510565162951535312, 1.000000000000000000, 0.9510565162951535312, 1.000000000000000000, 0.9510565162951535312, 1.000000000000000000, 0.9510565162951535312, 1.000000000000000000, 0.9510565162951535312, 1.000000000000000000, 0.9510565162951535312, 1.000000000000000000, 0.9510565162951535312, 1.000000000000000000, 0.9510565162951535312, 1.000000000000000000, 0.9510565162951535312, 1.000000000000000000, 0.9510565162951535312, 1.000000000000000000, 0.9510565162951535312, 1.000000000000000000, 0.9510565162951535312, 1.000000000000000000, 0.9510565162951535312, 1.000000000000000000, 0.9510565162951535312, 1.000000000000000000, 0.9510565162951535312, 1.000000000000000000, 0.9510565162951535312, 1.000000000000000000, 0.9510565162951535312, 1.000000000000000000, 0.9510565162951535312, 1.000000000000000000, 0.9510565162951535312, 1.000000000000000000, 0.9510565162951535312, 1.000000000000000000, 0.9510565162951535312, 1.000000000000000000, 0.9510565162951535312, 1.000000000000000000, 0.9510565162951535312, 1.000000000000000000, 0.9510565162951535312, 1.000000000000000000, 0.9510565162951535312, 1.000000000000000000, 0.9510565162951535312, 1.000000000000000000, 0.9510565162951535312, 1.000000000000000000, 0.9510565162951535312, 1.000000000000000000, 0.9510565162951535312, 1.000000000000000000, 0.9510565162951535312, 1.000000000000000000, 0.9510565162951535312, 1.000000000000000000, 0.9510565162951535312, 1.000000000000000000, 0.9510565162951535312, 1.000000000000000000, 0.9510565162951535312, 1.000000000000000000, 0.9510565162951535312, 1.000000000000000000, 0.9510565162951535312, 1.000000000000000000, 0.9510565162951535312, 1.000000000000000000, 0.9510565162951535312, 1.000000000000000000, 0.9510565162951535312, 1.000000000000000000, 0.9510565162951535312, 1.000000000000000000, 0.9510565162951535312, 1.000000000000000000, 0.9510565162951535312, 1.000000000000000000, 0.9510565162951535312, 1.000000000000000000, 0.9510565162951535312, 1.000000000000000000, 0.9510565162951535312, 1.000000000000000000, 0.9510565162951535312, 1.000000000000000000, 0.9510565162951535312, 1.000000000000000000, 0.9510565162951535312, 1.000000000000000000, 0.9510565162951535312, 1.000000000000000000, 0.9510565162951535312, 1.000000000000000000, 0.9510565162951535312, 1.000000000000000000, 0.9510565162951535312, 1.000000000000000000, 0.9510565162951535312, 1.000000000000000000, 0.9510565162951535312, 1.000000000000000000, 0.9510565162951535312, 1.000000000000000000, 0.9510565162951535312, 1.000000000000000000, 0.9510565162951535312, 1.000000000000000000, 0.9510565162951535312, 1.000000000000000000, 0.9510565162951535312, 1.000000000000000000, 0.9510565162951535312, 1.000000000000000000, 0.9510565162951535312, 1.000000000000000000, 0.9510565162951535312, 1.000000000000000000, 0.9510565162951535312, 1.000000000000000000, 0.9510565162951535312, 1.000000000000000000, 0.9510565162951535312, 1.000000000000000000, 0.9510565162951535312, 1.000000000000000000, 0.9510565162951535312, 1.000000000000000000, 0.9510565162951535312, 1.000000000000000000, 0.9510565162951535312, 1.000000000000000000, 0.9510565162951535312, 1.000000000000000000, 0.9510565162951535312, 1.000000000000000000, 0.9510565162951535312, 1.000000000000000000, 0.9510565162951535312, 1.000000000000000000, 0.9510565162951535312, 1.000000000000000000, 0.9510565162951535312, 1.000000000000000000, 0.9510565162951535312, 1.000000000000000000, 0.9510565162951535312, 1.000000000000000000, 0.9510565162951535312, 1.000000000000000000, 0.9510565162951535312, 1.000000000000000000, 0.9510565162951535312, 1.000000000000000000, 0.9510565162951535312, 1.000000000000000000, 0.9510565162951535312, 1.000000000000000000, 0.9510565162951535312, 1.000000000000000000, 0.9510565162951535312, 1.000000000000000000, 0.9510565162951535312, 1.000000000000000000, 0.9510565162951535312, 1.000000000000000000, 0.9510565162951535312, 1.000000000000000000, 0.9510565162951535312, 1.000000000000000000, 0.9510565162951535312, 1.000000000000000000, 0.9510565162951535312, 1.000000000000000000, 0.9510565162951535312, 1.000000000000000000, 0.9510565162951535312, 1.000000000000000000, 0.9510565162951535312, 1.000000000000000000, 0.9510565162951535312, 1.000000000000000000, 0.9510565162951535312, 1.000000000000000000, 0.9510565162951535312, 1.000000000000000000, 0.9510565162951535312, 1.000000000000000000, 0.9510565162951535312, 1.000000000000000000, 0.9510565162951535312, 1.000000000000000000, 0.9510565162951535312, 1.000000000000000000, 0.9510565162951535312, 1.000000000000000000, 0.9510565162951535312, 1.000000000000000000, 0.9510565162951535312, 1.000000000000000000, 0.9510565162951535312, 1.000000000000000000, 0.9510565162951535312, 1.000000000000000000, 0.9510565162951535312, 1.000000000000000000, 0.9510565162951535312, 1.000000000000000000, 0.9510565162951535312, 1.000000000000000000, 0.9510565162951535312, 1.000000000000000000, 0.9510565162951535312, 1.000000000000000000, 0.9510565162951535312, 1.000000000000000000, 0.9510565162951535312, 1.000000000000000000, 0.9510565162951535312, 1.000000000000000000, 0.9510565162951535312, 1.000000000000000000, 0.9510565162951535312, 1.000000000000000000, 0.9510565162951535312, 1.000000000000000000, 0.9510565162951535312, 1.000000000000000000, 0.9510565162951535312, 1.000000000000000000, 0.9510565162951535312, 1.000000000000000000, 0.9510565162951535312, 1.000000000000000000, 0.9510565162951535312, 1.000000000000000000, 0.9510565162951535312, 1.000000000000000000, 0.9510565162951535312, 1.000000000000000000, 0.9510565162951535312, 1.000000000000000000, 0.9510565162951535312, 1.000000000000000000, 0.9510565162951535312, 1.000000000000000000, 0.9510565162951535312, 1.000000000000000000, 0.9510565162951535312, 1.000000000000000000, 0.9510565162951535312, 1.000000000000000000, 0.9510565162951535312, 1.000000000000000000, 0.9510565162951535312, 1.000000000000000000, 0.9510565162951535312, 1.000000000000000000, 0.9510565162951535312, 1.000000000000000000, 0.9510565162951535312, 1.000000000000000000, 0.9510565162951535312, 1.000000000000000000, 0.9510565162951535312, 1.000000000000000000, 0.9510565162951535312, 1.000000000000000000, 0.9510565162951535312, 1.000000000000000000, 0.9510565162951535312, 1.000000000000000000, 0.9510565162951535312, 1.000000000000000000, 0.9510565162951535312, 1.000000000000000000, 0.9510565162951535312, 1.000000000000000000, 0.9510565162951535312, 1.000000000000000000, 0.9510565162951535312, 1.000000000000000000, 0.9510565162951535312, 1.000000000000000000, 0.9510565162951535312, 1.000000000000000000, 0.9510565162951535312, 1.000000000000000000, 0.9510565162951535312, 1.000000000000000000, 0.9510565162951535312, 1.000000000000000000, 0.9510565162951535312, 1.000000000000000000, 0.9510565162951535312, 1.000000000000000000, 0.9510565162951535312, 1.000000000000000000, 0.9510565162951535312, 1.000000000000000000, 0.9510565162951535312, 1.000000000000000000, 0.9510565162951535312, 1.000000000000000000, 0.9510565162951535312, 1.000000000000000000, 0.9510565162951535312, 1.000000000000000000, 0.9510565162951535312, 1.000000000000000000, 0.9510565162951535312, 1.000000000000000000, 0.9510565162951535312, 1.000000000000000000, 0.9510565162951535312, 1.000000000000000000, 0.9510565162951535312, 1.000000000000000000, 0.9510565162951535312, 1.000000000000000000, 0.9510565162951535312, 1.000000000000000000, 0.9510565162951535312, 1.000000000000000000, 0.9510565162951535312, 1.000000000000000000, 0.9510565162951535312, 1.000000000000000000, 0.9510565162951535312, 1.000000000000000000, 0.9510565162951535312, 1.000000000000000000, 0.9510565162951535312, 1.000000000000000000, 0.9510565162951535312, 1.000000000000000000, 0.9510565162951535312, 1.000000000000000000, 0.9510565162951535312, 1.000000000000000000, 0.9510565162951535312, 1.000000000000000000, 0.9510565162951535312, 1.000000000000000000, 0.9510565162951535312, 1.000000000000000000, 0.9510565162951535312, 1.000000000000000000, 0.9510565162951535312, 1.000000000000000000, 0.9510565162951535312, 1.000000000000000000, 0.9510565162951535312, 1.000000000000000000, 0.9510565162951535312, 1.000000000000000000, 0.9510565162951535312, 1.000000000000000000, 0.9510565162951535312, 1.000000000000000000, 0.9510565162951535312, 1.000000000000000000, 0.9510565162951535312, 1.000000000000000000, 0.9510565162951535312, 1.000000000000000000, 0.9510565162951535312, 1.000000000000000000, 0.9510565162951535312, 1.000000000000000000, 0.9510565162951535312, 1.000000000000000000, 0.9510565162951535312, 1.000000000000000000, 0.9510565162951535312, 1.000000000000000000, 0.9510565162951535312, 1.000000000000000000, 0.9510565162951535312, 1.000000000000000000, 0.9510565162951535312, 1.000000000000000000, 0.9510565162951535312, 1.000000000000000000),
 ( 1.000000000000000000, 0.9510565162951535312, 1.000000000000000000, 0.9510565162951535312, 1.000000000000000000, 0.9510565162951535312, 1.000000000000000000, 0.9510565162951535312, 1.000000000000000000, 0.9510565162951535312, 1.000000000000000000, 0.9510565162951535312, 1.000000000000000000, 0.9510565162951535312, 1.000000000000000000, 0.9510565162951535312, 1.000000000000000000, 0.9510565162951535312, 1.000000000000000000, 0.9510565162951535312, 1.000000000000000000, 0.9510565162951535312, 1.000000000000000000, 0.9510565162951535312, 1.000000000000000000, 0.9510565162951535312, 1.000000000000000000, 0.9510565162951535312, 1.000000000000000000, 0.9510565162951535312, 1.000000000000000000, 0.9510565162951535312, 1.000000000000000000, 0.9510565162951535312, 1.000000000000000000, 0.9510565162951535312, 1.000000000000000000, 0.9510565162951535312, 1.000000000000000000, 0.9510565162951535312, 1.000000000000000000, 0.9510565162951535312, 1.000000000000000000, 0.9510565162951535312, 1.000000000000000000, 0.9510565162951535312, 1.000000000000000000, 0.9510565162951535312, 1.000000000000000000, 0.9510565162951535312, 1.000000000000000000, 0.9510565162951535312, 1.000000000000000000, 0.9510565162951535312, 1.000000000000000000, 0.9510565162951535312, 1.000000000000000000, 0.9510565162951535312, 1.000000000000000000, 0.9510565162951535312, 1.000000000000000000, 0.9510565162951535312, 1.000000000000000000, 0.9510565162951535312, 1.000000000000000000, 0.9510565162951535312, 1.000000000000000000, 0.9510565162951535312, 1.000000000000000000, 0.9510565162951535312, 1.000000000000000000, 0.9510565162951535312, 1.000000000000000000, 0.9510565162951535312, 1.000000000000000000, 0.9510565162951535312, 1.000000000000000000, 0.9510565162951535312, 1.000000000000000000, 0.9510565162951535312, 1.000000000000000000, 0.9510565162951535312, 1.000000000000000000, 0.9510565162951535312, 1.000000000000000000, 0.9510565162951535312, 1.000000000000000000, 0.9510565162951535312, 1.000000000000000000, 0.9510565162951535312, 1.000000000000000000, 0.9510565162951535312, 1.000000000000000000, 0.9510565162951535312, 1.000000000000000000, 0.9510565162951535312, 1.000000000000000000, 0.9510565162951535312, 1.000000000000000000, 0.9510565162951535312, 1.000000000000000000, 0.9510565162951535312, 1.000000000000000000, 0.9510565162951535312, 1.000000000000000000, 0.9510565162951535312, 1.000000000000000000, 0.9510565162951535312, 1.000000000000000000, 0.9510565162951535312, 1.000000000000000000, 0.9510565162951535312, 1.000000000000000000, 0.9510565162951535312, 1.000000000000000000, 0.9510565162951535312, 1.000000000000000000, 0.9510565162951535312, 1.000000000000000000, 0.9510565162951535312, 1.000000000000000000, 0.9510565162951535312, 1.000000000000000000, 0.9510565162951535312, 1.000000000000000000, 0.9510565162951535312, 1.000000000000000000, 0.9510565162951535312, 1.000000000000000000, 0.9510565162951535312, 1.000000000000000000, 0.9510565162951535312, 1.000000000000000000, 0.9510565162951535312, 1.000000000000000000, 0.9510565162951535312, 1.000000000000000000, 0.9510565162951535312, 1.000000000000000000, 0.9510565162951535312, 1.000000000000000000, 0.9510565162951535312, 1.000000000000000000, 0.9510565162951535312, 1.000000000000000000, 0.9510565162951535312, 1.000000000000000000, 0.9510565162951535312, 1.000000000000000000, 0.9510565162951535312, 1.000000000000000000, 0.9510565162951535312, 1.000000000000000000, 0.9510565162951535312, 1.000000000000000000, 0.9510565162951535312, 1.000000000000000000, 0.9510565162951535312, 1.000000000000000000, 0.9510565162951535312, 1.000000000000000000, 0.9510565162951535312, 1.000000000000000000, 0.9510565162951535312, 1.000000000000000000, 0.9510565162951535312, 1.000000000000000000, 0.9510565162951535312, 1.000000000000000000, 0.9510565162951535312, 1.000000000000000000, 0.9510565162951535312, 1.000000000000000000, 0.9510565162951535312, 1.000000000000000000, 0.9510565162951535312, 1.000000000000000000, 0.9510565162951535312, 1.000000000000000000, 0.9510565162951535312, 1.000000000000000000, 0.9510565162951535312, 1.000000000000000000, 0.9510565162951535312, 1.000000000000000000, 0.9510565162951535312, 1.000000000000000000, 0.9510565162951535312, 1.000000000000000000, 0.9510565162951535312, 1.000000000000000000, 0.9510565162951535312, 1.000000000000000000, 0.9510565162951535312, 1.000000000000000000, 0.9510565162951535312, 1.000000000000000000, 0.9510565162951535312, 1.000000000000000000, 0.9510565162951535312, 1.000000000000000000, 0.9510565162951535312, 1.000000000000000000, 0.9510565162951535312, 1.000000000000000000, 0.9510565162951535312, 1.000000000000000000, 0.9510565162951535312, 1.000000000000000000, 0.9510565162951535312, 1.000000000000000000, 0.9510565162951535312, 1.000000000000000000, 0.9510565162951535312, 1.000000000000000000, 0.9510565162951535312, 1.000000000000000000, 0.9510565162951535312, 1.000000000000000000, 0.9510565162951535312, 1.000000000000000000, 0.9510565162951535312, 1.000000000000000000, 0.9510565162951535312, 1.000000000000000000, 0.9510565162951535312, 1.000000000000000000, 0.9510565162951535312, 1.000000000000000000, 0.9510565162951535312, 1.000000000000000000, 0.9510565162951535312, 1.000000000000000000, 0.9510565162951535312, 1.000000000000000000, 0.9510565162951535312, 1.000000000000000000, 0.9510565162951535312, 1.000000000000000000, 0.9510565162951535312, 1.000000000000000000, 0.9510565162951535312, 1.000000000000000000, 0.9510565162951535312, 1.000000000000000000, 0.9510565162951535312, 1.000000000000000000, 0.9510565162951535312, 1.000000000000000000, 0.9510565162951535312, 1.000000000000000000, 0.9510565162951535312, 1.000000000000000000, 0.9510565162951535312, 1.000000000000000000, 0.9510565162951535312, 1.000000000000000000, 0.9510565162951535312, 1.000000000000000000, 0.9510565162951535312, 1.000000000000000000, 0.9510565162951535312, 1.000000000000000000, 0.9510565162951535312, 1.000000000000000000, 0.9510565162951535312, 1.000000000000000000, 0.9510565162951535312, 1.000000000000000000, 0.9510565162951535312, 1.000000000000000000, 0.9510565162951535312, 1.000000000000000000, 0.9510565162951535312, 1.000000000000000000, 0.9510565162951535312, 1.000000000000000000, 0.9510565162951535312, 1.000000000000000000, 0.9510565162951535312, 1.000000000000000000, 0.9510565162951535312, 1.000000000000000000, 0.9510565162951535312, 1.000000000000000000, 0.9510565162951535312, 1.000000000000000000, 0.9510565162951535312, 1.000000000000000000, 0.9510565162951535312, 1.000000000000000000, 0.9510565162951535312, 1.000000000000000000, 0.9510565162951535312, 1.000000000000000000, 0.9510565162951535312, 1.000000000000000000, 0.9510565162951535312, 1.000000000000000000, 0.9510565162951535312, 1.000000000000000000, 0.9510565162951535312, 1.000000000000000000, 0.9510565162951535312, 1.000000000000000000, 0.9510565162951535312, 1.000000000000000000, 0.9510565162951535312, 1.000000000000000000, 0.9510565162951535312, 1.000000000000000000, 0.9510565162951535312, 1.000000000000000000, 0.9510565162951535312, 1.000000000000000000, 0.9510565162951535312, 1.000000000000000000, 0.9510565162951535312, 1.000000000000000000, 0.9510565162951535312, 1.000000000000000000, 0.9510565162951535312, 1.000000000000000000, 0.9510565162951535312, 1.000000000000000000, 0.9510565162951535312, 1.000000000000000000, 0.9510565162951535312, 1.000000000000000000, 0.9510565162951535312, 1.000000000000000000, 0.9510565162951535312, 1.000000000000000000, 0.9510565162951535312, 1.000000000000000000, 0.9510565162951535312, 1.000000000000000000, 0.9510565162951535312, 1.000000000000000000, 0.9510565162951535312, 1.000000000000000000, 0.9510565162951535312, 1.000000000000000000, 0.9510565162951535312, 1.000000000000000000, 0.9510565162951535312, 1.000000000000000000, 0.9510565162951535312, 1.000000000000000000, 0.9510565162951535312, 1.000000000000000000, 0.9510565162951535312, 1.000000000000000000, 0.9510565162951535312, 1.000000000000000000, 0.9510565162951535312, 1.000000000000000000, 0.9510565162951535312, 1.000000000000000000, 0.9510565162951535312, 1.000000000000000000, 0.9510565162951535312, 1.000000000000000000, 0.9510565162951535312, 1.000000000000000000, 0.9510565162951535312, 1.000000000000000000, 0.9510565162951535312, 1.000000000000000000, 0.9510565162951535312, 1.000000000000000000, 0.9510565162951535312, 1.000000000000000000, 0.9510565162951535312, 1.000000000000000000, 0.9510565162951535312, 1.000000000000000000, 0.9510565162951535312, 1.000000000000000000, 0.9510565162951535312, 1.000000000000000000, 0.9510565162951535312, 1.000000000000000000, 0.9510565162951535312, 1.000000000000000000, 0.9510565162951535312, 1.000000000000000000, 0.9510565162951535312, 1.000000000000000000, 0.9510565162951535312, 1.000000000000000000, 0.9510565162951535312, 1.000000000000000000, 0.9510565162951535312, 1.000000000000000000, 0.9510565162951535312, 1.000000000000000000, 0.9510565162951535312, 1.000000000000000000, 0.9510565162951535312, 1.000000000000000000, 0.9510565162951535312, 1.000000000000000000, 0.9510565162951535312, 1.000000000000000000, 0.9510565162951535312, 1.000000000000000000, 0.9510565162951535312, 1.000000000000000000, 0.9510565162951535312, 1.000000000000000000, 0.9510565162951535312, 1.000000000000000000, 0.9510565162951535312, 1.000000000000000000, 0.9510565162951535312, 1.000000000000000000, 0.9510565162951535312, 1.000000000000000000, 0.9510565162951535312, 1.000000000000000000, 0.9510565162951535312, 1.000000000000000000, 0.9510565162951535312, 1.000000000000000000, 0.9510565162951535312, 1.000000000000000000, 0.9510565162951535312, 1.000000000000000000, 0.9510565162951535312, 1.000000000000000000, 0.9510565162951535312, 1.000000000000000000, 0.9510565162951535312, 1.000000000000000000, 0.9510565162951535312, 1.000000000000000000, 0.9510565162951535312, 1.000000000000000000, 0.9510565162951535312, 1.000000000000000000, 0.9510565162951535312, 1.000000000000000000, 0.9510565162951535312, 1.000000000000000000, 0.9510565162951535312, 1.000000000000000000, 0.9510565162951535312, 1.000000000000000000, 0.9510565162951535312, 1.000000000000000000, 0.9510565162951535312, 1.000000000000000000, 0.9510565162951535312, 1.000000000000000000, 0.9510565162951535312, 1.000000000000000000, 0.9510565162951535312, 1.000000000000000000, 0.9510565162951535312, 1.000000000000000000, 0.9510565162951535312, 1.000000000000000000, 0.9510565162951535312, 1.000000000000000000, 0.9510565162951535312, 1.000000000000000000, 0.9510565162951535312, 1.000000000000000000, 0.9510565162951535312, 1.000000000000000000, 0.9510565162951535312, 1.000000000000000000, 0.9510565162951535312, 1.000000000000000000, 0.9510565162951535312, 1.000000000000000000, 0.9510565162951535312, 1.000000000000000000, 0.9510565162951535312, 1.000000000000000000, 0.9510565162951535312, 1.000000000000000000, 0.9510565162951535312, 1.000000000000000000, 0.9510565162951535312, 1.000000000000000000, 0.9510565162951535312, 1.000000000000000000, 0.9510565162951535312, 1.000000000000000000, 0.9510565162951535312, 1.000000000000000000, 0.9510565162951535312, 1.000000000000000000, 0.9510565162951535312, 1.000000000000000000, 0.9510565162951535312, 1.000000000000000000, 0.9510565162951535312, 1.000000000000000000, 0.9510565162951535312, 1.000000000000000000, 0.9510565162951535312, 1.000000000000000000, 0.9510565162951535312, 1.000000000000000000, 0.9510565162951535312, 1.000000000000000000, 0.9510565162951535312, 1.000000000000000000, 0.9510565162951535312, 1.000000000000000000, 0.9510565162951535312, 1.000000000000000000, 0.9510565162951535312, 1.000000000000000000, 0.9510565162951535312, 1.000000000000000000, 0.9510565162951535312, 1.000000000000000000, 0.9510565162951535312, 1.000000000000000000, 0.9510565162951535312, 1.000000000000000000, 0.9510565162951535312, 1.000000000000000000, 0.9510565162951535312, 1.000000000000000000, 0.9510565162951535312, 1.000000000000000000, 0.9510565162951535312, 1.000000000000000000, 0.9510565162951535312, 1.000000000000000000, 0.9510565162951535312, 1.000000000000000000, 0.9510565162951535312, 1.000000000000000000, 0.9510565162951535312, 1.000000000000000000, 0.9510565162951535312, 1.000000000000000000, 0.9510565162951535312, 1.000000000000000000, 0.9510565162951535312, 1.000000000000000000, 0.9510565162951535312, 1.000000000000000000, 0.9510565162951535312, 1.000000000000000000, 0.9510565162951535312, 1.000000000000000000, 0.9510565162951535312, 1.000000000000000000, 0.9510565162951535312, 1.000000000000000000, 0.9510565162951535312, 1.000000000000000000, 0.9510565162951535312, 1.000000000000000000, 0.9510565162951535312, 1.000000000000000000, 0.9510565162951535312, 1.000000000000000000, 0.9510565162951535312, 1.000000000000000000, 0.9510565162951535312, 1.000000000000000000, 0.9510565162951535312, 1.000000000000000000, 0.9510565162951535312, 1.000000000000000000, 0.9510565162951535312, 1.000000000000000000, 0.9510565162951535312, 1.000000000000000000, 0.9510565162951535312, 1.000000000000000000, 0.9510565162951535312, 1.000000000000000000, 0.9510565162951535312, 1.000000000000000000, 0.9510565162951535312, 1.000000000000000000, 0.9510565162951535312, 1.000000000000000000, 0.9510565162951535312, 1.000000000000000000, 0.9510565162951535312, 1.000000000000000000, 0.9510565162951535312, 1.000000000000000000, 0.9510565162951535312, 1.000000000000000000, 0.9510565162951535312, 1.000000000000000000, 0.9510565162951535312, 1.000000000000000000, 0.9510565162951535312, 1.000000000000000000, 0.9510565162951535312, 1.000000000000000000, 0.9510565162951535312, 1.000000000000000000, 0.9510565162951535312, 1.000000000000000000, 0.9510565162951535312, 1.000000000000000000, 0.9510565162951535312, 1.000000000000000000, 0.9510565162951535312, 1.000000000000000000, 0.9510565162951535312, 1.000000000000000000, 0.9510565162951535312, 1.000000000000000000, 0.9510565162951535312, 1.000000000000000000, 0.9510565162951535312, 1.000000000000000000, 0.9510565162951535312, 1.000000000000000000, 0.9510565162951535312, 1.000000000000000000, 0.9510565162951535312, 1.000000000000000000, 0.9510565162951535312, 1.000000000000000000, 0.9510565162951535312, 1.000000000000000000, 0.9510565162951535312, 1.000000000000000000, 0.9510565162951535312, 1.000000000000000000, 0.9510565162951535312, 1.000000000000000000, 0.9510565162951535312, 1.000000000000000000, 0.9510565162951535312, 1.000000000000000000, 0.9510565162951535312, 1.000000000000000000, 0.9510565162951535312, 1.000000000000000000, 0.9510565162951535312, 1.000000000000000000, 0.9510565162951535312, 1.000000000000000000, 0.9510565162951535312, 1.000000000000000000, 0.9510565162951535312, 1.000000000000000000, 0.9510565162951535312, 1.000000000000000000, 0.9510565162951535312, 1.000000000000000000, 0.9510565162951535312, 1.000000000000000000, 0.9510565162951535312, 1.000000000000000000, 0.9510565162951535312, 1.000000000000000000, 0.9510565162951535312, 1.000000000000000000, 0.9510565162951535312, 1.000000000000000000, 0.9510565162951535312, 1.000000000000000000, 0.9510565162951535312, 1.000000000000000000, 0.9510565162951535312, 1.000000000000000000, 0.9510565162951535312, 1.000000000000000000, 0.9510565162951535312, 1.000000000000000000, 0.9510565162951535312, 1.000000000000000000, 0.9510565162951535312, 1.000000000000000000, 0.9510565162951535312, 1.000000000000000000, 0.9510565162951535312, 1.000000000000000000, 0.9510565162951535312, 1.000000000000000000, 0.9510565162951535312, 1.000000000000000000, 0.9510565162951535312, 1.000000000000000000, 0.9510565162951535312, 1.000000000000000000, 0.9510565162951535312, 1.000000000000000000, 0.9510565162951535312, 1.000000000000000000, 0.9510565162951535312, 1.000000000000000000, 0.9510565162951535312, 1.000000000000000000, 0.9510565162951535312, 1.000000000000000000, 0.9510565162951535312, 1.000000000000000000, 0.9510565162951535312, 1.000000000000000000, 0.9510565162951535312, 1.000000000000000000, 0.9510565162951535312, 1.000000000000000000, 0.9510565162951535312, 1.000000000000000000, 0.9510565162951535312, 1.000000000000000000, 0.9510565162951535312, 1.000000000000000000, 0.9510565162951535312, 1.000000000000000000, 0.9510565162951535312, 1.000000000000000000, 0.9510565162951535312, 1.000000000000000000, 0.9510565162951535312, 1.000000000000000000, 0.9510565162951535312, 1.000000000000000000, 0.9510565162951535312, 1.000000000000000000, 0.9510565162951535312, 1.000000000000000000, 0.9510565162951535312, 1.000000000000000000, 0.9510565162951535312, 1.000000000000000000, 0.9510565162951535312, 1.000000000000000000, 0.9510565162951535312, 1.000000000000000000, 0.9510565162951535312, 1.000000000000000000, 0.9510565162951535312, 1.000000000000000000, 0.9510565162951535312, 1.000000000000000000, 0.9510565162951535312, 1.000000000000000000, 0.9510565162951535312, 1.000000000000000000, 0.9510565162951535312, 1.000000000000000000, 0.9510565162951535312, 1.000000000000000000, 0.9510565162951535312, 1.000000000000000000, 0.9510565162951535312, 1.000000000000000000, 0.9510565162951535312, 1.000000000000000000, 0.9510565162951535312, 1.000000000000000000, 0.9510565162951535312, 1.000000000000000000, 0.9510565162951535312, 1.000000000000000000, 0.9510565162951535312, 1.000000000000000000, 0.9510565162951535312, 1.000000000000000000, 0.9510565162951535312, 1.000000000000000000, 0.9510565162951535312, 1.000000000000000000, 0.9510565162951535312, 1.000000000000000000, 0.9510565162951535312, 1.000000000000000000, 0.9510565162951535312, 1.000000000000000000, 0.9510565162951535312, 1.000000000000000000) ) ) 
 REPRESENTATION_ITEM ( '' )  SURFACE ( )  );
#23830=CARTESIAN_POINT ( 'NONE',  ( 20.08610463437157279, 71.29999999999999716, -27.64615127144129758 ) ) ;
#23831=CARTESIAN_POINT ( 'NONE',  ( -20.75514604977248112, 17.42500000273117777, 28.56700777964554661 ) ) ;
#23835=CARTESIAN_POINT ( 'NONE',  ( -26.29305231718579350, 36.30000000546239391, -19.10302069950537884 ) ) ;
#23840=CARTESIAN_POINT ( 'NONE',  ( -27.16883889988624290, 64.92500000273119554, -19.73931689729374028 ) ) ;
#23844=CARTESIAN_POINT ( 'NONE',  ( -10.37757302488623701, 7.525000002731194293, 31.93888565452638417 ) ) ;
#23845=ORIENTED_EDGE ( 'NONE', *, *, #11354, .F. ) ;
#23854=CARTESIAN_POINT ( 'NONE',  ( -32.50000000000000000, 20.00000000000000355, 0.000000000000000000 ) ) ;
#23865=CARTESIAN_POINT ( 'NONE',  ( 0.3323905815834450328, 66.99999999999998579, -33.36564663192542213 ) ) ;
#23867=CARTESIAN_POINT ( 'NONE',  ( -20.75514604977248112, 37.42500000273118843, 28.56700777964554661 ) ) ;
#23869=CARTESIAN_POINT ( 'NONE',  ( 27.16883889988624290, 52.17500000273118843, 19.73931689729373673 ) ) ;
#23872=CARTESIAN_POINT ( 'NONE',  ( -26.29305231718579350, 52.30000000546237970, -19.10302069950537884 ) ) ;
#23877=CARTESIAN_POINT ( 'NONE',  ( -33.58253175000000113, 27.37500000273117351, 0.000000000000000000 ) ) ;
#23881=CARTESIAN_POINT ( 'NONE',  ( -10.04305231718578462, 14.90000000546236336, 30.90933677959249337 ) ) ;
#23891=CARTESIAN_POINT ( 'NONE',  ( -20.75514604977248823, 62.82500000273119412, -28.56700777964554305 ) ) ;
#23896=CARTESIAN_POINT ( 'NONE',  ( -32.50000000000000000, 66.40000000546238823, -10.55989012756945300 ) ) ;
#23901=CARTESIAN_POINT ( 'NONE',  ( -20.75514604977248823, 67.07500000273118701, -28.56700777964554305 ) ) ;
#23906=CARTESIAN_POINT ( 'NONE',  ( -27.16883889988623935, 51.32500000273120122, 19.73931689729374739 ) ) ;
#23907=CARTESIAN_POINT ( 'NONE',  ( -33.58253175000000113, 15.27500000273118985, -10.91162601494193218 ) ) ;
#23908=CARTESIAN_POINT ( 'NONE',  ( -27.16883889988624290, 5.175000002731189319, -19.73931689729374028 ) ) ;
#23912=CARTESIAN_POINT ( 'NONE',  ( -26.29305231718578995, 74.70000000546238539, 19.10302069950538595 ) ) ;
#23913=CARTESIAN_POINT ( 'NONE',  ( 33.24513298742186862, 52.00000000000000000, -2.427281437204658943 ) ) ;
#23920=CARTESIAN_POINT ( 'NONE',  ( -10.37757302488624411, 48.97500000273117848, -31.93888565452638417 ) ) ;
#23927=CARTESIAN_POINT ( 'NONE',  ( 6.486482029760649416E-15, 19.62500000273116996, 35.31076352940723240 ) ) ;
#23939=LINE ( 'NONE', #408, #29475 ) ;
#23942=CARTESIAN_POINT ( 'NONE',  ( 32.50000000000000000, 15.00000000000000000, -3.980102097228898626E-15 ) ) ;
#23948=CARTESIAN_POINT ( 'NONE',  ( -33.58253175000000113, 75.22500000273119269, 10.91162601494193929 ) ) ;
#23949=CARTESIAN_POINT ( 'NONE',  ( -10.37757302488624411, 34.97500000273119980, -31.93888565452638417 ) ) ;
#23954=CARTESIAN_POINT ( 'NONE',  ( -32.50000000000000000, 53.90000000000001279, -10.55989012756945478 ) ) ;
#23960=ORIENTED_EDGE ( 'NONE', *, *, #21402, .T. ) ;
#23961=CARTESIAN_POINT ( 'NONE',  ( -33.58253175000000113, 65.47500000273117848, 10.91162601494193929 ) ) ;
#23966=CARTESIAN_POINT ( 'NONE',  ( -33.58253175000000113, 39.22500000273119269, 10.91162601494193929 ) ) ;
#23970=CARTESIAN_POINT ( 'NONE',  ( 10.04305231718579705, 1.100000005462370423, 30.90933677959248982 ) ) ;
#23988=CARTESIAN_POINT ( 'NONE',  ( -33.58253175000000113, 57.27500000273120406, -10.91162601494193218 ) ) ;
#23995=CARTESIAN_POINT ( 'NONE',  ( -32.50000000000000000, 75.89999999999996305, -10.55989012756945478 ) ) ;
#23996=CARTESIAN_POINT ( 'NONE',  ( -2.162160676586881955E-15, 10.62500000273119127, -35.31076352940723240 ) ) ;
#24004=CARTESIAN_POINT ( 'NONE',  ( -33.58253175000000113, 61.02500000273118985, -10.91162601494193218 ) ) ;
#24008=CARTESIAN_POINT ( 'NONE',  ( 10.37757302488624056, 6.525000002731193405, -31.93888565452638417 ) ) ;
#24020=CARTESIAN_POINT ( 'NONE',  ( -26.29305231718579350, 25.80000000000000426, -19.10302069950537884 ) ) ;
#24025=CARTESIAN_POINT ( 'NONE',  ( -33.37605761044780905, 67.00000000000000000, -0.2721180500505538391 ) ) ;
#24033=CARTESIAN_POINT ( 'NONE',  ( -1.683996601885078048, 52.00000000000000000, 33.30202823065787499 ) ) ;
#24035=CARTESIAN_POINT ( 'NONE',  ( -10.37757302488623701, 31.52500000273118630, 31.93888565452638417 ) ) ;
#24036=CARTESIAN_POINT ( 'NONE',  ( 5.147494310547426899, 65.44874571845315359, -32.50000000000000000 ) ) ;
#24040=CARTESIAN_POINT ( 'NONE',  ( 32.50000000000000711, 53.40000000546238823, 10.55989012756945122 ) ) ;
#24047=ORIENTED_EDGE ( 'NONE', *, *, #4410, .T. ) ;
#24049=CARTESIAN_POINT ( 'NONE',  ( 20.08610463437158344, 19.20000000546236052, 27.64615127144129403 ) ) ;
#24061=CARTESIAN_POINT ( 'NONE',  ( 33.58253175000000823, 58.02500000273117564, 10.91162601494192685 ) ) ;
#24072=CARTESIAN_POINT ( 'NONE',  ( -33.58253175000000113, 69.27500000273116143, -10.91162601494193218 ) ) ;
#24076=CARTESIAN_POINT ( 'NONE',  ( 33.58253175000000113, 52.12500000273119838, -4.112674001490185761E-15 ) ) ;
#24077=CARTESIAN_POINT ( 'NONE',  ( 33.58253175000000113, 10.37500000273118594, -4.112674001490185761E-15 ) ) ;
#24078=CARTESIAN_POINT ( 'NONE',  ( 6.486482029760649416E-15, 3.875000002731187720, 35.31076352940723240 ) ) ;
#24082=CARTESIAN_POINT ( 'NONE',  ( -10.04305231718578462, 72.90000000546238823, 30.90933677959249337 ) ) ;
#24089=CARTESIAN_POINT ( 'NONE',  ( -33.58253175000000113, 45.37500000273119127, 0.000000000000000000 ) ) ;
#24094=CARTESIAN_POINT ( 'NONE',  ( 33.58253175000000823, 20.02500000273118275, 10.91162601494192863 ) ) ;
#24108=CARTESIAN_POINT ( 'NONE',  ( 26.29305231718578995, 7.199999999999998401, -19.10302069950538240 ) ) ;
#24115=CARTESIAN_POINT ( 'NONE',  ( 33.58253175000000113, 74.22500000273119269, -10.91162601494193751 ) ) ;
#24116=CARTESIAN_POINT ( 'NONE',  ( -20.75514604977248112, 31.67500000273119909, 28.56700777964554661 ) ) ;
#24122=CARTESIAN_POINT ( 'NONE',  ( 32.50000000000000000, 55.09999999999998010, -10.55989012756945833 ) ) ;
#24127=CARTESIAN_POINT ( 'NONE',  ( -20.75514604977248112, 67.67500000273116711, 28.56700777964554661 ) ) ;
#24132=CARTESIAN_POINT ( 'NONE',  ( -20.75514604977248823, 34.82500000273118701, -28.56700777964554305 ) ) ;
#24153=CARTESIAN_POINT ( 'NONE',  ( -10.37757302488624411, 54.97500000273118559, -31.93888565452638417 ) ) ;
#24160=CARTESIAN_POINT ( 'NONE',  ( -26.29305231718579350, 71.80000000000001137, -19.10302069950537884 ) ) ;
#24161=CARTESIAN_POINT ( 'NONE',  ( 33.58253175000000113, 10.12500000273118594, -4.112674001490185761E-15 ) ) ;
#24169=CARTESIAN_POINT ( 'NONE',  ( 33.58253175000000823, 58.02500000273117564, 10.91162601494192863 ) ) ;
#24174=CARTESIAN_POINT ( 'NONE',  ( 27.16883889988624290, 1.925000002731186433, 19.73931689729373673 ) ) ;
#24183=CARTESIAN_POINT ( 'NONE',  ( -20.08610463437157989, 25.70000000000000284, -27.64615127144129758 ) ) ;
#24198=CARTESIAN_POINT ( 'NONE',  ( 10.37757302488624056, 26.52500000273118275, -31.93888565452638417 ) ) ;
#24200=CARTESIAN_POINT ( 'NONE',  ( 5.147494310547380714, 64.55125428154684641, 32.50000000000002132 ) ) ;
#24202=CARTESIAN_POINT ( 'NONE',  ( 5.779280353836490358E-15, 61.00000000546238255, 32.49999999999999289 ) ) ;
#24204=CARTESIAN_POINT ( 'NONE',  ( 20.08610463437158344, 49.20000000546237828, 27.64615127144129403 ) ) ;
#24208=CARTESIAN_POINT ( 'NONE',  ( 6.486482029760649416E-15, 73.62500000273118417, 35.31076352940723240 ) ) ;
#24214=CARTESIAN_POINT ( 'NONE',  ( 26.29305231718579350, 17.30000000546237615, 19.10302069950537529 ) ) ;
#24222=DIRECTION ( 'NONE',  ( 0.000000000000000000, 0.000000000000000000, 1.000000000000000000 ) ) ;
#24232=CARTESIAN_POINT ( 'NONE',  ( -40.00000000000000711, 52.00000000000000711, -23.09401076758504345 ) ) ;
#24233=CARTESIAN_POINT ( 'NONE',  ( -20.75514604977248823, 69.07500000273115859, -28.56700777964554305 ) ) ;
#24238=CARTESIAN_POINT ( 'NONE',  ( 20.75514604977248467, 44.42500000273120264, -28.56700777964554305 ) ) ;
#24239=CARTESIAN_POINT ( 'NONE',  ( 10.37757302488624767, 13.97500000273120513, 31.93888565452638417 ) ) ;
#24240=CARTESIAN_POINT ( 'NONE',  ( -33.58253175000000113, 61.37500000273120548, 0.000000000000000000 ) ) ;
#24244=CARTESIAN_POINT ( 'NONE',  ( 32.50000000000000000, 71.50000000546236834, -3.980102097228898626E-15 ) ) ;
#24252=CARTESIAN_POINT ( 'NONE',  ( 33.58253175000000113, 46.47500000273118559, -10.91162601494193751 ) ) ;
#24257=CARTESIAN_POINT ( 'NONE',  ( -20.75514604977248823, 16.82500000273120122, -28.56700777964554305 ) ) ;
#24258=EDGE_CURVE ( 'NONE', #33963, #52, #31699, .T. ) ;
#24260=ORIENTED_EDGE ( 'NONE', *, *, #32206, .F. ) ;
#24267=AXIS2_PLACEMENT_3D ( 'NONE', #24232, #19417, #32104 ) ;
#24274=CARTESIAN_POINT ( 'NONE',  ( 10.04305231718579705, 12.59999999999998543, 30.90933677959248982 ) ) ;
#24280=CARTESIAN_POINT ( 'NONE',  ( -20.75514604977248823, 64.82500000273120122, -28.56700777964554305 ) ) ;
#24281=CARTESIAN_POINT ( 'NONE',  ( 20.75514604977249178, 28.07500000273119412, 28.56700777964553950 ) ) ;
#24282=CARTESIAN_POINT ( 'NONE',  ( -20.75514604977248823, 17.07500000273119056, -28.56700777964554305 ) ) ;
#24289=VECTOR ( 'NONE', #7859, 1000.000000000000000 ) ;
#24290=CARTESIAN_POINT ( 'NONE',  ( 32.50000000000000000, 57.09999999999999432, -10.55989012756945833 ) ) ;
#24295=CARTESIAN_POINT ( 'NONE',  ( 33.58253175000000113, 68.47500000273119269, -10.91162601494193751 ) ) ;
#24300=CARTESIAN_POINT ( 'NONE',  ( -33.58253175000000113, 39.02500000273118985, -10.91162601494193218 ) ) ;
#24301=VERTEX_POINT ( 'NONE', #26223 ) ;
#24314=CARTESIAN_POINT ( 'NONE',  ( 20.08610463437157279, 53.80000000546237970, -27.64615127144129758 ) ) ;
#24320=CARTESIAN_POINT ( 'NONE',  ( -20.75514604977248112, 49.67500000273118133, 28.56700777964554661 ) ) ;
#24326=CARTESIAN_POINT ( 'NONE',  ( -2.092463501923844636E-15, 75.50000000000001421, -34.17252228774368916 ) ) ;
#24327=CARTESIAN_POINT ( 'NONE',  ( 27.16883889988623935, 8.325000002731188786, -19.73931689729374384 ) ) ;
#24338=CARTESIAN_POINT ( 'NONE',  ( 33.58253175000000113, 56.12500000273119838, -4.112674001490185761E-15 ) ) ;
#24353=CARTESIAN_POINT ( 'NONE',  ( 20.08610463437158344, 24.70000000000000284, 27.64615127144129403 ) ) ;
#24363=CARTESIAN_POINT ( 'NONE',  ( 32.15037667113031716, 67.00000000000000000, -5.379467130814792775 ) ) ;
#24364=CARTESIAN_POINT ( 'NONE',  ( -2.357955684373814975, 51.99999999999997868, 33.24972188832315823 ) ) ;
#24365=CARTESIAN_POINT ( 'NONE',  ( -33.58253175000000113, 27.22500000273119269, 10.91162601494193929 ) ) ;
#24366=CARTESIAN_POINT ( 'NONE',  ( 2.205017735002230837E-13, 56.00000000546238255, -32.50000000000000000 ) ) ;
#24370=CARTESIAN_POINT ( 'NONE',  ( 20.08610463437157279, 45.80000000546240102, -27.64615127144129758 ) ) ;
#24374=CARTESIAN_POINT ( 'NONE',  ( -33.58253175000000113, 73.22500000273117848, 10.91162601494193929 ) ) ;
#24380=CARTESIAN_POINT ( 'NONE',  ( 20.08610463437158344, 15.20000000546237118, 27.64615127144129403 ) ) ;
#24395=CARTESIAN_POINT ( 'NONE',  ( 20.75514604977248467, 70.67500000273118133, -28.56700777964554305 ) ) ;
#24400=CARTESIAN_POINT ( 'NONE',  ( 27.16883889988623935, 46.32500000273119412, -19.73931689729374384 ) ) ;
#24401=CARTESIAN_POINT ( 'NONE',  ( -20.75514604977248823, 11.07500000273119056, -28.56700777964554305 ) ) ;
#24402=CARTESIAN_POINT ( 'NONE',  ( -20.75514604977248112, 63.67500000273117422, 28.56700777964554661 ) ) ;
#24406=CARTESIAN_POINT ( 'NONE',  ( 20.08610463437158344, 69.20000000546235697, 27.64615127144129403 ) ) ;
#24412=CARTESIAN_POINT ( 'NONE',  ( -20.75514604977248823, 47.07500000273117990, -28.56700777964554305 ) ) ;
#24417=CARTESIAN_POINT ( 'NONE',  ( 33.58253175000000113, 20.22500000273117848, -10.91162601494193751 ) ) ;
#24427=VECTOR ( 'NONE', #31440, 1000.000000000000000 ) ;
#24432=CARTESIAN_POINT ( 'NONE',  ( 20.08610463437157279, 11.30000000000000604, -27.64615127144129758 ) ) ;
#24438=CARTESIAN_POINT ( 'NONE',  ( 6.486482029760649416E-15, 63.62500000273117706, 35.31076352940723240 ) ) ;
#24439=CARTESIAN_POINT ( 'NONE',  ( 6.486482029760649416E-15, 31.87500000273119127, 35.31076352940723240 ) ) ;
#24440=CARTESIAN_POINT ( 'NONE',  ( -33.58253175000000113, 19.27500000273117919, -10.91162601494193218 ) ) ;
#24447=CARTESIAN_POINT ( 'NONE',  ( -32.50000000000000000, 46.09999999999999432, 10.55989012756946366 ) ) ;
#24452=CARTESIAN_POINT ( 'NONE',  ( -10.37757302488624411, 68.97500000273119269, -31.93888565452638417 ) ) ;
#24458=CARTESIAN_POINT ( 'NONE',  ( 33.58253175000000823, 38.02500000273117564, 10.91162601494192863 ) ) ;
#24463=CARTESIAN_POINT ( 'NONE',  ( -32.50000000000000000, 0.6000000054623827461, 10.55989012756946366 ) ) ;
#24476=CARTESIAN_POINT ( 'NONE',  ( -26.29305231718578995, 54.70000000546236407, 19.10302069950538595 ) ) ;
#24480=CARTESIAN_POINT ( 'NONE',  ( 27.16883889988623935, 50.57500000273117280, -19.73931689729374384 ) ) ;
#24487=CARTESIAN_POINT ( 'NONE',  ( 26.29305231718578995, 75.20000000000000284, -19.10302069950538240 ) ) ;
#24488=CARTESIAN_POINT ( 'NONE',  ( 20.75514604977249178, 11.82500000273118346, 28.56700777964553950 ) ) ;
#24497=CARTESIAN_POINT ( 'NONE',  ( 33.58253175000000823, 54.02500000273118275, 10.91162601494192863 ) ) ;
#24498=CARTESIAN_POINT ( 'NONE',  ( -20.75514604977248823, 31.07500000273118701, -28.56700777964554305 ) ) ;
#24508=CARTESIAN_POINT ( 'NONE',  ( 3.980102097228898626E-15, 52.00000000000000711, -32.50000000000000000 ) ) ;
#24526=CARTESIAN_POINT ( 'NONE',  ( -12.18942006770533837, 51.99999999999998579, 30.86762708970428193 ) ) ;
#24527=CARTESIAN_POINT ( 'NONE',  ( 20.75514604977248467, 28.42500000273118133, -28.56700777964554305 ) ) ;
#24529=CARTESIAN_POINT ( 'NONE',  ( 20.08610463437158344, 60.70000000000000284, 27.64615127144129403 ) ) ;
#24531=CARTESIAN_POINT ( 'NONE',  ( 26.29305231718579350, 51.30000000546237970, 19.10302069950537529 ) ) ;
#24533=CARTESIAN_POINT ( 'NONE',  ( -20.08610463437156923, 58.80000000546239391, 27.64615127144130113 ) ) ;
#24535=CARTESIAN_POINT ( 'NONE',  ( 10.37757302488624767, 77.72500000273117848, 31.93888565452638417 ) ) ;
#24538=ORIENTED_EDGE ( 'NONE', *, *, #24946, .F. ) ;
#24540=CARTESIAN_POINT ( 'NONE',  ( 26.29305231718578995, 13.70000000546238361, -19.10302069950538240 ) ) ;
#24547=CARTESIAN_POINT ( 'NONE',  ( -20.08610463437157989, 62.20000000546237118, -27.64615127144129758 ) ) ;
#24549=CARTESIAN_POINT ( 'NONE',  ( -32.50000000000000000, 35.90000000000000568, -10.55989012756945478 ) ) ;
#24557=CARTESIAN_POINT ( 'NONE',  ( 33.58253175000000823, 66.27500000273118985, 10.91162601494192863 ) ) ;
#24563=CARTESIAN_POINT ( 'NONE',  ( 20.75514604977248467, 50.42500000273118843, -28.56700777964554305 ) ) ;
#24564=CARTESIAN_POINT ( 'NONE',  ( 6.486482029760649416E-15, 13.87500000273117529, 35.31076352940723240 ) ) ;
#24565=CARTESIAN_POINT ( 'NONE',  ( 20.75514604977248467, 60.67500000273118133, -28.56700777964554305 ) ) ;
#24570=CARTESIAN_POINT ( 'NONE',  ( 6.277390505771533514E-15, 67.00000000546236834, 34.17252228774368916 ) ) ;
#24576=CARTESIAN_POINT ( 'NONE',  ( 33.58253175000000113, 38.37500000273118417, -4.112674001490185761E-15 ) ) ;
#24579=CARTESIAN_POINT ( 'NONE',  ( 32.50000000000000711, 27.40000000546239534, 10.55989012756945122 ) ) ;
#24581=CARTESIAN_POINT ( 'NONE',  ( 20.75514604977248467, 18.42500000273117422, -28.56700777964554305 ) ) ;
#24583=ORIENTED_EDGE ( 'NONE', *, *, #14595, .F. ) ;
#24596=CARTESIAN_POINT ( 'NONE',  ( 32.50000000000000000, 12.99999999999999822, -3.980102097228898626E-15 ) ) ;
#24602=CARTESIAN_POINT ( 'NONE',  ( -10.37757302488623701, 69.52500000273118985, 31.93888565452638417 ) ) ;
#24603=CARTESIAN_POINT ( 'NONE',  ( -27.16883889988624290, 27.17500000273119554, -19.73931689729374028 ) ) ;
#24604=CARTESIAN_POINT ( 'NONE',  ( -27.16883889988624290, 15.17500000273118488, -19.73931689729374028 ) ) ;
#24610=CARTESIAN_POINT ( 'NONE',  ( -26.29305231718579350, 49.79999999999999716, -19.10302069950537884 ) ) ;
#24611=CARTESIAN_POINT ( 'NONE',  ( 26.29305231718578995, 57.70000000546237118, -19.10302069950538240 ) ) ;
#24615=CARTESIAN_POINT ( 'NONE',  ( 27.16883889988624290, 64.17500000273116711, 19.73931689729373673 ) ) ;
#24620=CARTESIAN_POINT ( 'NONE',  ( 33.58253175000000113, 40.12500000273118417, -4.112674001490185761E-15 ) ) ;
#24640=CARTESIAN_POINT ( 'NONE',  ( -33.58253175000000113, 51.37500000273119127, 0.000000000000000000 ) ) ;
#24646=CARTESIAN_POINT ( 'NONE',  ( -26.29305231718579350, 63.80000000000001137, -19.10302069950537884 ) ) ;
#24647=CARTESIAN_POINT ( 'NONE',  ( -33.58253175000000113, 7.125000002731182391, 0.000000000000000000 ) ) ;
#24659=CARTESIAN_POINT ( 'NONE',  ( -27.16883889988623935, 59.32500000273120833, 19.73931689729374739 ) ) ;
#24660=CARTESIAN_POINT ( 'NONE',  ( -33.58253175000000113, 27.27500000273119340, -10.91162601494193218 ) ) ;
#24674=CARTESIAN_POINT ( 'NONE',  ( 20.75514604977248467, 56.42500000273120264, -28.56700777964554305 ) ) ;
#24690=CARTESIAN_POINT ( 'NONE',  ( 10.37757302488624767, 29.72500000273119269, 31.93888565452638417 ) ) ;
#24695=CARTESIAN_POINT ( 'NONE',  ( -32.50000000000000000, 48.50000000546238255, 0.000000000000000000 ) ) ;
#24696=CARTESIAN_POINT ( 'NONE',  ( -5.147494310547430452, 58.05125428700921475, -32.49999999999999289 ) ) ;
#24699=CARTESIAN_POINT ( 'NONE',  ( 27.16883889988623935, 72.32500000273118701, -19.73931689729374384 ) ) ;
#24704=CARTESIAN_POINT ( 'NONE',  ( 26.29305231718578995, 11.70000000546238184, -19.10302069950538240 ) ) ;
#24711=CARTESIAN_POINT ( 'NONE',  ( -10.04305231718578462, 62.90000000546238113, 30.90933677959249337 ) ) ;
#24714=CARTESIAN_POINT ( 'NONE',  ( 26.29305231718579350, 34.79999999999998295, 19.10302069950537529 ) ) ;
#24723=CARTESIAN_POINT ( 'NONE',  ( -33.58253175000000113, 63.37500000273120548, 0.000000000000000000 ) ) ;
#24728=CARTESIAN_POINT ( 'NONE',  ( 6.486482029760649416E-15, 47.62500000273118417, 35.31076352940723240 ) ) ;
#24729=CARTESIAN_POINT ( 'NONE',  ( 10.37757302488624767, 7.975000002731199800, 31.93888565452638417 ) ) ;
#24730=CARTESIAN_POINT ( 'NONE',  ( 27.16883889988624290, 64.17500000273116711, 19.73931689729373673 ) ) ;
#24734=CARTESIAN_POINT ( 'NONE',  ( 26.29305231718579350, 65.30000000546236549, 19.10302069950537529 ) ) ;
#24740=CARTESIAN_POINT ( 'NONE',  ( -20.75514604977248112, 43.67500000273119554, 28.56700777964554661 ) ) ;
#24743=CARTESIAN_POINT ( 'NONE',  ( -10.04305231718579172, 30.10000000546238397, -30.90933677959248982 ) ) ;
#24744=VERTEX_POINT ( 'NONE', #7127 ) ;
#24747=ORIENTED_EDGE ( 'NONE', *, *, #12800, .T. ) ;
#24759=CARTESIAN_POINT ( 'NONE',  ( 5.779280353836490358E-15, 56.49999999999998579, 32.49999999999999289 ) ) ;
#24761=CARTESIAN_POINT ( 'NONE',  ( -10.04305231718579172, 7.599999999999981881, -30.90933677959248982 ) ) ;
#24764=CARTESIAN_POINT ( 'NONE',  ( 0.000000000000000000, 52.00000000000000711, 32.50000000000000000 ) ) ;
#24766=CARTESIAN_POINT ( 'NONE',  ( 33.58253175000000823, 66.02500000273118985, 10.91162601494192863 ) ) ;
#24767=CARTESIAN_POINT ( 'NONE',  ( 33.58253175000000113, 32.37500000273117706, -4.112674001490185761E-15 ) ) ;
#24768=CARTESIAN_POINT ( 'NONE',  ( 10.37757302488624767, 13.97500000273120513, 31.93888565452638417 ) ) ;
#24774=CARTESIAN_POINT ( 'NONE',  ( -20.08610463437157989, 45.69999999999998863, -27.64615127144129758 ) ) ;
#24775=CARTESIAN_POINT ( 'NONE',  ( 32.50000000000000000, 57.50000000546238965, -3.980102097228898626E-15 ) ) ;
#24779=CARTESIAN_POINT ( 'NONE',  ( -27.16883889988623935, 59.57500000273117990, 19.73931689729374739 ) ) ;
#24781=AXIS2_PLACEMENT_3D ( 'NONE', #29299, #5799, #16608 ) ;
#24785=CARTESIAN_POINT ( 'NONE',  ( 33.58253175000000113, 28.12500000273120193, -4.112674001490185761E-15 ) ) ;
#24802=CARTESIAN_POINT ( 'NONE',  ( 5.147494310547426899, 53.94874572391552903, -32.50000000000000000 ) ) ;
#24808=CARTESIAN_POINT ( 'NONE',  ( 20.75514604977248467, 50.67500000273117422, -28.56700777964554305 ) ) ;
#24815=CARTESIAN_POINT ( 'NONE',  ( 32.50000000000000000, 64.99999999999998579, -3.980102097228898626E-15 ) ) ;
#24824=CARTESIAN_POINT ( 'NONE',  ( -20.75514604977248823, 54.82500000273118701, -28.56700777964554305 ) ) ;
#24825=CARTESIAN_POINT ( 'NONE',  ( -10.37757302488624411, 30.97500000273119269, -31.93888565452638417 ) ) ;
#24831=AXIS2_PLACEMENT_3D ( 'NONE', #28089, #12474, #10072 ) ;
#24840=CARTESIAN_POINT ( 'NONE',  ( 33.58253175000000113, 56.12500000273119838, -4.112674001490185761E-15 ) ) ;
#24855=CARTESIAN_POINT ( 'NONE',  ( 20.75514604977249178, 21.82500000273119056, 28.56700777964553950 ) ) ;
#24856=LINE ( 'NONE', #1508, #15500 ) ;
#24857=CARTESIAN_POINT ( 'NONE',  ( 32.50000000000000000, 53.00000000000000711, -3.980102097228898626E-15 ) ) ;
#24861=CARTESIAN_POINT ( 'NONE',  ( 26.29305231718578995, 45.70000000546238539, -19.10302069950538240 ) ) ;
#24865=CARTESIAN_POINT ( 'NONE',  ( 10.37757302488624767, 73.72500000273117848, 31.93888565452638417 ) ) ;
#24870=CARTESIAN_POINT ( 'NONE',  ( -20.08610463437156923, 8.800000005462383257, 27.64615127144130113 ) ) ;
#24878=CARTESIAN_POINT ( 'NONE',  ( -1.778240108872766143E-15, 62.00000000546238255, -32.49999999999999289 ) ) ;
#24881=CARTESIAN_POINT ( 'NONE',  ( 20.08610463437158344, 34.70000000000001705, 27.64615127144129403 ) ) ;
#24893=CARTESIAN_POINT ( 'NONE',  ( 20.75514604977249178, 47.82500000273117990, 28.56700777964553950 ) ) ;
#24894=CARTESIAN_POINT ( 'NONE',  ( -33.58253175000000113, 1.475000002731190474, 10.91162601494193929 ) ) ;
#24895=CARTESIAN_POINT ( 'NONE',  ( 27.16883889988624290, 62.17500000273119554, 19.73931689729373673 ) ) ;
#24900=CARTESIAN_POINT ( 'NONE',  ( -2.092463501923844636E-15, 70.00000000546239676, -34.17252228774368916 ) ) ;
#24908=CARTESIAN_POINT ( 'NONE',  ( 27.16883889988623935, 38.57500000273118701, -19.73931689729374384 ) ) ;
#24910=CARTESIAN_POINT ( 'NONE',  ( 10.04305231718579705, 33.10000000546238397, 30.90933677959248982 ) ) ;
#24911=VERTEX_POINT ( 'NONE', #33905 ) ;
#24919=CARTESIAN_POINT ( 'NONE',  ( -10.37757302488623701, 65.52500000273118985, 31.93888565452638417 ) ) ;
#24929=CARTESIAN_POINT ( 'NONE',  ( -20.08610463437156923, 4.299999999999994493, 27.64615127144130113 ) ) ;
#24934=CARTESIAN_POINT ( 'NONE',  ( -20.75514604977248823, 66.82500000273118701, -28.56700777964554305 ) ) ;
#24935=CARTESIAN_POINT ( 'NONE',  ( -27.16883889988623935, 25.57500000273120477, 19.73931689729374739 ) ) ;
#24936=CARTESIAN_POINT ( 'NONE',  ( 6.486482029760649416E-15, 19.87500000273119483, 35.31076352940723240 ) ) ;
#24942=CARTESIAN_POINT ( 'NONE',  ( -32.50000000000000000, 46.00000000000000000, 0.000000000000000000 ) ) ;
#24946=EDGE_CURVE ( 'NONE', #4618, #33963, #22710, .T. ) ;
#24949=CARTESIAN_POINT ( 'NONE',  ( 10.37757302488624056, 62.77500000273118985, -31.93888565452638417 ) ) ;
#24954=CARTESIAN_POINT ( 'NONE',  ( -33.58253175000000113, 31.02500000273118630, -10.91162601494193218 ) ) ;
#24977=CARTESIAN_POINT ( 'NONE',  ( -27.16883889988624290, 51.17500000273118843, -19.73931689729374028 ) ) ;
#24983=CARTESIAN_POINT ( 'NONE',  ( 10.04305231718578817, 65.40000000000000568, -30.90933677959249337 ) ) ;
#24984=AXIS2_PLACEMENT_3D ( 'NONE', #9657, #19621, #20137 ) ;
#24990=CARTESIAN_POINT ( 'NONE',  ( 20.75514604977248467, 78.67500000273116711, -28.56700777964554305 ) ) ;
#24995=CARTESIAN_POINT ( 'NONE',  ( -27.16883889988624290, 46.92500000273118133, -19.73931689729374028 ) ) ;
#24996=CARTESIAN_POINT ( 'NONE',  ( -27.16883889988624290, 25.17500000273119198, -19.73931689729374028 ) ) ;
#25008=CARTESIAN_POINT ( 'NONE',  ( -16.87750156402132617, 66.99999999999998579, -29.11635311643979662 ) ) ;
#25011=CARTESIAN_POINT ( 'NONE',  ( -2.162160676586882350E-15, 54.62500000273116996, -35.31076352940722529 ) ) ;
#25027=CARTESIAN_POINT ( 'NONE',  ( -10.37757302488624411, 18.72500000273118204, -31.93888565452638417 ) ) ;
#25032=CARTESIAN_POINT ( 'NONE',  ( -20.08610463437157989, 40.20000000546235697, -27.64615127144129758 ) ) ;
#25035=CARTESIAN_POINT ( 'NONE',  ( 10.37757302488624767, 65.97500000273119269, 31.93888565452638417 ) ) ;
#25038=CARTESIAN_POINT ( 'NONE',  ( 33.58253175000000823, 66.02500000273118985, 10.91162601494192863 ) ) ;
#25043=CARTESIAN_POINT ( 'NONE',  ( -26.29305231718578995, 8.700000005462380059, 19.10302069950538595 ) ) ;
#25053=CARTESIAN_POINT ( 'NONE',  ( -20.08610463437157989, 33.70000000000001705, -27.64615127144129758 ) ) ;
#25065=CARTESIAN_POINT ( 'NONE',  ( -2.162160676586881955E-15, 38.62500000273118417, -35.31076352940723240 ) ) ;
#25066=CARTESIAN_POINT ( 'NONE',  ( 27.16883889988623935, 6.575000002731187898, -19.73931689729374384 ) ) ;
#25067=CARTESIAN_POINT ( 'NONE',  ( -33.58253175000000113, 57.37500000273119838, 0.000000000000000000 ) ) ;
#25071=CARTESIAN_POINT ( 'NONE',  ( 32.50000000000000711, 69.40000000546235981, 10.55989012756945122 ) ) ;
#25076=CARTESIAN_POINT ( 'NONE',  ( -10.37757302488624411, 42.97500000273117848, -31.93888565452638417 ) ) ;
#25078=VERTEX_POINT ( 'NONE', #2317 ) ;
#25079=CARTESIAN_POINT ( 'NONE',  ( 10.04305231718579705, 29.10000000546238041, 30.90933677959248982 ) ) ;
#25080=ORIENTED_EDGE ( 'NONE', *, *, #16923, .F. ) ;
#25092=CARTESIAN_POINT ( 'NONE',  ( -27.16883889988623935, 65.32500000273118701, 19.73931689729374739 ) ) ;
#25104=CARTESIAN_POINT ( 'NONE',  ( 32.50000000000000711, 2.899999999999995470, 10.55989012756945122 ) ) ;
#25110=CARTESIAN_POINT ( 'NONE',  ( -2.162160676586881955E-15, 60.62500000273117706, -35.31076352940723240 ) ) ;
#25111=CARTESIAN_POINT ( 'NONE',  ( 10.37757302488624767, 21.97500000273118559, 31.93888565452638417 ) ) ;
#25112=CARTESIAN_POINT ( 'NONE',  ( -33.58253175000000113, 9.375000002731184168, 0.000000000000000000 ) ) ;
#25117=CARTESIAN_POINT ( 'NONE',  ( -2.092463501923844636E-15, 49.50000000000001421, -34.17252228774368916 ) ) ;
#25121=CARTESIAN_POINT ( 'NONE',  ( -20.75514604977248823, 61.07500000273119412, -28.56700777964554305 ) ) ;
#25126=CARTESIAN_POINT ( 'NONE',  ( 20.75514604977249178, 27.82500000273116925, 28.56700777964553950 ) ) ;
#25142=CARTESIAN_POINT ( 'NONE',  ( 10.04305231718579705, 54.59999999999999432, 30.90933677959248982 ) ) ;
#25149=CARTESIAN_POINT ( 'NONE',  ( 27.16883889988624290, 40.17500000273120975, 19.73931689729373673 ) ) ;
#25154=CARTESIAN_POINT ( 'NONE',  ( 32.50000000000000000, 69.09999999999998010, -10.55989012756945833 ) ) ;
#25159=CARTESIAN_POINT ( 'NONE',  ( 20.75514604977249178, 78.07500000273117280, 28.56700777964553950 ) ) ;
#25164=CARTESIAN_POINT ( 'NONE',  ( 33.58253175000000113, 52.12500000273119838, -4.112674001490185761E-15 ) ) ;
#25165=CARTESIAN_POINT ( 'NONE',  ( 27.16883889988624290, 20.17500000273118843, 19.73931689729373673 ) ) ;
#25184=EDGE_CURVE ( 'NONE', #33362, #26368, #8472, .T. ) ;
#25192=CARTESIAN_POINT ( 'NONE',  ( 5.485887633599118468E-07, 52.00000000000003553, -32.49999999999999289 ) ) ;
#25197=CARTESIAN_POINT ( 'NONE',  ( 33.58253175000000113, 20.12500000273119483, -4.112674001490185761E-15 ) ) ;
#25202=CARTESIAN_POINT ( 'NONE',  ( 6.277390505771533514E-15, 43.00000000546236123, 34.17252228774368916 ) ) ;
#25206=CARTESIAN_POINT ( 'NONE',  ( 6.486482029760648627E-15, 65.87500000273119838, 35.31076352940722529 ) ) ;
#25209=CARTESIAN_POINT ( 'NONE',  ( 6.486482029760649416E-15, 67.62500000273119838, 35.31076352940723240 ) ) ;
#25215=CARTESIAN_POINT ( 'NONE',  ( -27.16883889988624290, 12.92500000273118310, -19.73931689729374028 ) ) ;
#25223=CARTESIAN_POINT ( 'NONE',  ( -40.00000000000000711, 52.00000000000000711, -23.09401076758504345 ) ) ;
#25227=CARTESIAN_POINT ( 'NONE',  ( 10.04305231718578817, 35.39999999999999858, -30.90933677959249337 ) ) ;
#25241=CARTESIAN_POINT ( 'NONE',  ( -10.37757302488623701, 43.52500000273119696, 31.93888565452638417 ) ) ;
#25242=CARTESIAN_POINT ( 'NONE',  ( 10.37757302488624767, 1.975000002731180926, 31.93888565452638417 ) ) ;
#25243=CARTESIAN_POINT ( 'NONE',  ( -10.37757302488624411, 54.97500000273118559, -31.93888565452638417 ) ) ;
#25246=CARTESIAN_POINT ( 'NONE',  ( -32.50000000000000000, 58.60000000546236976, 10.55989012756946366 ) ) ;
#25252=CARTESIAN_POINT ( 'NONE',  ( -2.162160676586881955E-15, 42.87500000273119127, -35.31076352940723240 ) ) ;
#25256=CARTESIAN_POINT ( 'NONE',  ( -32.50000000000000000, 32.40000000546238113, -10.55989012756945478 ) ) ;
#25257=EDGE_LOOP ( 'NONE', ( #27346, #3854, #27664, #4574 ) ) ;
#25267=CARTESIAN_POINT ( 'NONE',  ( -20.75514604977248823, 64.82500000273120122, -28.56700777964554305 ) ) ;
#25277=CARTESIAN_POINT ( 'NONE',  ( -20.08610463437156923, 6.300000000000004263, 27.64615127144130113 ) ) ;
#25283=CARTESIAN_POINT ( 'NONE',  ( -33.58253175000000113, 63.12500000273117706, 0.000000000000000000 ) ) ;
#25284=CARTESIAN_POINT ( 'NONE',  ( -2.162160676586881955E-15, 22.87500000273118062, -35.31076352940723240 ) ) ;
#25285=CARTESIAN_POINT ( 'NONE',  ( -10.37757302488623701, 11.77500000273117031, 31.93888565452638417 ) ) ;
#25289=CARTESIAN_POINT ( 'NONE',  ( -2.162160676586881955E-15, 2.625000002731183724, -35.31076352940723240 ) ) ;
#25291=CARTESIAN_POINT ( 'NONE',  ( -32.50000000000000000, 43.90000000000001279, -10.55989012756945478 ) ) ;
#25299=CARTESIAN_POINT ( 'NONE',  ( 33.58253175000000823, 60.27500000273116143, 10.91162601494192863 ) ) ;
#25304=CARTESIAN_POINT ( 'NONE',  ( -10.37757302488624411, 28.72500000273118914, -31.93888565452638417 ) ) ;
#25317=CARTESIAN_POINT ( 'NONE',  ( 5.779280353836490358E-15, 54.49999999999999289, 32.49999999999999289 ) ) ;
#25318=CARTESIAN_POINT ( 'NONE',  ( -26.29305231718578995, 52.20000000000000995, 19.10302069950538595 ) ) ;
#25324=CARTESIAN_POINT ( 'NONE',  ( -10.37757302488623701, 45.77500000273119696, 31.93888565452638417 ) ) ;
#25327=CARTESIAN_POINT ( 'NONE',  ( -20.08610463437156923, 58.29999999999999716, 27.64615127144130113 ) ) ;
#25333=CARTESIAN_POINT ( 'NONE',  ( -10.37757302488624411, 78.97500000273120691, -31.93888565452638417 ) ) ;
#25339=CARTESIAN_POINT ( 'NONE',  ( 10.37757302488624056, 50.52500000273117564, -31.93888565452638417 ) ) ;
#25340=CARTESIAN_POINT ( 'NONE',  ( -27.16883889988623935, 21.57500000273120122, 19.73931689729374739 ) ) ;
#25363=CARTESIAN_POINT ( 'NONE',  ( -33.58253175000000113, 59.27500000273119696, -10.91162601494193218 ) ) ;
#25371=CARTESIAN_POINT ( 'NONE',  ( 10.37757302488624767, 21.72500000273118559, 31.93888565452638417 ) ) ;
#25373=CARTESIAN_POINT ( 'NONE',  ( -1.778240108872766143E-15, 53.50000000000000000, -32.49999999999999289 ) ) ;
#25376=CARTESIAN_POINT ( 'NONE',  ( 20.08610463437158344, 39.20000000546237118, 27.64615127144129403 ) ) ;
#25385=CARTESIAN_POINT ( 'NONE',  ( -33.58253175000000113, 67.22500000273117848, 10.91162601494193929 ) ) ;
#25391=CARTESIAN_POINT ( 'NONE',  ( -33.58253175000000113, 11.22500000273118559, 10.91162601494193929 ) ) ;
#25398=CARTESIAN_POINT ( 'NONE',  ( 5.779280353836490358E-15, 65.00000000546236834, 32.49999999999999289 ) ) ;
#25400=CARTESIAN_POINT ( 'NONE',  ( -32.50000000000000000, 28.00000000000001066, 0.000000000000000000 ) ) ;
#25415=CARTESIAN_POINT ( 'NONE',  ( 33.58253175000000823, 44.02500000273118275, 10.91162601494192863 ) ) ;
#25416=CARTESIAN_POINT ( 'NONE',  ( 33.58253175000000823, 6.275000002731184523, 10.91162601494192863 ) ) ;
#25417=CARTESIAN_POINT ( 'NONE',  ( 10.37757302488624767, 55.97500000273118559, 31.93888565452638417 ) ) ;
#25419=CARTESIAN_POINT ( 'NONE',  ( -1.137977401836464321E-14, 66.99999999999998579, 46.18802153517007270 ) ) ;
#25421=CARTESIAN_POINT ( 'NONE',  ( 26.29305231718578995, 61.70000000546237118, -19.10302069950538240 ) ) ;
#25428=CARTESIAN_POINT ( 'NONE',  ( -20.75514604977248823, 37.07500000273120122, -28.56700777964554305 ) ) ;
#25433=CARTESIAN_POINT ( 'NONE',  ( -26.29305231718578995, 26.70000000546236762, 19.10302069950538595 ) ) ;
#25452=CARTESIAN_POINT ( 'NONE',  ( 20.52662985655321393, 52.00000000000000000, 26.66963712870524716 ) ) ;
#25453=CARTESIAN_POINT ( 'NONE',  ( 20.08610463437157279, 5.300000000000006928, -27.64615127144129758 ) ) ;
#25459=CARTESIAN_POINT ( 'NONE',  ( -10.37757302488623701, 57.52500000273118275, 31.93888565452638417 ) ) ;
#25460=CARTESIAN_POINT ( 'NONE',  ( 20.75514604977249178, 24.07500000273120122, 28.56700777964553950 ) ) ;
#25461=CARTESIAN_POINT ( 'NONE',  ( -10.37757302488624411, 12.97500000273120513, -31.93888565452638417 ) ) ;
#25466=CARTESIAN_POINT ( 'NONE',  ( -33.58253175000000113, 1.225000002731198467, 10.91162601494193929 ) ) ;
#25468=CARTESIAN_POINT ( 'NONE',  ( 20.08610463437157279, 41.30000000000001137, -27.64615127144129758 ) ) ;
#25473=CARTESIAN_POINT ( 'NONE',  ( 10.37757302488624056, 58.77500000273121117, -31.93888565452638417 ) ) ;
#25479=CARTESIAN_POINT ( 'NONE',  ( 6.486482029760649416E-15, 29.62500000273120193, 35.31076352940723240 ) ) ;
#25498=CARTESIAN_POINT ( 'NONE',  ( -33.58253175000000113, 79.02500000273118985, -10.91162601494193218 ) ) ;
#25499=CARTESIAN_POINT ( 'NONE',  ( -10.37757302488624411, 42.97500000273117848, -31.93888565452638417 ) ) ;
#25505=CARTESIAN_POINT ( 'NONE',  ( -20.08610463437156923, 62.29999999999997584, 27.64615127144130113 ) ) ;
#25509=CARTESIAN_POINT ( 'NONE',  ( -33.58253175000000113, 79.37500000273119838, 0.000000000000000000 ) ) ;
#25515=CARTESIAN_POINT ( 'NONE',  ( 10.37757302488624767, 49.72500000273117848, 31.93888565452638417 ) ) ;
#25516=CARTESIAN_POINT ( 'NONE',  ( 20.75514604977248467, 24.67500000273118843, -28.56700777964554305 ) ) ;
#25517=VERTEX_POINT ( 'NONE', #29905 ) ;
#25530=CARTESIAN_POINT ( 'NONE',  ( -26.72982461517107566, 67.00000000000000000, -20.44820386143222635 ) ) ;
#25541=CARTESIAN_POINT ( 'NONE',  ( -27.16883889988624290, 65.17500000273116711, -19.73931689729374028 ) ) ;
#25547=CARTESIAN_POINT ( 'NONE',  ( 10.04305231718578817, 79.40000000000000568, -30.90933677959249337 ) ) ;
#25548=CARTESIAN_POINT ( 'NONE',  ( 33.58253175000000113, 22.22500000273117493, -10.91162601494193751 ) ) ;
#25550=CARTESIAN_POINT ( 'NONE',  ( 20.08610463437158344, 55.20000000546238539, 27.64615127144129403 ) ) ;
#25553=CARTESIAN_POINT ( 'NONE',  ( -20.08610463437156923, 38.80000000546237260, 27.64615127144130113 ) ) ;
#25559=CARTESIAN_POINT ( 'NONE',  ( -27.16883889988623935, 67.32500000273118701, 19.73931689729374739 ) ) ;
#25565=CARTESIAN_POINT ( 'NONE',  ( -10.37757302488623701, 11.52500000273119696, 31.93888565452638417 ) ) ;
#25574=CARTESIAN_POINT ( 'NONE',  ( -2.092463501923844636E-15, 29.49999999999999645, -34.17252228774368916 ) ) ;
#25587=CARTESIAN_POINT ( 'NONE',  ( 27.16883889988624290, 37.92500000273117422, 19.73931689729373673 ) ) ;
#25588=CARTESIAN_POINT ( 'NONE',  ( -20.75514604977248823, 3.075000002731183901, -28.56700777964554305 ) ) ;
#25589=CARTESIAN_POINT ( 'NONE',  ( 33.58253175000000113, 54.37500000273119838, -4.112674001490185761E-15 ) ) ;
#25594=CARTESIAN_POINT ( 'NONE',  ( -10.04305231718578462, 58.90000000546240244, 30.90933677959249337 ) ) ;
#25602=CARTESIAN_POINT ( 'NONE',  ( -33.58253175000000113, 33.47500000273119269, 10.91162601494193929 ) ) ;
#25606=CARTESIAN_POINT ( 'NONE',  ( 32.50000000000000000, 23.50000000546238610, -3.980102097228898626E-15 ) ) ;
#25625=ADVANCED_FACE ( 'NONE', ( #9830 ), #27680, .F. ) ;
#25626=CARTESIAN_POINT ( 'NONE',  ( -27.16883889988624290, 73.17500000273118133, -19.73931689729374028 ) ) ;
#25631=CARTESIAN_POINT ( 'NONE',  ( 10.37757302488624056, 58.52500000273118275, -31.93888565452638417 ) ) ;
#25632=CARTESIAN_POINT ( 'NONE',  ( 33.58253175000000113, 26.47500000273118559, -10.91162601494193751 ) ) ;
#25633=CARTESIAN_POINT ( 'NONE',  ( -20.75514604977248823, 13.07500000273118879, -28.56700777964554305 ) ) ;
#25637=CARTESIAN_POINT ( 'NONE',  ( -20.75514604977248112, 5.425000002731182214, 28.56700777964554661 ) ) ;
#25639=CARTESIAN_POINT ( 'NONE',  ( -20.08610463437157989, 41.69999999999999574, -27.64615127144129758 ) ) ;
#25644=CARTESIAN_POINT ( 'NONE',  ( 33.58253175000000113, 56.47500000273116427, -10.91162601494193751 ) ) ;
#25645=CARTESIAN_POINT ( 'NONE',  ( 5.779280353836490358E-15, 59.00000000546238255, 32.49999999999999289 ) ) ;
#25649=CARTESIAN_POINT ( 'NONE',  ( -27.16883889988623935, 21.32500000273117280, 19.73931689729374739 ) ) ;
#25651=VERTEX_POINT ( 'NONE', #7426 ) ;
#25663=CARTESIAN_POINT ( 'NONE',  ( -5.147494310547531704, 52.44874571845314648, 32.49999999999996447 ) ) ;
#25668=CARTESIAN_POINT ( 'NONE',  ( 33.58253175000000113, 78.12500000273118417, -4.112674001490185761E-15 ) ) ;
#25669=CARTESIAN_POINT ( 'NONE',  ( -10.37757302488623701, 41.77500000273119696, 31.93888565452638417 ) ) ;
#25673=CARTESIAN_POINT ( 'NONE',  ( 32.50000000000000711, 58.90000000000000568, 10.55989012756945122 ) ) ;
#25678=CARTESIAN_POINT ( 'NONE',  ( 20.75514604977249178, 74.07500000273120122, 28.56700777964553950 ) ) ;
#25683=CARTESIAN_POINT ( 'NONE',  ( -10.37757302488623701, 47.52500000273117564, 31.93888565452638417 ) ) ;
#25687=CARTESIAN_POINT ( 'NONE',  ( 10.04305231718578817, 13.90000000546236159, -30.90933677959249337 ) ) ;
#25706=CARTESIAN_POINT ( 'NONE',  ( -20.75514604977248112, 61.67500000273117422, 28.56700777964554661 ) ) ;
#25709=ADVANCED_FACE ( 'NONE', ( #19786 ), #17390, .T. ) ;
#25713=CARTESIAN_POINT ( 'NONE',  ( 20.75514604977249178, 15.82500000273117102, 28.56700777964553950 ) ) ;
#25716=EDGE_CURVE ( 'NONE', #30177, #2261, #64, .T. ) ;
#25719=CARTESIAN_POINT ( 'NONE',  ( -32.50000000000000000, 42.50000000546237544, 0.000000000000000000 ) ) ;
#25725=CARTESIAN_POINT ( 'NONE',  ( 27.16883889988623935, 70.32500000273118701, -19.73931689729374384 ) ) ;
#25731=CARTESIAN_POINT ( 'NONE',  ( -2.162160676586881955E-15, 10.62500000273119127, -35.31076352940723240 ) ) ;
#25740=CARTESIAN_POINT ( 'NONE',  ( 26.29305231718578995, 31.19999999999999218, -19.10302069950538240 ) ) ;
#25744=CARTESIAN_POINT ( 'NONE',  ( -9.358181289160242500, 66.99999999999998579, 31.32043657353317201 ) ) ;
#25753=CARTESIAN_POINT ( 'NONE',  ( 33.58253175000000823, 40.02500000273119696, 10.91162601494192863 ) ) ;
#25754=CARTESIAN_POINT ( 'NONE',  ( 5.779280353836490358E-15, 65.00000000546236834, 32.49999999999999289 ) ) ;
#25755=CARTESIAN_POINT ( 'NONE',  ( 20.75514604977248467, 52.67500000273116711, -28.56700777964554305 ) ) ;
#25757=CARTESIAN_POINT ( 'NONE',  ( -1.778240108872766143E-15, 65.50000000000000000, -32.49999999999999289 ) ) ;
#25759=CARTESIAN_POINT ( 'NONE',  ( 10.04305231718578817, 63.90000000546238113, -30.90933677959249337 ) ) ;
#25765=DIRECTION ( 'NONE',  ( 0.8660254037844387076, 0.000000000000000000, -0.4999999999999998890 ) ) ;
#25766=CARTESIAN_POINT ( 'NONE',  ( -10.37757302488624411, 32.97500000273119269, -31.93888565452638417 ) ) ;
#25770=CARTESIAN_POINT ( 'NONE',  ( 20.08610463437157279, 25.80000000546239036, -27.64615127144129758 ) ) ;
#25775=EDGE_LOOP ( 'NONE', ( #1222, #17753, #26742, #22507 ) ) ;
#25780=CARTESIAN_POINT ( 'NONE',  ( -2.162160676586882350E-15, 58.62500000273118417, -35.31076352940722529 ) ) ;
#25789=CARTESIAN_POINT ( 'NONE',  ( -10.37757302488624411, 74.97500000273120691, -31.93888565452638417 ) ) ;
#25794=CARTESIAN_POINT ( 'NONE',  ( -2.162160676586881955E-15, 62.62500000273116996, -35.31076352940723240 ) ) ;
#25795=CARTESIAN_POINT ( 'NONE',  ( 33.58253175000000823, 18.27500000273118275, 10.91162601494192863 ) ) ;
#25796=CARTESIAN_POINT ( 'NONE',  ( 27.16883889988623935, 8.575000002731188786, -19.73931689729374384 ) ) ;
#25800=CARTESIAN_POINT ( 'NONE',  ( 20.75514604977248467, 2.425000002731189763, -28.56700777964554305 ) ) ;
#25802=CARTESIAN_POINT ( 'NONE',  ( 32.50000000000000000, 41.10000000000001563, -10.55989012756945833 ) ) ;
#25808=CARTESIAN_POINT ( 'NONE',  ( 33.58253175000000113, 52.37500000273119838, -4.112674001490185761E-15 ) ) ;
#25814=CARTESIAN_POINT ( 'NONE',  ( -10.37757302488624411, 24.72500000273118559, -31.93888565452638417 ) ) ;
#25828=CARTESIAN_POINT ( 'NONE',  ( 32.50000000000000000, 19.10000000000000497, -10.55989012756945833 ) ) ;
#25833=CARTESIAN_POINT ( 'NONE',  ( -2.162160676586881955E-15, 76.62500000273118417, -35.31076352940723240 ) ) ;
#25836=CARTESIAN_POINT ( 'NONE',  ( -2.162160676586881955E-15, 44.87500000273119127, -35.31076352940723240 ) ) ;
#25841=CARTESIAN_POINT ( 'NONE',  ( 26.29305231718579350, 60.80000000000000426, 19.10302069950537529 ) ) ;
#25845=CARTESIAN_POINT ( 'NONE',  ( -20.75514604977248112, 71.67500000273116711, 28.56700777964554661 ) ) ;
#25850=CARTESIAN_POINT ( 'NONE',  ( 10.37757302488624767, 41.72500000273119980, 31.93888565452638417 ) ) ;
#25854=CARTESIAN_POINT ( 'NONE',  ( 32.50000000000000000, 5.600000005462370645, -10.55989012756945833 ) ) ;
#25873=CARTESIAN_POINT ( 'NONE',  ( 10.37757302488624767, 61.97500000273119269, 31.93888565452638417 ) ) ;
#25878=CARTESIAN_POINT ( 'NONE',  ( -40.00000000000000711, 66.99999999999998579, -23.09401076758504345 ) ) ;
#25879=CARTESIAN_POINT ( 'NONE',  ( 10.37757302488624056, 12.52500000273119873, -31.93888565452638417 ) ) ;
#25884=CARTESIAN_POINT ( 'NONE',  ( 26.29305231718578995, 37.70000000546237828, -19.10302069950538240 ) ) ;
#25889=CARTESIAN_POINT ( 'NONE',  ( -27.16883889988623935, 65.32500000273118701, 19.73931689729374739 ) ) ;
#25897=CARTESIAN_POINT ( 'NONE',  ( -33.58253175000000113, 9.025000002731184523, -10.91162601494193218 ) ) ;
#25909=CARTESIAN_POINT ( 'NONE',  ( 32.50000000000000000, 29.00000000000001066, -3.980102097228898626E-15 ) ) ;
#25912=( BOUNDED_CURVE ( )  B_SPLINE_CURVE ( 2, ( #5784, #19332, #620, #3874, #24476, #3217, #21748, #29776, #950, #21578, #789, #456, #14013 ),
 .UNSPECIFIED., .F., .F. ) 
 B_SPLINE_CURVE_WITH_KNOTS ( ( 3, 2, 2, 2, 2, 2, 3 ),
 ( 0.3012820512820512664, 0.3025641025641025439, 0.3051282051282051544, 0.3076923076923077094, 0.3102564102564102644, 0.3128205128205128194, 0.3141025641025640969 ),
 .UNSPECIFIED. ) 
 CURVE ( )  GEOMETRIC_REPRESENTATION_ITEM ( )  RATIONAL_B_SPLINE_CURVE ( ( 0.9755282581475768211, 0.9755282581475768211, 1.000000000000000000, 0.9510565162951535312, 1.000000000000000000, 0.9510565162951535312, 1.000000000000000000, 0.9510565162951535312, 1.000000000000000000, 0.9510565162951535312, 1.000000000000000000, 0.9755282581475768211, 0.9755282581475768211 ) ) 
 REPRESENTATION_ITEM ( '' )  );
#25920=CARTESIAN_POINT ( 'NONE',  ( 29.41736854754607222, 66.99999999999997158, -14.41477566699509083 ) ) ;
#25922=CARTESIAN_POINT ( 'NONE',  ( -33.58253175000000113, 35.02500000273118275, -10.91162601494193218 ) ) ;
#25924=AXIS2_PLACEMENT_3D ( 'NONE', #31429, #20814, #25944 ) ;
#25927=CARTESIAN_POINT ( 'NONE',  ( -26.29305231718578995, 52.70000000546236407, 19.10302069950538595 ) ) ;
#25935=CARTESIAN_POINT ( 'NONE',  ( -27.16883889988623935, 35.57500000273118701, 19.73931689729374739 ) ) ;
#25939=CARTESIAN_POINT ( 'NONE',  ( -2.092463501923844636E-15, 22.00000000546238965, -34.17252228774368916 ) ) ;
#25944=DIRECTION ( 'NONE',  ( 0.000000000000000000, 0.000000000000000000, 1.000000000000000000 ) ) ;
#25950=CARTESIAN_POINT ( 'NONE',  ( -20.75514604977248112, 59.42500000273118843, 28.56700777964554661 ) ) ;
#25960=CARTESIAN_POINT ( 'NONE',  ( 27.16883889988624290, 76.17500000273118133, 19.73931689729373673 ) ) ;
#25965=CARTESIAN_POINT ( 'NONE',  ( 33.58253175000000113, 54.22500000273117848, -10.91162601494193751 ) ) ;
#25966=CARTESIAN_POINT ( 'NONE',  ( -10.37757302488624411, 18.97500000273118204, -31.93888565452638417 ) ) ;
#25967=CARTESIAN_POINT ( 'NONE',  ( 10.37757302488624056, 6.775000002731193405, -31.93888565452638417 ) ) ;
#25972=CARTESIAN_POINT ( 'NONE',  ( -10.04305231718579172, 78.10000000546239107, -30.90933677959248982 ) ) ;
#25973=CARTESIAN_POINT ( 'NONE',  ( 29.99227890624914039, 52.00000000000002132, -14.07346378240328910 ) ) ;
#25980=CARTESIAN_POINT ( 'NONE',  ( 33.58253175000000823, 54.27500000273118275, 10.91162601494192863 ) ) ;
#25985=CARTESIAN_POINT ( 'NONE',  ( 27.16883889988623935, 24.32500000273117635, -19.73931689729374384 ) ) ;
#25999=CARTESIAN_POINT ( 'NONE',  ( -10.04305231718578462, 18.40000000000001279, 30.90933677959249337 ) ) ;
#26006=CARTESIAN_POINT ( 'NONE',  ( -20.75514604977248823, 76.82500000273120122, -28.56700777964554305 ) ) ;
#26007=CARTESIAN_POINT ( 'NONE',  ( -33.58253175000000113, 39.47500000273117848, 10.91162601494193929 ) ) ;
#26014=CARTESIAN_POINT ( 'NONE',  ( -32.50000000000000000, 60.09999999999999432, 10.55989012756946366 ) ) ;
#26020=CARTESIAN_POINT ( 'NONE',  ( -33.58253175000000113, 73.27500000273118985, -10.91162601494193218 ) ) ;
#26026=CARTESIAN_POINT ( 'NONE',  ( -33.58253175000000113, 45.22500000273117848, 10.91162601494193929 ) ) ;
#26029=CYLINDRICAL_SURFACE ( 'NONE', #24831, 32.50000000000000000 ) ;
#26030=CARTESIAN_POINT ( 'NONE',  ( -10.04305231718579172, 6.100000005462375086, -30.90933677959248982 ) ) ;
#26049=CARTESIAN_POINT ( 'NONE',  ( 27.16883889988623935, 58.57500000273117990, -19.73931689729374384 ) ) ;
#26057=CARTESIAN_POINT ( 'NONE',  ( 20.75514604977248467, 12.42500000273117777, -28.56700777964554305 ) ) ;
#26062=CARTESIAN_POINT ( 'NONE',  ( 26.29305231718578995, 35.70000000546237828, -19.10302069950538240 ) ) ;
#26066=ORIENTED_EDGE ( 'NONE', *, *, #3297, .T. ) ;
#26067=CARTESIAN_POINT ( 'NONE',  ( -27.16883889988624290, 62.92500000273119554, -19.73931689729374028 ) ) ;
#26069=ORIENTED_EDGE ( 'NONE', *, *, #32784, .F. ) ;
#26072=CARTESIAN_POINT ( 'NONE',  ( -33.58253175000000113, 5.025000002731194293, -10.91162601494193218 ) ) ;
#26083=CARTESIAN_POINT ( 'NONE',  ( -10.04305231718579172, 29.60000000000000142, -30.90933677959248982 ) ) ;
#26087=CARTESIAN_POINT ( 'NONE',  ( -30.82792611048012787, 66.99999999999995737, 12.22707559850328174 ) ) ;
#26092=CARTESIAN_POINT ( 'NONE',  ( 15.83883214465800826, 67.00000000000004263, -29.08710441171870542 ) ) ;
#26094=CARTESIAN_POINT ( 'NONE',  ( 33.58253175000000823, 36.02500000273117564, 10.91162601494192863 ) ) ;
#26095=DIRECTION ( 'NONE',  ( 0.8660254037844387076, 0.000000000000000000, -0.4999999999999998890 ) ) ;
#26099=CARTESIAN_POINT ( 'NONE',  ( 10.04305231718578817, 51.90000000546239534, -30.90933677959249337 ) ) ;
#26101=( NAMED_UNIT ( * ) PLANE_ANGLE_UNIT ( ) SI_UNIT ( $, .RADIAN. ) );
#26106=CARTESIAN_POINT ( 'NONE',  ( 33.58253175000000113, 32.37500000273117706, -4.112674001490185761E-15 ) ) ;
#26110=CARTESIAN_POINT ( 'NONE',  ( -20.08610463437157989, 24.20000000546238184, -27.64615127144129758 ) ) ;
#26121=CARTESIAN_POINT ( 'NONE',  ( -27.16883889988624290, 62.92500000273119554, -19.73931689729374028 ) ) ;
#26126=DIRECTION ( 'NONE',  ( 0.000000000000000000, 0.000000000000000000, 1.000000000000000000 ) ) ;
#26131=CARTESIAN_POINT ( 'NONE',  ( 27.16883889988623935, 74.57500000273118701, -19.73931689729374384 ) ) ;
#26136=CARTESIAN_POINT ( 'NONE',  ( 27.16883889988624290, 53.92500000273118843, 19.73931689729373673 ) ) ;
#26137=CARTESIAN_POINT ( 'NONE',  ( 20.75514604977248467, 14.67500000273117955, -28.56700777964554305 ) ) ;
#26138=CARTESIAN_POINT ( 'NONE',  ( -33.58253175000000113, 5.375000002731181503, 0.000000000000000000 ) ) ;
#26141=EDGE_CURVE ( 'NONE', #13792, #24744, #12919, .T. ) ;
#26143=CARTESIAN_POINT ( 'NONE',  ( 10.04305231718579705, 75.10000000546239107, 30.90933677959248982 ) ) ;
#26144=CARTESIAN_POINT ( 'NONE',  ( 19.64450058003839672, 52.00000000000002132, -26.34187928026370429 ) ) ;
#26152=CARTESIAN_POINT ( 'NONE',  ( 27.16883889988624290, 54.17500000273118843, 19.73931689729373673 ) ) ;
#26157=CARTESIAN_POINT ( 'NONE',  ( 27.16883889988624290, 21.92500000273119198, 19.73931689729373673 ) ) ;
#26162=DIRECTION ( 'NONE',  ( 0.000000000000000000, -0.000000000000000000, 1.000000000000000000 ) ) ;
#26174=CARTESIAN_POINT ( 'NONE',  ( -10.04305231718579172, 17.59999999999999076, -30.90933677959248982 ) ) ;
#26180=CARTESIAN_POINT ( 'NONE',  ( 6.486482029760649416E-15, 71.62500000273119838, 35.31076352940723240 ) ) ;
#26181=CARTESIAN_POINT ( 'NONE',  ( -33.58253175000000113, 35.27500000273120406, -10.91162601494193218 ) ) ;
#26186=CARTESIAN_POINT ( 'NONE',  ( 32.50000000000000711, 54.90000000000001279, 10.55989012756945122 ) ) ;
#26191=CARTESIAN_POINT ( 'NONE',  ( -33.58253175000000113, 73.37500000273118417, 0.000000000000000000 ) ) ;
#26196=CARTESIAN_POINT ( 'NONE',  ( -33.58253175000000113, 43.02500000273118275, -10.91162601494193218 ) ) ;
#26200=CARTESIAN_POINT ( 'NONE',  ( 20.75514604977249178, 66.07500000273118701, 28.56700777964553950 ) ) ;
#26201=CARTESIAN_POINT ( 'NONE',  ( 26.29305231718579350, 7.300000005462367270, 19.10302069950537529 ) ) ;
#26220=CARTESIAN_POINT ( 'NONE',  ( 10.37757302488624056, 52.77500000273120406, -31.93888565452638417 ) ) ;
#26223=CARTESIAN_POINT ( 'NONE',  ( 2.205017735002230837E-13, 57.49999999999998579, -32.50000000000000000 ) ) ;
#26228=CARTESIAN_POINT ( 'NONE',  ( 10.04305231718579705, 78.59999999999999432, 30.90933677959248982 ) ) ;
#26229=CARTESIAN_POINT ( 'NONE',  ( -10.37757302488624411, 16.72500000273117848, -31.93888565452638417 ) ) ;
#26234=CARTESIAN_POINT ( 'NONE',  ( -20.08610463437157989, 36.20000000546237828, -27.64615127144129758 ) ) ;
#26239=CARTESIAN_POINT ( 'NONE',  ( 10.37757302488624056, 64.52500000273118985, -31.93888565452638417 ) ) ;
#26241=ORIENTED_EDGE ( 'NONE', *, *, #949, .F. ) ;
#26244=CARTESIAN_POINT ( 'NONE',  ( -33.58253175000000113, 7.225000002731182924, 10.91162601494193929 ) ) ;
#26253=CARTESIAN_POINT ( 'NONE',  ( -2.092463501923844636E-15, 23.49999999999998934, -34.17252228774368916 ) ) ;
#26265=CARTESIAN_POINT ( 'NONE',  ( 27.16883889988624290, 33.92500000273117422, 19.73931689729373673 ) ) ;
#26270=CARTESIAN_POINT ( 'NONE',  ( -32.50000000000000000, 56.50000000546238965, 0.000000000000000000 ) ) ;
#26277=CARTESIAN_POINT ( 'NONE',  ( 27.16883889988624290, 30.17500000273119909, 19.73931689729373673 ) ) ;
#26281=CARTESIAN_POINT ( 'NONE',  ( 32.50000000000000000, 19.60000000546237686, -10.55989012756945833 ) ) ;
#26293=CARTESIAN_POINT ( 'NONE',  ( -33.58253175000000113, 61.12500000273117706, 0.000000000000000000 ) ) ;
#26303=CARTESIAN_POINT ( 'NONE',  ( -27.16883889988623935, 73.57500000273118701, 19.73931689729374739 ) ) ;
#26307=CARTESIAN_POINT ( 'NONE',  ( 20.75514604977248467, 52.42500000273118133, -28.56700777964554305 ) ) ;
#26308=CARTESIAN_POINT ( 'NONE',  ( 10.37757302488624056, 14.77500000273117209, -31.93888565452638417 ) ) ;
#26309=CARTESIAN_POINT ( 'NONE',  ( -20.75514604977248823, 5.075000002731193227, -28.56700777964554305 ) ) ;
#26313=CARTESIAN_POINT ( 'NONE',  ( -10.04305231718579172, 72.10000000546239107, -30.90933677959248982 ) ) ;
#26314=CARTESIAN_POINT ( 'NONE',  ( 15.01861347032150640, 52.00000000000000711, -29.12398716250640263 ) ) ;
#26320=CARTESIAN_POINT ( 'NONE',  ( -10.37757302488624411, 52.97500000273118559, -31.93888565452638417 ) ) ;
#26326=CARTESIAN_POINT ( 'NONE',  ( 27.16883889988624290, 23.92500000273119198, 19.73931689729373673 ) ) ;
#26341=CARTESIAN_POINT ( 'NONE',  ( 20.08610463437158344, 16.69999999999999574, 27.64615127144129403 ) ) ;
#26347=CARTESIAN_POINT ( 'NONE',  ( 27.16883889988624290, 69.92500000273120975, 19.73931689729373673 ) ) ;
#26348=CARTESIAN_POINT ( 'NONE',  ( -33.58253175000000113, 37.37500000273118417, 0.000000000000000000 ) ) ;
#26354=CARTESIAN_POINT ( 'NONE',  ( -26.29305231718579350, 51.79999999999999716, -19.10302069950537884 ) ) ;
#26360=CARTESIAN_POINT ( 'NONE',  ( -10.37757302488623701, 75.77500000273117564, 31.93888565452638417 ) ) ;
#26365=CARTESIAN_POINT ( 'NONE',  ( 33.58253175000000113, 42.22500000273118559, -10.91162601494193751 ) ) ;
#26367=ADVANCED_FACE ( 'NONE', ( #8602 ), #6028, .T. ) ;
#26368=VERTEX_POINT ( 'NONE', #19249 ) ;
#26370=CARTESIAN_POINT ( 'NONE',  ( -5.147494310547423346, 60.94874572391552903, 32.50000000000000000 ) ) ;
#26371=CARTESIAN_POINT ( 'NONE',  ( -32.50000000000000000, 4.500000005462371000, 0.000000000000000000 ) ) ;
#26390=CARTESIAN_POINT ( 'NONE',  ( 27.16883889988623935, 54.57500000273117280, -19.73931689729374384 ) ) ;
#26396=CARTESIAN_POINT ( 'NONE',  ( 32.50000000000000000, 75.00000000000000000, -3.980102097228898626E-15 ) ) ;
#26397=CARTESIAN_POINT ( 'NONE',  ( 20.75514604977248467, 16.42500000273118133, -28.56700777964554305 ) ) ;
#26401=CARTESIAN_POINT ( 'NONE',  ( 20.08610463437157279, 37.80000000546239391, -27.64615127144129758 ) ) ;
#26407=CARTESIAN_POINT ( 'NONE',  ( -20.75514604977248112, 65.42500000273118133, 28.56700777964554661 ) ) ;
#26411=CARTESIAN_POINT ( 'NONE',  ( 33.58253175000000823, 8.025000002731188076, 10.91162601494192863 ) ) ;
#26421=CARTESIAN_POINT ( 'NONE',  ( -26.29305231718578995, 20.19999999999998153, 19.10302069950538595 ) ) ;
#26433=CARTESIAN_POINT ( 'NONE',  ( -25.10896554811091974, 52.00000000000000000, 21.28139962774348604 ) ) ;
#26434=CARTESIAN_POINT ( 'NONE',  ( 33.58253175000000113, 34.22500000273117848, -10.91162601494193751 ) ) ;
#26435=CARTESIAN_POINT ( 'NONE',  ( -10.04305231718579172, 64.10000000546239107, -30.90933677959248982 ) ) ;
#26440=CARTESIAN_POINT ( 'NONE',  ( 6.277390505771533514E-15, 53.00000000546237544, 34.17252228774368916 ) ) ;
#26447=CARTESIAN_POINT ( 'NONE',  ( -10.37757302488624411, 26.97500000273118914, -31.93888565452638417 ) ) ;
#26451=CARTESIAN_POINT ( 'NONE',  ( -32.50000000000000000, 16.60000000546238752, 10.55989012756946366 ) ) ;
#26461=CARTESIAN_POINT ( 'NONE',  ( 27.16883889988623935, 64.32500000273121543, -19.73931689729374384 ) ) ;
#26471=CARTESIAN_POINT ( 'NONE',  ( 10.37757302488624056, 68.77500000273118985, -31.93888565452638417 ) ) ;
#26476=CARTESIAN_POINT ( 'NONE',  ( -33.58253175000000113, 53.12500000273119838, 0.000000000000000000 ) ) ;
#26477=CARTESIAN_POINT ( 'NONE',  ( -20.75514604977248112, 15.67500000273117600, 28.56700777964554661 ) ) ;
#26478=CARTESIAN_POINT ( 'NONE',  ( -27.16883889988623935, 3.575000002731185234, 19.73931689729374739 ) ) ;
#26482=CARTESIAN_POINT ( 'NONE',  ( -32.50000000000000000, 74.40000000546234560, -10.55989012756945478 ) ) ;
#26483=CARTESIAN_POINT ( 'NONE',  ( 26.85105675556561167, 51.99999999999999289, -19.27006841923020275 ) ) ;
#26489=CARTESIAN_POINT ( 'NONE',  ( 33.58253175000000113, 46.37500000273119127, -4.112674001490185761E-15 ) ) ;
#26494=CARTESIAN_POINT ( 'NONE',  ( -2.162160676586881955E-15, 18.62500000273117351, -35.31076352940723240 ) ) ;
#26506=CARTESIAN_POINT ( 'NONE',  ( -26.29305231718578995, 64.20000000000001705, 19.10302069950538595 ) ) ;
#26510=CARTESIAN_POINT ( 'NONE',  ( -32.50000000000000000, 59.89999999999999147, -10.55989012756945300 ) ) ;
#26511=CARTESIAN_POINT ( 'NONE',  ( -2.092463501923844636E-15, 17.50000000000000000, -34.17252228774368916 ) ) ;
#26517=CARTESIAN_POINT ( 'NONE',  ( 27.16883889988623935, 72.32500000273118701, -19.73931689729374384 ) ) ;
#26518=CARTESIAN_POINT ( 'NONE',  ( -27.16883889988624290, 37.17500000273120264, -19.73931689729374028 ) ) ;
#26525=CARTESIAN_POINT ( 'NONE',  ( 32.50000000000000000, 53.09999999999998721, -10.55989012756945833 ) ) ;
#26530=CARTESIAN_POINT ( 'NONE',  ( 27.16883889988624290, 66.17500000273116711, 19.73931689729373673 ) ) ;
#26535=CARTESIAN_POINT ( 'NONE',  ( 33.58253175000000113, 42.12500000273118417, -4.112674001490185761E-15 ) ) ;
#26558=CARTESIAN_POINT ( 'NONE',  ( -27.16883889988623935, 55.57500000273117280, 19.73931689729374739 ) ) ;
#26565=CARTESIAN_POINT ( 'NONE',  ( -26.29305231718578995, 74.20000000000000284, 19.10302069950538595 ) ) ;
#26566=CARTESIAN_POINT ( 'NONE',  ( -33.58253175000000113, 9.225000002731190918, 10.91162601494193929 ) ) ;
#26575=CARTESIAN_POINT ( 'NONE',  ( -33.58253175000000113, 63.12500000273117706, 0.000000000000000000 ) ) ;
#26577=ORIENTED_EDGE ( 'NONE', *, *, #25716, .F. ) ;
#26580=CARTESIAN_POINT ( 'NONE',  ( 10.37757302488624056, 2.525000002731189852, -31.93888565452638417 ) ) ;
#26588=CARTESIAN_POINT ( 'NONE',  ( -26.29305231718579350, 52.30000000546237970, -19.10302069950537884 ) ) ;
#26590=CARTESIAN_POINT ( 'NONE',  ( 20.08610463437157279, 25.29999999999998650, -27.64615127144129758 ) ) ;
#26602=CARTESIAN_POINT ( 'NONE',  ( -0.3323905815833131383, 52.00000000000001421, 33.36564663192542923 ) ) ;
#26603=CARTESIAN_POINT ( 'NONE',  ( -33.58253175000000113, 35.22500000273119980, 10.91162601494193929 ) ) ;
#26608=CARTESIAN_POINT ( 'NONE',  ( 20.08610463437157279, 53.80000000546237970, -27.64615127144129758 ) ) ;
#26614=CARTESIAN_POINT ( 'NONE',  ( 33.58253175000000113, 26.37500000273117351, -4.112674001490185761E-15 ) ) ;
#26619=CARTESIAN_POINT ( 'NONE',  ( -10.04305231718578462, 18.90000000546236691, 30.90933677959249337 ) ) ;
#26630=CARTESIAN_POINT ( 'NONE',  ( -20.75514604977248112, 55.42500000273120264, 28.56700777964554661 ) ) ;
#26639=CARTESIAN_POINT ( 'NONE',  ( -33.58253175000000113, 69.37500000273121259, 0.000000000000000000 ) ) ;
#26644=CARTESIAN_POINT ( 'NONE',  ( -33.58253175000000113, 51.12500000273119127, 0.000000000000000000 ) ) ;
#26645=CARTESIAN_POINT ( 'NONE',  ( -2.162160676586881955E-15, 12.87500000273117884, -35.31076352940723240 ) ) ;
#26646=CARTESIAN_POINT ( 'NONE',  ( -10.37757302488623701, 5.775000002731192517, 31.93888565452638417 ) ) ;
#26650=CARTESIAN_POINT ( 'NONE',  ( -32.50000000000000000, 76.50000000546238255, 0.000000000000000000 ) ) ;
#26657=CARTESIAN_POINT ( 'NONE',  ( -20.75514604977248823, 45.07500000273117990, -28.56700777964554305 ) ) ;
#26662=CARTESIAN_POINT ( 'NONE',  ( 20.75514604977248467, 16.42500000273118133, -28.56700777964554305 ) ) ;
#26664=ADVANCED_FACE ( 'NONE', ( #7478 ), #23829, .T. ) ;
#26679=CARTESIAN_POINT ( 'NONE',  ( 26.29305231718578995, 11.20000000000000107, -19.10302069950538240 ) ) ;
#26685=CARTESIAN_POINT ( 'NONE',  ( 10.37757302488624767, 75.72500000273117848, 31.93888565452638417 ) ) ;
#26686=CARTESIAN_POINT ( 'NONE',  ( -33.58253175000000113, 31.37500000273117706, 0.000000000000000000 ) ) ;
#26691=CARTESIAN_POINT ( 'NONE',  ( -10.04305231718579172, 51.60000000000002274, -30.90933677959248982 ) ) ;
#26697=CARTESIAN_POINT ( 'NONE',  ( 27.16883889988623935, 66.57500000273118701, -19.73931689729374384 ) ) ;
#26703=CARTESIAN_POINT ( 'NONE',  ( 27.16883889988623935, 38.32500000273118701, -19.73931689729374384 ) ) ;
#26712=EDGE_CURVE ( 'NONE', #26368, #23797, #551, .T. ) ;
#26726=CARTESIAN_POINT ( 'NONE',  ( -10.37757302488623701, 57.77500000273121117, 31.93888565452638417 ) ) ;
#26734=CARTESIAN_POINT ( 'NONE',  ( 26.29305231718579350, 72.80000000000001137, 19.10302069950537529 ) ) ;
#26735=CARTESIAN_POINT ( 'NONE',  ( 33.58253175000000823, 12.02500000273117742, 10.91162601494192863 ) ) ;
#26742=ORIENTED_EDGE ( 'NONE', *, *, #2025, .T. ) ;
#26743=CARTESIAN_POINT ( 'NONE',  ( 33.58253175000000113, 56.22500000273117138, -10.91162601494193751 ) ) ;
#26747=CARTESIAN_POINT ( 'NONE',  ( -27.16883889988624290, 2.925000002731187543, -19.73931689729374028 ) ) ;
#26750=AXIS2_PLACEMENT_3D ( 'NONE', #17652, #32895, #14903 ) ;
#26757=CARTESIAN_POINT ( 'NONE',  ( 6.277390505771533514E-15, 22.49999999999998934, 34.17252228774368916 ) ) ;
#26768=CARTESIAN_POINT ( 'NONE',  ( 32.24336671818456779, 66.99999999999997158, -4.711964452985279550 ) ) ;
#26769=CARTESIAN_POINT ( 'NONE',  ( -29.96643421716997224, 51.99999999999999289, 13.17858490638463387 ) ) ;
#26771=CARTESIAN_POINT ( 'NONE',  ( 10.37757302488624767, 27.72500000273118914, 31.93888565452638417 ) ) ;
#26777=CARTESIAN_POINT ( 'NONE',  ( 6.277390505771533514E-15, 45.00000000546235412, 34.17252228774368916 ) ) ;
#26785=CARTESIAN_POINT ( 'NONE',  ( -26.29305231718578995, 16.70000000546238539, 19.10302069950538595 ) ) ;
#26795=CARTESIAN_POINT ( 'NONE',  ( -33.58253175000000113, 55.02500000273118985, -10.91162601494193041 ) ) ;
#26799=CARTESIAN_POINT ( 'NONE',  ( -26.29305231718579350, 66.30000000546236549, -19.10302069950537884 ) ) ;
#26803=CARTESIAN_POINT ( 'NONE',  ( -10.37757302488624411, 70.97500000273120691, -31.93888565452638417 ) ) ;
#26808=CARTESIAN_POINT ( 'NONE',  ( -33.58253175000000113, 47.12500000273119127, 0.000000000000000000 ) ) ;
#26809=CARTESIAN_POINT ( 'NONE',  ( -33.58253175000000113, 11.47500000273119625, 10.91162601494193929 ) ) ;
#26810=CARTESIAN_POINT ( 'NONE',  ( -20.75514604977248112, 61.67500000273117422, 28.56700777964554661 ) ) ;
#26814=CARTESIAN_POINT ( 'NONE',  ( 20.08610463437157279, 71.80000000546236549, -27.64615127144129758 ) ) ;
#26821=CARTESIAN_POINT ( 'NONE',  ( 20.75514604977249178, 48.07500000273120122, 28.56700777964553950 ) ) ;
#26826=CARTESIAN_POINT ( 'NONE',  ( 20.75514604977249178, 15.82500000273117102, 28.56700777964553950 ) ) ;
#26838=CARTESIAN_POINT ( 'NONE',  ( 5.147494310547434893, 65.05125428700921475, 32.49999999999999289 ) ) ;
#26840=CARTESIAN_POINT ( 'NONE',  ( 10.04305231718578817, 9.400000000000005684, -30.90933677959249337 ) ) ;
#26846=CARTESIAN_POINT ( 'NONE',  ( 10.37757302488624056, 70.52500000273118985, -31.93888565452638417 ) ) ;
#26847=CARTESIAN_POINT ( 'NONE',  ( -27.16883889988623935, 29.57500000273117990, 19.73931689729374739 ) ) ;
#26848=CARTESIAN_POINT ( 'NONE',  ( -27.16883889988623935, 13.57500000273119412, 19.73931689729374739 ) ) ;
#26855=CARTESIAN_POINT ( 'NONE',  ( -20.08610463437157989, 53.69999999999999574, -27.64615127144129758 ) ) ;
#26861=CARTESIAN_POINT ( 'NONE',  ( 20.75514604977249178, 66.07500000273118701, 28.56700777964553950 ) ) ;
#26865=ORIENTED_EDGE ( 'NONE', *, *, #11313, .F. ) ;
#26866=CARTESIAN_POINT ( 'NONE',  ( 6.486482029760649416E-15, 37.62500000273118417, 35.31076352940723240 ) ) ;
#26870=CARTESIAN_POINT ( 'NONE',  ( 5.779280353836490358E-15, 61.00000000546238255, 32.49999999999999289 ) ) ;
#26887=CARTESIAN_POINT ( 'NONE',  ( 27.16883889988624290, 48.17500000273118843, 19.73931689729373673 ) ) ;
#26892=CARTESIAN_POINT ( 'NONE',  ( -26.29305231718578995, 70.20000000000000284, 19.10302069950538595 ) ) ;
#26893=CARTESIAN_POINT ( 'NONE',  ( -10.37757302488624411, 8.725000002731173154, -31.93888565452638417 ) ) ;
#26902=CARTESIAN_POINT ( 'NONE',  ( 20.75514604977249178, 57.82500000273118701, 28.56700777964553950 ) ) ;
#26916=CARTESIAN_POINT ( 'NONE',  ( -32.50000000000000000, 22.09999999999999787, 10.55989012756946366 ) ) ;
#26926=CARTESIAN_POINT ( 'NONE',  ( -20.30017892146885217, 52.00000000000002132, 26.02681000244164267 ) ) ;
#26927=CARTESIAN_POINT ( 'NONE',  ( 33.58253175000000823, 28.02500000273119340, 10.91162601494192863 ) ) ;
#26929=CARTESIAN_POINT ( 'NONE',  ( 32.50000000000000000, 65.10000000000000853, -10.55989012756945833 ) ) ;
#26933=CARTESIAN_POINT ( 'NONE',  ( 20.08610463437158344, 51.20000000546237828, 27.64615127144129403 ) ) ;
#26938=CARTESIAN_POINT ( 'NONE',  ( 27.16883889988624290, 75.92500000273120975, 19.73931689729373673 ) ) ;
#26943=CARTESIAN_POINT ( 'NONE',  ( 10.04305231718579705, 15.10000000546239640, 30.90933677959248982 ) ) ;
#26960=CARTESIAN_POINT ( 'NONE',  ( 27.16883889988623935, 70.57500000273118701, -19.73931689729374384 ) ) ;
#26965=CARTESIAN_POINT ( 'NONE',  ( -10.37757302488624411, 46.72500000273120691, -31.93888565452638417 ) ) ;
#26966=CARTESIAN_POINT ( 'NONE',  ( 27.16883889988623935, 8.575000002731188786, -19.73931689729374384 ) ) ;
#26967=CARTESIAN_POINT ( 'NONE',  ( 10.37757302488624056, 62.77500000273118985, -31.93888565452638417 ) ) ;
#26971=CARTESIAN_POINT ( 'NONE',  ( 26.29305231718578995, 69.70000000546238539, -19.10302069950538240 ) ) ;
#26979=CARTESIAN_POINT ( 'NONE',  ( -20.75514604977248112, 47.67500000273118843, 28.56700777964554661 ) ) ;
#26984=CARTESIAN_POINT ( 'NONE',  ( -10.37757302488624411, 14.72500000273117848, -31.93888565452638417 ) ) ;
#26993=VECTOR ( 'NONE', #23395, 999.9999999999998863 ) ;
#27001=CARTESIAN_POINT ( 'NONE',  ( -32.50000000000000000, 7.900000000000012790, -10.55989012756945478 ) ) ;
#27008=CARTESIAN_POINT ( 'NONE',  ( 33.58253175000000113, 68.12500000273118417, -4.112674001490185761E-15 ) ) ;
#27009=CARTESIAN_POINT ( 'NONE',  ( -33.58253175000000113, 33.27500000273120406, -10.91162601494193218 ) ) ;
#27010=CARTESIAN_POINT ( 'NONE',  ( 20.75514604977249178, 18.07500000273119056, 28.56700777964553950 ) ) ;
#27018=CARTESIAN_POINT ( 'NONE',  ( -10.04305231718578462, 50.39999999999998437, 30.90933677959249337 ) ) ;
#27024=CARTESIAN_POINT ( 'NONE',  ( 10.37757302488624056, 68.77500000273118985, -31.93888565452638417 ) ) ;
#27029=CARTESIAN_POINT ( 'NONE',  ( 10.37757302488624056, 34.52500000273118985, -31.93888565452638417 ) ) ;
#27047=CARTESIAN_POINT ( 'NONE',  ( 32.50000000000000711, 53.40000000546238113, 10.55989012756945122 ) ) ;
#27052=CARTESIAN_POINT ( 'NONE',  ( 33.58253175000000113, 46.37500000273119127, -4.112674001490185761E-15 ) ) ;
#27058=CARTESIAN_POINT ( 'NONE',  ( 10.04305231718579705, 70.59999999999998010, 30.90933677959248982 ) ) ;
#27059=CARTESIAN_POINT ( 'NONE',  ( -20.75514604977248112, 7.425000002731191984, 28.56700777964554661 ) ) ;
#27070=CARTESIAN_POINT ( 'NONE',  ( 27.16883889988623935, 58.32500000273120833, -19.73931689729374384 ) ) ;
#27096=FACE_OUTER_BOUND ( 'NONE', #13193, .T. ) ;
#27099=CARTESIAN_POINT ( 'NONE',  ( -33.58253175000000113, 31.02500000273118630, -10.91162601494193218 ) ) ;
#27100=CARTESIAN_POINT ( 'NONE',  ( 20.08610463437158344, 56.69999999999998153, 27.64615127144129403 ) ) ;
#27104=CARTESIAN_POINT ( 'NONE',  ( 10.04305231718579705, 47.10000000546236976, 30.90933677959248982 ) ) ;
#27106=DIRECTION ( 'NONE',  ( 0.000000000000000000, 0.000000000000000000, -1.000000000000000000 ) ) ;
#27109=CARTESIAN_POINT ( 'NONE',  ( -33.58253175000000113, 77.02500000273118985, -10.91162601494193218 ) ) ;
#27113=DIRECTION ( 'NONE',  ( 0.000000000000000000, 1.000000000000000000, 0.000000000000000000 ) ) ;
#27116=CARTESIAN_POINT ( 'NONE',  ( 26.29305231718579350, 11.30000000546237082, 19.10302069950537529 ) ) ;
#27123=CARTESIAN_POINT ( 'NONE',  ( -5.147494310547478413, 62.94874572391552192, 32.49999999999998579 ) ) ;
#27125=CARTESIAN_POINT ( 'NONE',  ( 20.08610463437158344, 32.69999999999998863, 27.64615127144129403 ) ) ;
#27132=CARTESIAN_POINT ( 'NONE',  ( 33.58253175000000823, 70.27500000273118985, 10.91162601494192863 ) ) ;
#27138=CARTESIAN_POINT ( 'NONE',  ( 33.58253175000000823, 48.02500000273119696, 10.91162601494192863 ) ) ;
#27139=CARTESIAN_POINT ( 'NONE',  ( 27.16883889988624290, 8.175000002731177773, 19.73931689729373673 ) ) ;
#27140=CARTESIAN_POINT ( 'NONE',  ( 10.37757302488624767, 61.97500000273119269, 31.93888565452638417 ) ) ;
#27144=CARTESIAN_POINT ( 'NONE',  ( -32.50000000000000000, 68.40000000546237402, -10.55989012756945478 ) ) ;
#27151=CARTESIAN_POINT ( 'NONE',  ( -33.58253175000000113, 45.27500000273116854, -10.91162601494193218 ) ) ;
#27154=CARTESIAN_POINT ( 'NONE',  ( -10.04305231718579172, 28.10000000546238041, -30.90933677959248982 ) ) ;
#27155=ORIENTED_EDGE ( 'NONE', *, *, #2025, .F. ) ;
#27156=CARTESIAN_POINT ( 'NONE',  ( 33.58253175000000113, 18.22500000273118559, -10.91162601494193751 ) ) ;
#27172=EDGE_CURVE ( 'NONE', #23797, #24301, #4056, .T. ) ;
#27173=CARTESIAN_POINT ( 'NONE',  ( 26.29305231718579350, 10.80000000000001847, 19.10302069950537529 ) ) ;
#27179=CARTESIAN_POINT ( 'NONE',  ( -27.16883889988623935, 67.32500000273118701, 19.73931689729374739 ) ) ;
#27180=CARTESIAN_POINT ( 'NONE',  ( -33.58253175000000113, 29.47500000273117848, 10.91162601494193929 ) ) ;
#27181=CARTESIAN_POINT ( 'NONE',  ( -20.75514604977248112, 17.67500000273117422, 28.56700777964554661 ) ) ;
#27188=CARTESIAN_POINT ( 'NONE',  ( 26.29305231718579350, 48.79999999999999716, 19.10302069950537529 ) ) ;
#27189=CARTESIAN_POINT ( 'NONE',  ( 10.04305231718578817, 57.90000000546240244, -30.90933677959249337 ) ) ;
#27191=APPLICATION_CONTEXT ( 'automotive_design' ) ;
#27193=ADVANCED_FACE ( 'NONE', ( #225, #7793 ), #23591, .T. ) ;
#27195=CARTESIAN_POINT ( 'NONE',  ( -33.58253175000000113, 65.37500000273121259, 0.000000000000000000 ) ) ;
#27199=ORIENTED_EDGE ( 'NONE', *, *, #33754, .F. ) ;
#27200=CARTESIAN_POINT ( 'NONE',  ( 10.37757302488624056, 36.52500000273118985, -31.93888565452638417 ) ) ;
#27205=CARTESIAN_POINT ( 'NONE',  ( 26.29305231718579350, 58.80000000000000426, 19.10302069950537529 ) ) ;
#27221=CARTESIAN_POINT ( 'NONE',  ( 6.486482029760649416E-15, 51.87500000273119127, 35.31076352940723240 ) ) ;
#27227=CARTESIAN_POINT ( 'NONE',  ( 20.08610463437158344, 64.70000000000001705, 27.64615127144129403 ) ) ;
#27228=CARTESIAN_POINT ( 'NONE',  ( -10.37757302488624411, 6.725000002731185589, -31.93888565452638417 ) ) ;
#27239=CARTESIAN_POINT ( 'NONE',  ( -10.37757302488624411, 54.72500000273118559, -31.93888565452638417 ) ) ;
#27240=CARTESIAN_POINT ( 'NONE',  ( -33.58253175000000113, 29.47500000273117848, 10.91162601494193929 ) ) ;
#27266=DIRECTION ( 'NONE',  ( -0.5000000000000001110, 0.000000000000000000, -0.8660254037844387076 ) ) ;
#27267=CARTESIAN_POINT ( 'NONE',  ( -32.24336671818454647, 52.00000000000002132, 4.711964452985278662 ) ) ;
#27268=CARTESIAN_POINT ( 'NONE',  ( -33.58253175000000113, 31.22500000273118559, 10.91162601494193929 ) ) ;
#27273=CARTESIAN_POINT ( 'NONE',  ( 20.08610463437158344, 45.20000000546239249, 27.64615127144129403 ) ) ;
#27278=CARTESIAN_POINT ( 'NONE',  ( 27.16883889988624290, 73.92500000273120975, 19.73931689729373673 ) ) ;
#27284=CARTESIAN_POINT ( 'NONE',  ( -10.04305231718578462, 12.90000000546236159, 30.90933677959249337 ) ) ;
#27291=CARTESIAN_POINT ( 'NONE',  ( 5.779280353836490358E-15, 57.00000000546238965, 32.49999999999999289 ) ) ;
#27293=FILL_AREA_STYLE ('',( #29518 ) ) ;
#27294=CARTESIAN_POINT ( 'NONE',  ( 26.29305231718579350, 38.79999999999999005, 19.10302069950537529 ) ) ;
#27302=CARTESIAN_POINT ( 'NONE',  ( -33.58253175000000113, 61.47500000273117848, 10.91162601494193929 ) ) ;
#27308=CARTESIAN_POINT ( 'NONE',  ( 10.37757302488624056, 50.52500000273117564, -31.93888565452638417 ) ) ;
#27309=CARTESIAN_POINT ( 'NONE',  ( -10.37757302488624411, 8.975000002731201576, -31.93888565452638417 ) ) ;
#27310=CARTESIAN_POINT ( 'NONE',  ( -33.58253175000000113, 61.27500000273118985, -10.91162601494193041 ) ) ;
#27315=CARTESIAN_POINT ( 'NONE',  ( 10.04305231718578817, 69.90000000546238823, -30.90933677959249337 ) ) ;
#27324=CARTESIAN_POINT ( 'NONE',  ( -10.37757302488623701, 39.77500000273119696, 31.93888565452638417 ) ) ;
#27326=CARTESIAN_POINT ( 'NONE',  ( -32.50000000000000000, 30.40000000546238823, -10.55989012756945478 ) ) ;
#27345=CARTESIAN_POINT ( 'NONE',  ( -10.04305231718578462, 8.400000000000003908, 30.90933677959249337 ) ) ;
#27346=ORIENTED_EDGE ( 'NONE', *, *, #9844, .F. ) ;
#27351=CARTESIAN_POINT ( 'NONE',  ( 33.58253175000000823, 68.02500000273117564, 10.91162601494192863 ) ) ;
#27352=CARTESIAN_POINT ( 'NONE',  ( 27.16883889988623935, 28.57500000273117990, -19.73931689729374384 ) ) ;
#27353=CARTESIAN_POINT ( 'NONE',  ( -33.58253175000000113, 17.37500000273119127, 0.000000000000000000 ) ) ;
#27359=CARTESIAN_POINT ( 'NONE',  ( 10.04305231718579705, 48.59999999999998721, 30.90933677959248982 ) ) ;
#27364=CARTESIAN_POINT ( 'NONE',  ( 27.16883889988623935, 62.57500000273117990, -19.73931689729374384 ) ) ;
#27369=CARTESIAN_POINT ( 'NONE',  ( -27.16883889988624290, 34.92500000273117422, -19.73931689729374028 ) ) ;
#27389=CARTESIAN_POINT ( 'NONE',  ( 20.75514604977249178, 50.07500000273120122, 28.56700777964553950 ) ) ;
#27395=CARTESIAN_POINT ( 'NONE',  ( 32.50000000000000711, 66.90000000000001990, 10.55989012756945122 ) ) ;
#27401=CARTESIAN_POINT ( 'NONE',  ( -20.75514604977248823, 77.07500000273117280, -28.56700777964554305 ) ) ;
#27406=CARTESIAN_POINT ( 'NONE',  ( -33.58253175000000113, 53.12500000273119838, 0.000000000000000000 ) ) ;
#27407=CARTESIAN_POINT ( 'NONE',  ( -2.162160676586881955E-15, 30.87500000273119483, -35.31076352940723240 ) ) ;
#27421=CARTESIAN_POINT ( 'NONE',  ( 10.37757302488624056, 54.52500000273118275, -31.93888565452638417 ) ) ;
#27435=CARTESIAN_POINT ( 'NONE',  ( -2.162160676586881955E-15, 30.62500000273119838, -35.31076352940723240 ) ) ;
#27440=CARTESIAN_POINT ( 'NONE',  ( -2.092463501923844636E-15, 50.00000000546237544, -34.17252228774368916 ) ) ;
#27445=CARTESIAN_POINT ( 'NONE',  ( -10.37757302488624411, 76.72500000273117848, -31.93888565452638417 ) ) ;
#27451=CARTESIAN_POINT ( 'NONE',  ( -20.08610463437157989, 12.20000000546237828, -27.64615127144129758 ) ) ;
#27460=DIRECTION ( 'NONE',  ( 0.000000000000000000, 0.000000000000000000, 1.000000000000000000 ) ) ;
#27461=CARTESIAN_POINT ( 'NONE',  ( -20.08610463437157989, 35.70000000000000995, -27.64615127144129758 ) ) ;
#27476=CARTESIAN_POINT ( 'NONE',  ( -27.16883889988624290, 48.92500000273118843, -19.73931689729374028 ) ) ;
#27477=CARTESIAN_POINT ( 'NONE',  ( 10.37757302488624767, 5.975000002731184701, 31.93888565452638417 ) ) ;
#27478=CARTESIAN_POINT ( 'NONE',  ( -33.58253175000000113, 59.37500000273119838, 0.000000000000000000 ) ) ;
#27482=CARTESIAN_POINT ( 'NONE',  ( -20.08610463437157989, 68.20000000546239960, -27.64615127144129758 ) ) ;
#27485=CARTESIAN_POINT ( 'NONE',  ( -20.08610463437156923, 54.30000000000000426, 27.64615127144130113 ) ) ;
#27488=CARTESIAN_POINT ( 'NONE',  ( 33.58253175000000113, 42.37500000273118417, -4.112674001490185761E-15 ) ) ;
#27491=CARTESIAN_POINT ( 'NONE',  ( -20.08610463437156923, 26.80000000546238681, 27.64615127144130113 ) ) ;
#27511=CARTESIAN_POINT ( 'NONE',  ( 10.04305231718579705, 2.599999999999991207, 30.90933677959248982 ) ) ;
#27517=CARTESIAN_POINT ( 'NONE',  ( 33.58253175000000823, 64.02500000273118985, 10.91162601494192863 ) ) ;
#27518=CARTESIAN_POINT ( 'NONE',  ( -10.37757302488624411, 22.97500000273118559, -31.93888565452638417 ) ) ;
#27519=CARTESIAN_POINT ( 'NONE',  ( -33.58253175000000113, 17.27500000273118630, -10.91162601494193218 ) ) ;
#27524=CARTESIAN_POINT ( 'NONE',  ( -20.08610463437156923, 46.29999999999999716, 27.64615127144130113 ) ) ;
#27528=CARTESIAN_POINT ( 'NONE',  ( -20.75514604977248112, 63.67500000273116711, 28.56700777964554661 ) ) ;
#27534=CARTESIAN_POINT ( 'NONE',  ( 33.58253175000000823, 28.02500000273119340, 10.91162601494192863 ) ) ;
#27556=CARTESIAN_POINT ( 'NONE',  ( 10.37757302488624767, 51.97500000273118559, 31.93888565452638417 ) ) ;
#27563=CARTESIAN_POINT ( 'NONE',  ( -32.50000000000000000, 68.09999999999995168, 10.55989012756946366 ) ) ;
#27568=CARTESIAN_POINT ( 'NONE',  ( -33.58253175000000113, 77.47500000273120691, 10.91162601494193929 ) ) ;
#27573=CARTESIAN_POINT ( 'NONE',  ( -33.58253175000000113, 47.02500000273116854, -10.91162601494193218 ) ) ;
#27574=CARTESIAN_POINT ( 'NONE',  ( -10.37757302488624411, 24.97500000273118914, -31.93888565452638417 ) ) ;
#27585=CARTESIAN_POINT ( 'NONE',  ( 32.49999999999965183, 66.90000000000001990, 10.55989012756993795 ) ) ;
#27588=CARTESIAN_POINT ( 'NONE',  ( -33.58253175000000113, 57.22500000273117848, 10.91162601494193929 ) ) ;
#27598=LINE ( 'NONE', #14563, #14479 ) ;
#27601=CARTESIAN_POINT ( 'NONE',  ( -31.92269207768538308, 51.99999999999999289, 6.710300343870669870 ) ) ;
#27602=CARTESIAN_POINT ( 'NONE',  ( 20.75514604977249178, 19.82500000273119412, 28.56700777964553950 ) ) ;
#27604=CARTESIAN_POINT ( 'NONE',  ( 10.04305231718579705, 52.60000000000002274, 30.90933677959248982 ) ) ;
#27611=CARTESIAN_POINT ( 'NONE',  ( -20.08610463437157989, 44.20000000546238539, -27.64615127144129758 ) ) ;
#27618=CARTESIAN_POINT ( 'NONE',  ( 33.58253175000000113, 78.12500000273118417, -4.112674001490185761E-15 ) ) ;
#27623=CARTESIAN_POINT ( 'NONE',  ( -26.29305231718579350, 10.30000000546237082, -19.10302069950537884 ) ) ;
#27633=CARTESIAN_POINT ( 'NONE',  ( -26.29305231718578995, 34.19999999999999574, 19.10302069950538595 ) ) ;
#27646=CARTESIAN_POINT ( 'NONE',  ( 20.75514604977248467, 40.42500000273117422, -28.56700777964554305 ) ) ;
#27647=CARTESIAN_POINT ( 'NONE',  ( -33.58253175000000113, 5.375000002731181503, 0.000000000000000000 ) ) ;
#27648=CARTESIAN_POINT ( 'NONE',  ( 10.37757302488624056, 58.77500000273121117, -31.93888565452638417 ) ) ;
#27652=CARTESIAN_POINT ( 'NONE',  ( -26.29305231718579350, 64.30000000546236549, -19.10302069950537884 ) ) ;
#27658=CARTESIAN_POINT ( 'NONE',  ( -33.58253175000000113, 43.37500000273118417, 0.000000000000000000 ) ) ;
#27661=CARTESIAN_POINT ( 'NONE',  ( -20.08610463437157989, 30.20000000546236407, -27.64615127144129758 ) ) ;
#27664=ORIENTED_EDGE ( 'NONE', *, *, #33257, .F. ) ;
#27670=CARTESIAN_POINT ( 'NONE',  ( -20.75514604977248112, 65.42500000273116711, 28.56700777964554661 ) ) ;
#27680=CYLINDRICAL_SURFACE ( 'NONE', #5152, 32.50000000000000000 ) ;
#27681=CARTESIAN_POINT ( 'NONE',  ( 26.29305231718579350, 6.800000000000000711, 19.10302069950537529 ) ) ;
#27686=CARTESIAN_POINT ( 'NONE',  ( -33.58253175000000113, 65.22500000273117848, 10.91162601494193929 ) ) ;
#27687=CARTESIAN_POINT ( 'NONE',  ( -2.162160676586881955E-15, 24.87500000273117351, -35.31076352940723240 ) ) ;
#27688=CARTESIAN_POINT ( 'NONE',  ( -33.58253175000000113, 7.275000002731196957, -10.91162601494193218 ) ) ;
#27693=CARTESIAN_POINT ( 'NONE',  ( -10.04305231718579172, 45.60000000000001563, -30.90933677959248982 ) ) ;
#27699=CARTESIAN_POINT ( 'NONE',  ( 33.58253175000000113, 58.37500000273119838, -4.112674001490185761E-15 ) ) ;
#27705=CARTESIAN_POINT ( 'NONE',  ( -33.58253175000000113, 33.12500000273120548, 0.000000000000000000 ) ) ;
#27721=CARTESIAN_POINT ( 'NONE',  ( 5.147494310547426899, 55.44874571845314648, -32.50000000000000000 ) ) ;
#27728=CARTESIAN_POINT ( 'NONE',  ( -2.162160676586881955E-15, 40.87500000273119838, -35.31076352940723240 ) ) ;
#27733=CARTESIAN_POINT ( 'NONE',  ( 10.04305231718579705, 66.60000000000000853, 30.90933677959248982 ) ) ;
#27742=CARTESIAN_POINT ( 'NONE',  ( -33.58253175000000113, 49.12500000273119127, 0.000000000000000000 ) ) ;
#27743=CARTESIAN_POINT ( 'NONE',  ( 27.16883889988624290, 22.17500000273119198, 19.73931689729373673 ) ) ;
#27756=CARTESIAN_POINT ( 'NONE',  ( 10.04305231718579705, 66.60000000000000853, 30.90933677959248982 ) ) ;
#27759=CARTESIAN_POINT ( 'NONE',  ( -10.37757302488624411, 56.72500000273118559, -31.93888565452638417 ) ) ;
#27771=CARTESIAN_POINT ( 'NONE',  ( 5.779280353836490358E-15, 56.49999999999998579, 32.49999999999999289 ) ) ;
#27774=CARTESIAN_POINT ( 'NONE',  ( 26.29305231718579350, 63.30000000546235839, 19.10302069950537529 ) ) ;
#27776=CARTESIAN_POINT ( 'NONE',  ( -33.58253175000000113, 23.02500000273117919, -10.91162601494193218 ) ) ;
#27778=CARTESIAN_POINT ( 'NONE',  ( 32.50000000000000711, 52.89999999999999147, 10.55989012756945122 ) ) ;
#27781=CARTESIAN_POINT ( 'NONE',  ( -20.08610463437156923, 42.80000000546236549, 27.64615127144130113 ) ) ;
#27787=CARTESIAN_POINT ( 'NONE',  ( 20.75514604977249178, 67.82500000273120122, 28.56700777964553950 ) ) ;
#27794=CARTESIAN_POINT ( 'NONE',  ( 33.58253175000000113, 8.225000002731182036, -10.91162601494193751 ) ) ;
#27804=CARTESIAN_POINT ( 'NONE',  ( 6.277390505771533514E-15, 38.50000000000000711, 34.17252228774368916 ) ) ;
#27818=CARTESIAN_POINT ( 'NONE',  ( 20.75514604977249178, 43.82500000273119412, 28.56700777964553950 ) ) ;
#27819=CARTESIAN_POINT ( 'NONE',  ( 33.58253175000000113, 4.475000002731183812, -10.91162601494193751 ) ) ;
#27820=CARTESIAN_POINT ( 'NONE',  ( -27.16883889988623935, 57.57500000273117990, 19.73931689729374739 ) ) ;
#27824=CARTESIAN_POINT ( 'NONE',  ( 6.277390505771533514E-15, 61.00000000546237544, 34.17252228774368916 ) ) ;
#27827=CARTESIAN_POINT ( 'NONE',  ( -1.778240108872766143E-15, 53.50000000000000000, -32.49999999999999289 ) ) ;
#27830=CARTESIAN_POINT ( 'NONE',  ( -27.16883889988623935, 43.57500000273119412, 19.73931689729374739 ) ) ;
#27834=CARTESIAN_POINT ( 'NONE',  ( -10.04305231718578462, 28.90000000546237402, 30.90933677959249337 ) ) ;
#27843=APPLICATION_CONTEXT ( 'automotive_design' ) ;
#27845=CARTESIAN_POINT ( 'NONE',  ( -33.58253175000000113, 65.02500000273118985, -10.91162601494193041 ) ) ;
#27854=CARTESIAN_POINT ( 'NONE',  ( -1.778240108872766143E-15, 55.49999999999999289, -32.49999999999999289 ) ) ;
#27855=CARTESIAN_POINT ( 'NONE',  ( -40.00000000000000711, 52.00000000000000711, 23.09401076758504345 ) ) ;
#27856=CARTESIAN_POINT ( 'NONE',  ( 33.58253175000000823, 78.27500000273116143, 10.91162601494192863 ) ) ;
#27861=CARTESIAN_POINT ( 'NONE',  ( -20.75514604977248112, 59.42500000273118843, 28.56700777964554661 ) ) ;
#27862=CARTESIAN_POINT ( 'NONE',  ( -33.58253175000000113, 21.47500000273119980, 10.91162601494193929 ) ) ;
#27863=CARTESIAN_POINT ( 'NONE',  ( -33.58253175000000113, 13.37500000273118772, 0.000000000000000000 ) ) ;
#27867=CARTESIAN_POINT ( 'NONE',  ( -33.58253175000000113, 1.125000002731191273, 0.000000000000000000 ) ) ;
#27869=CARTESIAN_POINT ( 'NONE',  ( 26.29305231718578995, 41.20000000000000284, -19.10302069950538240 ) ) ;
#27873=ORIENTED_EDGE ( 'NONE', *, *, #12800, .F. ) ;
#27874=CARTESIAN_POINT ( 'NONE',  ( -33.58253175000000113, 59.47500000273118559, 10.91162601494193929 ) ) ;
#27879=CARTESIAN_POINT ( 'NONE',  ( 33.58253175000000113, 30.12500000273120193, -4.112674001490185761E-15 ) ) ;
#27893=CARTESIAN_POINT ( 'NONE',  ( 20.08610463437157279, 55.29999999999999716, -27.64615127144129758 ) ) ;
#27894=CARTESIAN_POINT ( 'NONE',  ( -10.04305231718578462, 52.39999999999999147, 30.90933677959249337 ) ) ;
#27900=CARTESIAN_POINT ( 'NONE',  ( -20.75514604977248823, 78.82500000273120122, -28.56700777964554305 ) ) ;
#27901=CARTESIAN_POINT ( 'NONE',  ( 6.486482029760649416E-15, 39.87500000273119127, 35.31076352940723240 ) ) ;
#27907=CARTESIAN_POINT ( 'NONE',  ( -32.50000000000000000, 63.99999999999998579, 0.000000000000000000 ) ) ;
#27912=CARTESIAN_POINT ( 'NONE',  ( 10.37757302488624767, 77.97500000273120691, 31.93888565452638417 ) ) ;
#27917=CARTESIAN_POINT ( 'NONE',  ( 27.16883889988624290, 51.92500000273118843, 19.73931689729373673 ) ) ;
#27918=CARTESIAN_POINT ( 'NONE',  ( 33.58253175000000113, 22.47500000273119625, -10.91162601494193751 ) ) ;
#27929=CARTESIAN_POINT ( 'NONE',  ( 32.50000000000000000, 66.99999999999998579, -3.980102097228898626E-15 ) ) ;
#27941=CARTESIAN_POINT ( 'NONE',  ( 33.58253175000000823, 64.27500000273118985, 10.91162601494192863 ) ) ;
#27949=CARTESIAN_POINT ( 'NONE',  ( 27.16883889988623935, 20.32500000273117280, -19.73931689729374384 ) ) ;
#27951=LINE ( 'NONE', #12331, #21576 ) ;
#27952=LINE ( 'NONE', #9929, #4503 ) ;
#27954=CARTESIAN_POINT ( 'NONE',  ( 20.08610463437158344, 41.20000000546236407, 27.64615127144129403 ) ) ;
#27959=CARTESIAN_POINT ( 'NONE',  ( 33.58253175000000113, 70.12500000273118417, -4.112674001490185761E-15 ) ) ;
#27965=CARTESIAN_POINT ( 'NONE',  ( 27.16883889988623935, 14.32500000273119412, -19.73931689729374384 ) ) ;
#27974=CARTESIAN_POINT ( 'NONE',  ( 10.04305231718578817, 27.39999999999999503, -30.90933677959249337 ) ) ;
#27978=CARTESIAN_POINT ( 'NONE',  ( -17.97732221215932569, 66.99999999999998579, 27.49025280458516463 ) ) ;
#27987=CARTESIAN_POINT ( 'NONE',  ( -10.37757302488623701, 39.52500000273119696, 31.93888565452638417 ) ) ;
#27988=CARTESIAN_POINT ( 'NONE',  ( -27.16883889988624290, 7.175000002731176885, -19.73931689729374028 ) ) ;
#27989=CARTESIAN_POINT ( 'NONE',  ( -2.162160676586882350E-15, 56.87500000273117706, -35.31076352940722529 ) ) ;
#27993=CARTESIAN_POINT ( 'NONE',  ( 26.29305231718578995, 63.70000000546237118, -19.10302069950538240 ) ) ;
#27999=CARTESIAN_POINT ( 'NONE',  ( -27.16883889988624290, 33.17500000273120264, -19.73931689729374028 ) ) ;
#28003=CARTESIAN_POINT ( 'NONE',  ( -10.04305231718578462, 24.90000000546237047, 30.90933677959249337 ) ) ;
#28016=FACE_OUTER_BOUND ( 'NONE', #3817, .T. ) ;
#28021=CARTESIAN_POINT ( 'NONE',  ( -10.04305231718579172, 5.599999999999994316, -30.90933677959248982 ) ) ;
#28027=CARTESIAN_POINT ( 'NONE',  ( 10.37757302488624767, 57.72500000273118559, 31.93888565452638417 ) ) ;
#28028=CARTESIAN_POINT ( 'NONE',  ( 27.16883889988623935, 22.57500000273120122, -19.73931689729374384 ) ) ;
#28029=CARTESIAN_POINT ( 'NONE',  ( -10.37757302488623701, 9.775000002731168536, 31.93888565452638417 ) ) ;
#28034=CARTESIAN_POINT ( 'NONE',  ( 10.37757302488624767, 5.725000002731183812, 31.93888565452638417 ) ) ;
#28036=CARTESIAN_POINT ( 'NONE',  ( 20.08610463437157279, 43.30000000000000426, -27.64615127144129758 ) ) ;
#28043=CARTESIAN_POINT ( 'NONE',  ( 20.75514604977249178, 60.07500000273119412, 28.56700777964553950 ) ) ;
#28044=CARTESIAN_POINT ( 'NONE',  ( 26.29305231718579350, 59.30000000546238681, 19.10302069950537529 ) ) ;
#28048=CARTESIAN_POINT ( 'NONE',  ( 33.58253175000000113, 30.22500000273118559, -10.91162601494193751 ) ) ;
#28061=CARTESIAN_POINT ( 'NONE',  ( 32.50000000000000000, 55.00000000000000711, -3.980102097228898626E-15 ) ) ;
#28068=CARTESIAN_POINT ( 'NONE',  ( -20.75514604977248823, 45.07500000273117990, -28.56700777964554305 ) ) ;
#28073=CARTESIAN_POINT ( 'NONE',  ( 10.04305231718579705, 62.60000000000000142, 30.90933677959248982 ) ) ;
#28078=CARTESIAN_POINT ( 'NONE',  ( 33.58253175000000113, 78.47500000273116427, -10.91162601494193751 ) ) ;
#28083=CARTESIAN_POINT ( 'NONE',  ( -27.16883889988623935, 49.32500000273120122, 19.73931689729374739 ) ) ;
#28084=CARTESIAN_POINT ( 'NONE',  ( 20.75514604977249178, 22.07500000273117990, 28.56700777964553950 ) ) ;
#28086=ORIENTED_EDGE ( 'NONE', *, *, #33257, .T. ) ;
#28089=CARTESIAN_POINT ( 'NONE',  ( 0.000000000000000000, 52.00000000000000711, 0.000000000000000000 ) ) ;
#28109=CARTESIAN_POINT ( 'NONE',  ( 6.486482029760649416E-15, 63.87500000273119127, 35.31076352940723240 ) ) ;
#28115=CARTESIAN_POINT ( 'NONE',  ( -32.50000000000000000, 78.00000000000000000, 0.000000000000000000 ) ) ;
#28116=CARTESIAN_POINT ( 'NONE',  ( -27.16883889988624290, 20.92500000273118843, -19.73931689729374028 ) ) ;
#28121=CARTESIAN_POINT ( 'NONE',  ( -2.092463501923844636E-15, 40.00000000546237544, -34.17252228774368916 ) ) ;
#28127=CARTESIAN_POINT ( 'NONE',  ( -27.16883889988623935, 69.32500000273118701, 19.73931689729374739 ) ) ;
#28134=CARTESIAN_POINT ( 'NONE',  ( 20.75514604977248467, 10.42500000273120087, -28.56700777964554305 ) ) ;
#28145=CARTESIAN_POINT ( 'NONE',  ( -26.29305231718579350, 29.80000000000000782, -19.10302069950537884 ) ) ;
#28153=EDGE_LOOP ( 'NONE', ( #3202, #31671, #1175, #26241 ) ) ;
#28158=CARTESIAN_POINT ( 'NONE',  ( 33.58253175000000113, 38.12500000273118417, -4.112674001490185761E-15 ) ) ;
#28159=CARTESIAN_POINT ( 'NONE',  ( 33.58253175000000113, 4.375000002731193938, -4.112674001490185761E-15 ) ) ;
#28160=CARTESIAN_POINT ( 'NONE',  ( 33.58253175000000113, 54.47500000273117138, -10.91162601494193574 ) ) ;
#28164=CARTESIAN_POINT ( 'NONE',  ( 20.08610463437158344, 59.20000000546237828, 27.64615127144129403 ) ) ;
#28169=LINE ( 'NONE', #20284, #33857 ) ;
#28170=CARTESIAN_POINT ( 'NONE',  ( 10.37757302488624056, 32.77500000273118985, -31.93888565452638417 ) ) ;
#28175=CARTESIAN_POINT ( 'NONE',  ( 32.50000000000000711, 23.40000000546237047, 10.55989012756945122 ) ) ;
#28193=CARTESIAN_POINT ( 'NONE',  ( -33.58253175000000113, 79.37500000273119838, 0.000000000000000000 ) ) ;
#28194=ORIENTED_EDGE ( 'NONE', *, *, #16639, .T. ) ;
#28199=ADVANCED_FACE ( 'NONE', ( #7412 ), #30919, .F. ) ;
#28200=CARTESIAN_POINT ( 'NONE',  ( -27.16883889988623935, 59.32500000273120833, 19.73931689729374739 ) ) ;
#28201=CARTESIAN_POINT ( 'NONE',  ( 33.58253175000000113, 22.37500000273119483, -4.112674001490185761E-15 ) ) ;
#28202=CARTESIAN_POINT ( 'NONE',  ( 33.58253175000000113, 8.475000002731185589, -10.91162601494193751 ) ) ;
#28206=CARTESIAN_POINT ( 'NONE',  ( -33.58253175000000113, 3.025000002731184967, -10.91162601494193218 ) ) ;
#28208=CARTESIAN_POINT ( 'NONE',  ( -10.04305231718578462, 44.40000000000000568, 30.90933677959249337 ) ) ;
#28212=CARTESIAN_POINT ( 'NONE',  ( 27.16883889988623935, 52.57500000273117280, -19.73931689729374384 ) ) ;
#28217=CARTESIAN_POINT ( 'NONE',  ( -20.75514604977248823, 28.82500000273116569, -28.56700777964554305 ) ) ;
#28239=CARTESIAN_POINT ( 'NONE',  ( 33.58253175000000113, 42.47500000273119980, -10.91162601494193751 ) ) ;
#28246=CARTESIAN_POINT ( 'NONE',  ( 20.08610463437157279, 63.30000000000001137, -27.64615127144129758 ) ) ;
#28251=CARTESIAN_POINT ( 'NONE',  ( 33.58253175000000823, 70.27500000273118985, 10.91162601494192863 ) ) ;
#28255=ORIENTED_EDGE ( 'NONE', *, *, #15561, .F. ) ;
#28256=CARTESIAN_POINT ( 'NONE',  ( 27.16883889988623935, 50.32500000273120122, -19.73931689729374384 ) ) ;
#28257=ORIENTED_EDGE ( 'NONE', *, *, #27172, .F. ) ;
#28261=CARTESIAN_POINT ( 'NONE',  ( 10.04305231718578817, 7.900000005462357144, -30.90933677959249337 ) ) ;
#28280=CARTESIAN_POINT ( 'NONE',  ( 6.486482029760649416E-15, 61.87500000273117706, 35.31076352940723240 ) ) ;
#28286=FACE_OUTER_BOUND ( 'NONE', #18489, .T. ) ;
#28287=CARTESIAN_POINT ( 'NONE',  ( -33.58253175000000113, 19.22500000273118204, 10.91162601494193929 ) ) ;
#28291=CARTESIAN_POINT ( 'NONE',  ( -2.092463501923844636E-15, 44.00000000546238965, -34.17252228774368916 ) ) ;
#28297=CARTESIAN_POINT ( 'NONE',  ( -10.37757302488623701, 67.52500000273118985, 31.93888565452638417 ) ) ;
#28303=CARTESIAN_POINT ( 'NONE',  ( -10.37757302488624411, 10.72500000273117493, -31.93888565452638417 ) ) ;
#28312=CARTESIAN_POINT ( 'NONE',  ( 26.29305231718579350, 26.80000000000000426, 19.10302069950537529 ) ) ;
#28326=CARTESIAN_POINT ( 'NONE',  ( 27.16883889988623935, 42.32500000273119412, -19.73931689729374384 ) ) ;
#28328=CARTESIAN_POINT ( 'NONE',  ( 10.37757302488624767, 57.97500000273118559, 31.93888565452638417 ) ) ;
#28334=CARTESIAN_POINT ( 'NONE',  ( 10.04305231718579705, 59.10000000546237686, 30.90933677959248982 ) ) ;
#28342=CARTESIAN_POINT ( 'NONE',  ( -33.58253175000000113, 33.27500000273120406, -10.91162601494193218 ) ) ;
#28346=CARTESIAN_POINT ( 'NONE',  ( 20.08610463437158344, 23.20000000546238539, 27.64615127144129403 ) ) ;
#28356=CARTESIAN_POINT ( 'NONE',  ( -27.16883889988624290, 60.92500000273119554, -19.73931689729374028 ) ) ;
#28366=CARTESIAN_POINT ( 'NONE',  ( 10.37757302488624767, 77.97500000273120691, 31.93888565452638417 ) ) ;
#28371=CARTESIAN_POINT ( 'NONE',  ( -33.58253175000000113, 63.02500000273118985, -10.91162601494193218 ) ) ;
#28372=CARTESIAN_POINT ( 'NONE',  ( -10.37757302488624411, 16.97500000273118204, -31.93888565452638417 ) ) ;
#28373=CARTESIAN_POINT ( 'NONE',  ( 6.486482029760649416E-15, 7.875000002731177950, 35.31076352940723240 ) ) ;
#28377=CARTESIAN_POINT ( 'NONE',  ( -10.37757302488623701, 5.525000002731192517, 31.93888565452638417 ) ) ;
#28379=CARTESIAN_POINT ( 'NONE',  ( -26.29305231718579350, 43.79999999999999005, -19.10302069950537884 ) ) ;
#28384=CARTESIAN_POINT ( 'NONE',  ( -20.75514604977248823, 57.07500000273117280, -28.56700777964554305 ) ) ;
#28389=CARTESIAN_POINT ( 'NONE',  ( -33.58253175000000113, 25.02500000273117209, -10.91162601494193218 ) ) ;
#28392=CARTESIAN_POINT ( 'NONE',  ( -5.147494310547423346, 58.44874571845313938, 32.50000000000000000 ) ) ;
#28402=CARTESIAN_POINT ( 'NONE',  ( 32.50000000000000000, 55.09999999999997300, -10.55989012756945833 ) ) ;
#28403=CARTESIAN_POINT ( 'NONE',  ( 20.08610463437158344, 14.70000000000000107, 27.64615127144129403 ) ) ;
#28409=CARTESIAN_POINT ( 'NONE',  ( -20.75514604977248823, 41.07500000273119412, -28.56700777964554305 ) ) ;
#28414=CARTESIAN_POINT ( 'NONE',  ( 32.50000000000000000, 61.09999999999998721, -10.55989012756945833 ) ) ;
#28419=CARTESIAN_POINT ( 'NONE',  ( 33.58253175000000113, 72.37500000273118417, -4.112674001490185761E-15 ) ) ;
#28425=CARTESIAN_POINT ( 'NONE',  ( 10.37757302488624056, 46.52500000273117564, -31.93888565452638417 ) ) ;
#28429=CARTESIAN_POINT ( 'NONE',  ( -26.29305231718579350, 2.300000005462377040, -19.10302069950537884 ) ) ;
#28446=CARTESIAN_POINT ( 'NONE',  ( 27.16883889988623935, 60.57500000273117990, -19.73931689729374384 ) ) ;
#28450=CARTESIAN_POINT ( 'NONE',  ( 0.000000000000000000, 52.00000000000000711, 0.000000000000000000 ) ) ;
#28454=CARTESIAN_POINT ( 'NONE',  ( -20.75514604977248823, 12.82500000273119589, -28.56700777964554305 ) ) ;
#28459=CARTESIAN_POINT ( 'NONE',  ( -10.04305231718579172, 38.10000000546236265, -30.90933677959248982 ) ) ;
#28464=CARTESIAN_POINT ( 'NONE',  ( -27.16883889988623935, 63.32500000273120833, 19.73931689729374739 ) ) ;
#28469=ORIENTED_EDGE ( 'NONE', *, *, #13461, .F. ) ;
#28470=CARTESIAN_POINT ( 'NONE',  ( 10.37757302488624767, 9.725000002731173154, 31.93888565452638417 ) ) ;
#28480=CARTESIAN_POINT ( 'NONE',  ( -2.092463501923844636E-15, 31.49999999999999289, -34.17252228774368916 ) ) ;
#28489=CARTESIAN_POINT ( 'NONE',  ( 28.18730216971810165, 66.99999999999998579, -16.82255561448983983 ) ) ;
#28490=CARTESIAN_POINT ( 'NONE',  ( -10.37757302488623701, 35.52500000273118985, 31.93888565452638417 ) ) ;
#28491=CARTESIAN_POINT ( 'NONE',  ( -26.29305231718579350, 64.30000000546236549, -19.10302069950537884 ) ) ;
#28495=CARTESIAN_POINT ( 'NONE',  ( 20.08610463437158344, 61.20000000546237118, 27.64615127144129403 ) ) ;
#28501=CARTESIAN_POINT ( 'NONE',  ( -27.16883889988624290, 37.17500000273120264, -19.73931689729374028 ) ) ;
#28505=CARTESIAN_POINT ( 'NONE',  ( -26.29305231718579350, 24.30000000546238326, -19.10302069950537884 ) ) ;
#28518=CARTESIAN_POINT ( 'NONE',  ( 33.58253175000000113, 62.12500000273117706, -4.112674001490185761E-15 ) ) ;
#28528=CARTESIAN_POINT ( 'NONE',  ( -20.75514604977248823, 73.07500000273115859, -28.56700777964554305 ) ) ;
#28533=CARTESIAN_POINT ( 'NONE',  ( -33.58253175000000113, 57.12500000273116996, 0.000000000000000000 ) ) ;
#28534=CARTESIAN_POINT ( 'NONE',  ( -33.58253175000000113, 19.27500000273117919, -10.91162601494193218 ) ) ;
#28535=CARTESIAN_POINT ( 'NONE',  ( -27.16883889988623935, 1.575000002731183457, 19.73931689729374739 ) ) ;
#28539=CARTESIAN_POINT ( 'NONE',  ( 27.16883889988624290, 3.925000002731188431, 19.73931689729373673 ) ) ;
#28540=CARTESIAN_POINT ( 'NONE',  ( 21.25115026575265631, 51.99999999999997158, -25.10892607490231043 ) ) ;
#28545=CARTESIAN_POINT ( 'NONE',  ( -10.37757302488623701, 55.77500000273121117, 31.93888565452638417 ) ) ;
#28551=CARTESIAN_POINT ( 'NONE',  ( 10.37757302488624056, 24.52500000273118275, -31.93888565452638417 ) ) ;
#28566=CARTESIAN_POINT ( 'NONE',  ( 26.29305231718579350, 18.79999999999999716, 19.10302069950537529 ) ) ;
#28572=CARTESIAN_POINT ( 'NONE',  ( 20.75514604977249178, 77.82500000273120122, 28.56700777964553950 ) ) ;
#28574=CARTESIAN_POINT ( 'NONE',  ( 20.75514604977249178, 34.07500000273117990, 28.56700777964553950 ) ) ;
#28580=CARTESIAN_POINT ( 'NONE',  ( -10.04305231718579172, 63.60000000000000142, -30.90933677959248982 ) ) ;
#28584=CARTESIAN_POINT ( 'NONE',  ( 10.37757302488624767, 75.97500000273120691, 31.93888565452638417 ) ) ;
#28589=CARTESIAN_POINT ( 'NONE',  ( 6.486482029760649416E-15, 45.62500000273118417, 35.31076352940723240 ) ) ;
#28592=FACE_OUTER_BOUND ( 'NONE', #2655, .T. ) ;
#28593=CARTESIAN_POINT ( 'NONE',  ( 26.29305231718579350, 5.300000005462379704, 19.10302069950537529 ) ) ;
#28611=CARTESIAN_POINT ( 'NONE',  ( 33.58253175000000823, 58.27500000273116854, 10.91162601494192863 ) ) ;
#28620=CARTESIAN_POINT ( 'NONE',  ( 27.16883889988624290, 15.92500000273118488, 19.73931689729373673 ) ) ;
#28625=CARTESIAN_POINT ( 'NONE',  ( 32.50000000000000000, 37.50000000546237544, -3.980102097228898626E-15 ) ) ;
#28630=CARTESIAN_POINT ( 'NONE',  ( 27.16883889988624290, 63.92500000273120264, 19.73931689729373673 ) ) ;
#28637=CARTESIAN_POINT ( 'NONE',  ( 10.37757302488624056, 4.525000002731191628, -31.93888565452638417 ) ) ;
#28648=CARTESIAN_POINT ( 'NONE',  ( 32.50000000000000711, 30.89999999999998437, 10.55989012756945122 ) ) ;
#28652=CARTESIAN_POINT ( 'NONE',  ( -33.36402495954516922, 67.00000000000002842, 0.4025740098929149191 ) ) ;
#28660=CARTESIAN_POINT ( 'NONE',  ( -2.376701315729135899, 67.00000000000000000, -33.34874525913694754 ) ) ;
#28663=CARTESIAN_POINT ( 'NONE',  ( -20.75514604977248112, 35.42500000273119554, 28.56700777964554661 ) ) ;
#28670=CARTESIAN_POINT ( 'NONE',  ( 10.04305231718579705, 55.10000000546237686, 30.90933677959248982 ) ) ;
#28676=CARTESIAN_POINT ( 'NONE',  ( 20.75514604977249178, 34.07500000273117990, 28.56700777964553950 ) ) ;
#28680=CARTESIAN_POINT ( 'NONE',  ( -32.50000000000000000, 20.60000000546237686, 10.55989012756946366 ) ) ;
#28691=CARTESIAN_POINT ( 'NONE',  ( -33.58253175000000113, 63.22500000273119269, 10.91162601494193929 ) ) ;
#28701=CARTESIAN_POINT ( 'NONE',  ( 33.58253175000000113, 76.37500000273118417, -4.112674001490185761E-15 ) ) ;
#28705=CARTESIAN_POINT ( 'NONE',  ( 33.58253175000000113, 52.22500000273117848, -10.91162601494193751 ) ) ;
#28706=CARTESIAN_POINT ( 'NONE',  ( 27.16883889988624290, 16.17500000273118488, 19.73931689729373673 ) ) ;
#28707=CARTESIAN_POINT ( 'NONE',  ( -27.16883889988624290, 78.92500000273118133, -19.73931689729374028 ) ) ;
#28711=CARTESIAN_POINT ( 'NONE',  ( 26.29305231718579350, 73.30000000546236549, 19.10302069950537529 ) ) ;
#28719=CARTESIAN_POINT ( 'NONE',  ( -2.162160676586881955E-15, 56.87500000273117706, -35.31076352940723240 ) ) ;
#28725=CARTESIAN_POINT ( 'NONE',  ( 10.37757302488624056, 26.52500000273118275, -31.93888565452638417 ) ) ;
#28734=CARTESIAN_POINT ( 'NONE',  ( -20.08610463437157989, 63.69999999999999574, -27.64615127144129758 ) ) ;
#28739=CARTESIAN_POINT ( 'NONE',  ( -32.50000000000000000, 16.10000000000001563, 10.55989012756946366 ) ) ;
#28745=CARTESIAN_POINT ( 'NONE',  ( 27.16883889988623935, 70.32500000273118701, -19.73931689729374384 ) ) ;
#28746=CARTESIAN_POINT ( 'NONE',  ( -33.58253175000000113, 33.47500000273119269, 10.91162601494193929 ) ) ;
#28753=CARTESIAN_POINT ( 'NONE',  ( -20.08610463437157989, 57.70000000000000284, -27.64615127144129758 ) ) ;
#28759=CARTESIAN_POINT ( 'NONE',  ( 33.58253175000000823, 72.27500000273118985, 10.91162601494192863 ) ) ;
#28764=CARTESIAN_POINT ( 'NONE',  ( -10.37757302488623701, 41.52500000273119696, 31.93888565452638417 ) ) ;
#28768=CARTESIAN_POINT ( 'NONE',  ( 20.08610463437158344, 7.200000005462378283, 27.64615127144129403 ) ) ;
#28785=CARTESIAN_POINT ( 'NONE',  ( -10.37757302488623701, 53.77500000273120406, 31.93888565452638417 ) ) ;
#28789=DIRECTION ( 'NONE',  ( 0.000000000000000000, 0.000000000000000000, 1.000000000000000000 ) ) ;
#28791=CARTESIAN_POINT ( 'NONE',  ( -10.04305231718579172, 79.59999999999999432, -30.90933677959248982 ) ) ;
#28792=CARTESIAN_POINT ( 'NONE',  ( -20.75514604977248823, 14.82500000273117635, -28.56700777964554305 ) ) ;
#28798=CARTESIAN_POINT ( 'NONE',  ( -10.04305231718579172, 36.10000000546239107, -30.90933677959248982 ) ) ;
#28804=CARTESIAN_POINT ( 'NONE',  ( -33.58253175000000113, 61.12500000273117706, 0.000000000000000000 ) ) ;
#28809=CARTESIAN_POINT ( 'NONE',  ( 33.58253175000000113, 6.125000002731181503, -4.112674001490185761E-15 ) ) ;
#28819=CARTESIAN_POINT ( 'NONE',  ( -10.04305231718579172, 21.59999999999999432, -30.90933677959248982 ) ) ;
#28823=CARTESIAN_POINT ( 'NONE',  ( -24.23786831611838011, 66.99999999999998579, 22.37122307655967290 ) ) ;
#28831=CARTESIAN_POINT ( 'NONE',  ( 20.75514604977249178, 35.82500000273117990, 28.56700777964553950 ) ) ;
#28836=CARTESIAN_POINT ( 'NONE',  ( -26.29305231718579350, 54.30000000546237970, -19.10302069950537884 ) ) ;
#28843=CARTESIAN_POINT ( 'NONE',  ( -33.58253175000000113, 25.37500000273119838, 0.000000000000000000 ) ) ;
#28847=CARTESIAN_POINT ( 'NONE',  ( -20.08610463437156923, 16.80000000546237970, 27.64615127144130113 ) ) ;
#28849=CARTESIAN_POINT ( 'NONE',  ( 12.90513655866702081, 52.00000000000000711, 31.00393344628893288 ) ) ;
#28859=CARTESIAN_POINT ( 'NONE',  ( 20.75514604977249178, 61.82500000273117280, 28.56700777964553950 ) ) ;
#28864=CARTESIAN_POINT ( 'NONE',  ( 3.980102097228898626E-15, 52.00000000000000711, -32.50000000000000000 ) ) ;
#28869=CARTESIAN_POINT ( 'NONE',  ( -27.16883889988623935, 77.57500000273120122, 19.73931689729374739 ) ) ;
#28871=CIRCLE ( 'NONE', #33802, 32.50000000000000000 ) ;
#28874=CARTESIAN_POINT ( 'NONE',  ( -27.16883889988624290, 52.92500000273118843, -19.73931689729374028 ) ) ;
#28875=CARTESIAN_POINT ( 'NONE',  ( 27.16883889988624290, 14.17500000273118310, 19.73931689729373673 ) ) ;
#28876=CARTESIAN_POINT ( 'NONE',  ( 33.58253175000000113, 6.375000002731182391, -4.112674001490185761E-15 ) ) ;
#28880=CARTESIAN_POINT ( 'NONE',  ( 20.08610463437158344, 71.20000000546237118, 27.64615127144129403 ) ) ;
#28881=CARTESIAN_POINT ( 'NONE',  ( 5.485887633599118468E-07, 52.00000000000003553, -32.49999999999999289 ) ) ;
#28886=CARTESIAN_POINT ( 'NONE',  ( 6.486482029760649416E-15, 51.87500000273119127, 35.31076352940723240 ) ) ;
#28891=CARTESIAN_POINT ( 'NONE',  ( -33.58253175000000113, 21.22500000273117848, 10.91162601494193929 ) ) ;
#28901=CARTESIAN_POINT ( 'NONE',  ( -1.053607264507113999E-13, 64.50000000000000000, 32.50000000000000711 ) ) ;
#28905=CARTESIAN_POINT ( 'NONE',  ( 20.08610463437157279, 17.30000000000000782, -27.64615127144129758 ) ) ;
#28911=CARTESIAN_POINT ( 'NONE',  ( -2.162160676586881955E-15, 72.62500000273118417, -35.31076352940723240 ) ) ;
#28912=CARTESIAN_POINT ( 'NONE',  ( 20.75514604977249178, 38.07500000273116569, 28.56700777964553950 ) ) ;
#28919=CARTESIAN_POINT ( 'NONE',  ( -32.50000000000000000, 52.00000000000000711, 0.000000000000000000 ) ) ;
#28923=VECTOR ( 'NONE', #1331, 1000.000000000000000 ) ;
#28925=CARTESIAN_POINT ( 'NONE',  ( -20.75514604977248823, 71.07500000273117280, -28.56700777964554305 ) ) ;
#28930=CARTESIAN_POINT ( 'NONE',  ( -2.162160676586881955E-15, 40.62500000273120548, -35.31076352940723240 ) ) ;
#28935=CARTESIAN_POINT ( 'NONE',  ( -2.092463501923844636E-15, 6.000000005462371888, -34.17252228774368916 ) ) ;
#28957=CARTESIAN_POINT ( 'NONE',  ( -20.75514604977248112, 55.67500000273118843, 28.56700777964554661 ) ) ;
#28963=CARTESIAN_POINT ( 'NONE',  ( -20.08610463437157989, 73.70000000000000284, -27.64615127144129758 ) ) ;
#28964=CARTESIAN_POINT ( 'NONE',  ( 27.16883889988624290, 13.92500000273118310, 19.73931689729373673 ) ) ;
#28968=CARTESIAN_POINT ( 'NONE',  ( -2.092463501923844636E-15, 38.00000000546237544, -34.17252228774368916 ) ) ;
#28973=CARTESIAN_POINT ( 'NONE',  ( -2.162160676586881955E-15, 60.62500000273117706, -35.31076352940723240 ) ) ;
#28977=CARTESIAN_POINT ( 'NONE',  ( 6.486482029760649416E-15, 5.625000002731175286, 35.31076352940723240 ) ) ;
#28987=CARTESIAN_POINT ( 'NONE',  ( -10.04305231718578462, 24.39999999999999147, 30.90933677959249337 ) ) ;
#28991=CARTESIAN_POINT ( 'NONE',  ( -31.78338918835712334, 66.99999999999997158, 9.699108655006819291 ) ) ;
#28998=CARTESIAN_POINT ( 'NONE',  ( 20.75514604977249178, 37.82500000273117280, 28.56700777964553950 ) ) ;
#29000=CARTESIAN_POINT ( 'NONE',  ( 21.62020457442521248, 52.08848768517668049, 27.37635686616407327 ) ) ;
#29003=CARTESIAN_POINT ( 'NONE',  ( 32.50000000000000000, 57.50000000546238965, -3.980102097228898626E-15 ) ) ;
#29010=CARTESIAN_POINT ( 'NONE',  ( 33.58253175000000113, 28.47500000273118204, -10.91162601494193751 ) ) ;
#29014=CARTESIAN_POINT ( 'NONE',  ( 26.29305231718578995, 15.70000000546238539, -19.10302069950538240 ) ) ;
#29023=CARTESIAN_POINT ( 'NONE',  ( -10.37757302488623701, 59.52500000273118275, 31.93888565452638417 ) ) ;
#29033=CARTESIAN_POINT ( 'NONE',  ( 33.58253175000000113, 72.37500000273118417, -4.112674001490185761E-15 ) ) ;
#29034=ORIENTED_EDGE ( 'NONE', *, *, #30108, .T. ) ;
#29037=CARTESIAN_POINT ( 'NONE',  ( 33.58253175000000113, 54.12500000273119838, -4.112674001490185761E-15 ) ) ;
#29038=CARTESIAN_POINT ( 'NONE',  ( 6.486482029760649416E-15, 15.87500000273120015, 35.31076352940723240 ) ) ;
#29039=CARTESIAN_POINT ( 'NONE',  ( 20.75514604977249178, 6.075000002731190563, 28.56700777964553950 ) ) ;
#29043=CARTESIAN_POINT ( 'NONE',  ( 20.08610463437158344, 75.20000000546241381, 27.64615127144129403 ) ) ;
#29050=CARTESIAN_POINT ( 'NONE',  ( 20.75514604977249178, 46.07500000273117280, 28.56700777964553950 ) ) ;
#29055=CARTESIAN_POINT ( 'NONE',  ( 10.37757302488624056, 18.52500000273120406, -31.93888565452638417 ) ) ;
#29067=DIRECTION ( 'NONE',  ( 0.000000000000000000, 1.000000000000000000, 0.000000000000000000 ) ) ;
#29068=CARTESIAN_POINT ( 'NONE',  ( 20.08610463437158344, 65.20000000546235697, 27.64615127144129403 ) ) ;
#29070=EDGE_CURVE ( 'NONE', #1729, #21053, #22499, .T. ) ;
#29071=CARTESIAN_POINT ( 'NONE',  ( 20.08610463437157279, 19.30000000000000426, -27.64615127144129758 ) ) ;
#29077=CARTESIAN_POINT ( 'NONE',  ( -27.16883889988623935, 73.32500000273118701, 19.73931689729374739 ) ) ;
#29078=CARTESIAN_POINT ( 'NONE',  ( 20.75514604977248467, 38.67500000273117422, -28.56700777964554305 ) ) ;
#29084=CARTESIAN_POINT ( 'NONE',  ( -10.04305231718578462, 52.39999999999999147, 30.90933677959249337 ) ) ;
#29089=CARTESIAN_POINT ( 'NONE',  ( 33.58253175000000113, 66.47500000273119269, -10.91162601494193751 ) ) ;
#29094=CARTESIAN_POINT ( 'NONE',  ( 27.16883889988623935, 46.32500000273119412, -19.73931689729374384 ) ) ;
#29098=CARTESIAN_POINT ( 'NONE',  ( -10.04305231718579172, 60.10000000546238397, -30.90933677959248982 ) ) ;
#29099=CARTESIAN_POINT ( 'NONE',  ( -32.50000000000000000, 6.600000005462382191, 10.55989012756946366 ) ) ;
#29115=CARTESIAN_POINT ( 'NONE',  ( 0.000000000000000000, 52.00000000000000711, 0.000000000000000000 ) ) ;
#29117=( BOUNDED_CURVE ( )  B_SPLINE_CURVE ( 2, ( #25373, #30507, #4264, #14738, #32902, #7176, #24857, #27778, #20404, #3929, #27604, #17150, #1677 ),
 .UNSPECIFIED., .F., .T. ) 
 B_SPLINE_CURVE_WITH_KNOTS ( ( 3, 2, 2, 2, 2, 2, 3 ),
 ( 0.3397435897435897578, 0.3410256410256410353, 0.3435897435897435903, 0.3461538461538461453, 0.3487179487179487003, 0.3512820512820512553, 0.3525641025641025883 ),
 .UNSPECIFIED. ) 
 CURVE ( )  GEOMETRIC_REPRESENTATION_ITEM ( )  RATIONAL_B_SPLINE_CURVE ( ( 0.9755282581475768211, 0.9755282581475768211, 1.000000000000000000, 0.9510565162951535312, 1.000000000000000000, 0.9510565162951535312, 1.000000000000000000, 0.9510565162951535312, 1.000000000000000000, 0.9510565162951535312, 1.000000000000000000, 0.9755282581475762660, 0.9755282581475768211 ) ) 
 REPRESENTATION_ITEM ( '' )  );
#29120=CARTESIAN_POINT ( 'NONE',  ( 6.486482029760649416E-15, 57.87500000273117706, 35.31076352940723240 ) ) ;
#29126=CARTESIAN_POINT ( 'NONE',  ( -2.092463501923844636E-15, 73.49999999999998579, -34.17252228774368916 ) ) ;
#29127=CARTESIAN_POINT ( 'NONE',  ( 33.58253175000000823, 18.02500000273118630, 10.91162601494192863 ) ) ;
#29136=CARTESIAN_POINT ( 'NONE',  ( 33.58253175000000113, 60.22500000273119980, -10.91162601494193751 ) ) ;
#29140=CARTESIAN_POINT ( 'NONE',  ( -33.58253175000000113, 7.125000002731182391, 0.000000000000000000 ) ) ;
#29146=CARTESIAN_POINT ( 'NONE',  ( -20.08610463437156923, 52.80000000546237260, 27.64615127144130113 ) ) ;
#29148=CARTESIAN_POINT ( 'NONE',  ( 32.50000000000000000, 25.00000000000000711, -3.980102097228898626E-15 ) ) ;
#29152=CARTESIAN_POINT ( 'NONE',  ( -33.24513298742183309, 66.99999999999998579, 2.427281437204855230 ) ) ;
#29159=CARTESIAN_POINT ( 'NONE',  ( 19.22940031075280132, 66.99999999999994316, -26.85591229561295989 ) ) ;
#29160=CARTESIAN_POINT ( 'NONE',  ( -22.34582402162608616, 52.00000000000002842, 24.25905220314540500 ) ) ;
#29161=CARTESIAN_POINT ( 'NONE',  ( 27.16883889988624290, 31.92500000273119909, 19.73931689729373673 ) ) ;
#29163=CARTESIAN_POINT ( 'NONE',  ( -1.778240108872766143E-15, 65.50000000000000000, -32.49999999999999289 ) ) ;
#29167=CARTESIAN_POINT ( 'NONE',  ( 32.50000000000000711, 57.40000000546237402, 10.55989012756945122 ) ) ;
#29170=( LENGTH_UNIT ( ) NAMED_UNIT ( * ) SI_UNIT ( .MILLI., .METRE. ) );
#29173=EDGE_CURVE ( 'NONE', #679, #20850, #26, .T. ) ;
#29177=CARTESIAN_POINT ( 'NONE',  ( -10.37757302488623701, 25.77500000273118275, 31.93888565452638417 ) ) ;
#29181=CARTESIAN_POINT ( 'NONE',  ( 32.50000000000000711, 19.40000000546238468, 10.55989012756945122 ) ) ;
#29191=CARTESIAN_POINT ( 'NONE',  ( 33.58253175000000823, 52.06397437591922994, 6.658888170994894828 ) ) ;
#29202=CARTESIAN_POINT ( 'NONE',  ( -27.16883889988623935, 65.57500000273118701, 19.73931689729374739 ) ) ;
#29206=CARTESIAN_POINT ( 'NONE',  ( -20.75514604977248112, 55.42500000273119554, 28.56700777964554661 ) ) ;
#29207=CARTESIAN_POINT ( 'NONE',  ( 33.58253175000000113, 12.47500000273119447, -10.91162601494193751 ) ) ;
#29208=CARTESIAN_POINT ( 'NONE',  ( 33.58253175000000823, 6.275000002731184523, 10.91162601494192863 ) ) ;
#29212=CARTESIAN_POINT ( 'NONE',  ( -26.29305231718579350, 74.30000000546236549, -19.10302069950537884 ) ) ;
#29219=CARTESIAN_POINT ( 'NONE',  ( -10.37757302488623701, 47.77500000273120406, 31.93888565452638417 ) ) ;
#29224=CARTESIAN_POINT ( 'NONE',  ( 6.486482029760649416E-15, 17.62500000273117351, 35.31076352940723240 ) ) ;
#29232=CARTESIAN_POINT ( 'NONE',  ( 40.00000000000000000, 52.00000000000000711, -23.09401076758505766 ) ) ;
#29239=CARTESIAN_POINT ( 'NONE',  ( -20.08610463437157989, 59.70000000000000284, -27.64615127144129758 ) ) ;
#29240=CARTESIAN_POINT ( 'NONE',  ( 10.04305231718578817, 7.400000000000003908, -30.90933677959249337 ) ) ;
#29246=CARTESIAN_POINT ( 'NONE',  ( 33.58253175000000113, 76.22500000273119269, -10.91162601494193751 ) ) ;
#29247=CARTESIAN_POINT ( 'NONE',  ( -10.37757302488624411, 38.97500000273117138, -31.93888565452638417 ) ) ;
#29253=CARTESIAN_POINT ( 'NONE',  ( -32.50000000000000000, 52.10000000000001563, 10.55989012756946366 ) ) ;
#29258=CARTESIAN_POINT ( 'NONE',  ( -10.37757302488623701, 67.77500000273118985, 31.93888565452638417 ) ) ;
#29264=CARTESIAN_POINT ( 'NONE',  ( 33.58253175000000113, 36.22500000273119980, -10.91162601494193751 ) ) ;
#29266=VERTEX_POINT ( 'NONE', #2961 ) ;
#29268=CARTESIAN_POINT ( 'NONE',  ( -1.778240108872766143E-15, 53.50000000000000000, -32.49999999999999289 ) ) ;
#29288=CARTESIAN_POINT ( 'NONE',  ( 27.16883889988624290, 56.17500000273119554, 19.73931689729373673 ) ) ;
#29296=CARTESIAN_POINT ( 'NONE',  ( -10.04305231718579172, 71.59999999999998010, -30.90933677959248982 ) ) ;
#29297=CARTESIAN_POINT ( 'NONE',  ( 33.58253175000000113, 6.125000002731181503, -4.112674001490185761E-15 ) ) ;
#29299=CARTESIAN_POINT ( 'NONE',  ( 0.000000000000000000, 52.00000000000000711, 0.000000000000000000 ) ) ;
#29305=CARTESIAN_POINT ( 'NONE',  ( 33.58253175000000113, 58.12500000273116996, -4.112674001490185761E-15 ) ) ;
#29309=CARTESIAN_POINT ( 'NONE',  ( -27.16883889988624290, 4.925000002731189319, -19.73931689729374028 ) ) ;
#29314=( BOUNDED_CURVE ( )  B_SPLINE_CURVE ( 2, ( #23144, #31034, #7530, #4951, #2380, #635, #19516, #13866, #29964, #16610, #29464, #32537, #14030 ),
 .UNSPECIFIED., .F., .T. ) 
 B_SPLINE_CURVE_WITH_KNOTS ( ( 3, 2, 2, 2, 2, 2, 3 ),
 ( 0.1730769230769230727, 0.1743589743589743501, 0.1769230769230769329, 0.1794871794871794879, 0.1820512820512820429, 0.1846153846153846256, 0.1858974358974359031 ),
 .UNSPECIFIED. ) 
 CURVE ( )  GEOMETRIC_REPRESENTATION_ITEM ( )  RATIONAL_B_SPLINE_CURVE ( ( 0.9755282581475768211, 0.9755282581475768211, 1.000000000000000000, 0.9510565162951535312, 1.000000000000000000, 0.9510565162951535312, 1.000000000000000000, 0.9510565162951535312, 1.000000000000000000, 0.9510565162951535312, 1.000000000000000000, 0.9755282581475768211, 0.9755282581475768211 ) ) 
 REPRESENTATION_ITEM ( '' )  );
#29320=CARTESIAN_POINT ( 'NONE',  ( 26.29305231718579350, 22.80000000000000071, 19.10302069950537529 ) ) ;
#29333=CARTESIAN_POINT ( 'NONE',  ( -29.41736854754604380, 52.00000000000000000, 14.41477566699508195 ) ) ;
#29334=CARTESIAN_POINT ( 'NONE',  ( 10.37757302488624767, 25.72500000273118914, 31.93888565452638417 ) ) ;
#29337=CARTESIAN_POINT ( 'NONE',  ( 32.50000000000000000, 60.99999999999998579, -3.980102097228898626E-15 ) ) ;
#29339=CARTESIAN_POINT ( 'NONE',  ( 26.29305231718578995, 57.70000000546237118, -19.10302069950538240 ) ) ;
#29340=COLOUR_RGB ( '', 0.72549020, 0.75294118, 0.79215686) ;
#29342=CARTESIAN_POINT ( 'NONE',  ( -20.08610463437157989, 58.20000000546238539, -27.64615127144129758 ) ) ;
#29350=CARTESIAN_POINT ( 'NONE',  ( -20.08610463437156923, 18.80000000546237615, 27.64615127144130113 ) ) ;
#29360=CARTESIAN_POINT ( 'NONE',  ( -20.75514604977248112, 53.42500000273117422, 28.56700777964554661 ) ) ;
#29365=CARTESIAN_POINT ( 'NONE',  ( -26.29305231718578995, 66.70000000546237118, 19.10302069950538595 ) ) ;
#29370=CARTESIAN_POINT ( 'NONE',  ( 20.75514604977249178, 68.07500000273118701, 28.56700777964553950 ) ) ;
#29371=ORIENTED_EDGE ( 'NONE', *, *, #8471, .F. ) ;
#29376=CARTESIAN_POINT ( 'NONE',  ( -33.58253175000000113, 45.12500000273119127, 0.000000000000000000 ) ) ;
#29377=CARTESIAN_POINT ( 'NONE',  ( 20.75514604977248467, 8.675000002731195536, -28.56700777964554305 ) ) ;
#29378=CARTESIAN_POINT ( 'NONE',  ( -33.58253175000000113, 65.47500000273117848, 10.91162601494193929 ) ) ;
#29382=CARTESIAN_POINT ( 'NONE',  ( -32.50000000000000000, 72.50000000546238255, 0.000000000000000000 ) ) ;
#29389=CARTESIAN_POINT ( 'NONE',  ( 27.16883889988623935, 48.57500000273119412, -19.73931689729374384 ) ) ;
#29394=CARTESIAN_POINT ( 'NONE',  ( -33.58253175000000113, 19.02500000273118630, -10.91162601494193218 ) ) ;
#29404=CARTESIAN_POINT ( 'NONE',  ( -32.50000000000000000, 63.89999999999998437, -10.55989012756945300 ) ) ;
#29408=CARTESIAN_POINT ( 'NONE',  ( -20.08610463437156923, 8.300000000000000711, 27.64615127144130113 ) ) ;
#29415=CARTESIAN_POINT ( 'NONE',  ( 20.75514604977248467, 74.42500000273119554, -28.56700777964554305 ) ) ;
#29416=CARTESIAN_POINT ( 'NONE',  ( 20.75514604977248467, 28.67500000273117777, -28.56700777964554305 ) ) ;
#29422=CARTESIAN_POINT ( 'NONE',  ( 26.29305231718579350, 56.80000000000000426, 19.10302069950537529 ) ) ;
#29423=CARTESIAN_POINT ( 'NONE',  ( 1.076200423132605543E-16, 66.99999999999998579, -46.18802153517007980 ) ) ;
#29427=CARTESIAN_POINT ( 'NONE',  ( 33.58253175000000823, 64.27500000273118985, 10.91162601494192863 ) ) ;
#29428=CARTESIAN_POINT ( 'NONE',  ( -32.50000000000000000, 61.99999999999998579, 0.000000000000000000 ) ) ;
#29432=CARTESIAN_POINT ( 'NONE',  ( 20.75514604977249178, 39.82500000273116569, 28.56700777964553950 ) ) ;
#29453=CARTESIAN_POINT ( 'NONE',  ( -27.16883889988624290, 47.17500000273118843, -19.73931689729374028 ) ) ;
#29459=CARTESIAN_POINT ( 'NONE',  ( -10.04305231718578462, 76.40000000000000568, 30.90933677959249337 ) ) ;
#29460=CARTESIAN_POINT ( 'NONE',  ( -33.58253175000000113, 9.025000002731184523, -10.91162601494193218 ) ) ;
#29464=CARTESIAN_POINT ( 'NONE',  ( -10.04305231718579172, 65.60000000000000853, -30.90933677959248982 ) ) ;
#29468=CARTESIAN_POINT ( 'NONE',  ( -33.58253175000000113, 59.02500000273120406, -10.91162601494193218 ) ) ;
#29475=VECTOR ( 'NONE', #29067, 1000.000000000000000 ) ;
#29481=CARTESIAN_POINT ( 'NONE',  ( -32.50000000000000000, 22.00000000000000711, 0.000000000000000000 ) ) ;
#29494=CARTESIAN_POINT ( 'NONE',  ( -10.37757302488624411, 28.72500000273118914, -31.93888565452638417 ) ) ;
#29495=CARTESIAN_POINT ( 'NONE',  ( 5.147494310547434893, 61.05125428700922185, 32.49999999999999289 ) ) ;
#29499=CARTESIAN_POINT ( 'NONE',  ( -20.08610463437157989, 46.20000000546237828, -27.64615127144129758 ) ) ;
#29503=CARTESIAN_POINT ( 'NONE',  ( 10.37757302488624056, 76.52500000273120406, -31.93888565452638417 ) ) ;
#29509=CARTESIAN_POINT ( 'NONE',  ( 20.08610463437157279, 15.80000000546238326, -27.64615127144129758 ) ) ;
#29518=FILL_AREA_STYLE_COLOUR ( '', #29340 ) ;
#29526=CARTESIAN_POINT ( 'NONE',  ( -2.162160676586881955E-15, 68.87500000273118417, -35.31076352940723240 ) ) ;
#29531=CARTESIAN_POINT ( 'NONE',  ( -2.162160676586881955E-15, 44.62500000273119838, -35.31076352940723240 ) ) ;
#29532=CARTESIAN_POINT ( 'NONE',  ( -33.58253175000000113, 11.27500000273118630, -10.91162601494193218 ) ) ;
#29533=CARTESIAN_POINT ( 'NONE',  ( 33.58253175000000113, 62.47500000273118559, -10.91162601494193574 ) ) ;
#29537=CARTESIAN_POINT ( 'NONE',  ( 32.50000000000000000, 65.60000000546237686, -10.55989012756945833 ) ) ;
#29544=CARTESIAN_POINT ( 'NONE',  ( -20.75514604977248823, 49.07500000273117280, -28.56700777964554305 ) ) ;
#29549=ORIENTED_EDGE ( 'NONE', *, *, #20791, .F. ) ;
#29550=CARTESIAN_POINT ( 'NONE',  ( -33.58253175000000113, 15.22500000273119447, 10.91162601494193929 ) ) ;
#29564=CARTESIAN_POINT ( 'NONE',  ( -32.50000000000000000, 7.999999999999992895, 0.000000000000000000 ) ) ;
#29565=ORIENTED_EDGE ( 'NONE', *, *, #29173, .T. ) ;
#29570=CARTESIAN_POINT ( 'NONE',  ( -27.16883889988624290, 64.92500000273119554, -19.73931689729374028 ) ) ;
#29571=CARTESIAN_POINT ( 'NONE',  ( -33.58253175000000113, 31.27500000273118275, -10.91162601494193218 ) ) ;
#29572=CARTESIAN_POINT ( 'NONE',  ( 27.16883889988624290, 14.17500000273118310, 19.73931689729373673 ) ) ;
#29579=CARTESIAN_POINT ( 'NONE',  ( -26.29305231718578995, 54.20000000000000995, 19.10302069950538595 ) ) ;
#29585=CARTESIAN_POINT ( 'NONE',  ( 6.486482029760649416E-15, 65.87500000273119838, 35.31076352940723240 ) ) ;
#29591=CARTESIAN_POINT ( 'NONE',  ( -33.58253175000000113, 37.12500000273118417, 0.000000000000000000 ) ) ;
#29595=CARTESIAN_POINT ( 'NONE',  ( -26.29305231718579350, 60.30000000546238681, -19.10302069950537884 ) ) ;
#29608=CARTESIAN_POINT ( 'NONE',  ( 32.50000000000000000, 53.60000000546238397, -10.55989012756945833 ) ) ;
#29612=CARTESIAN_POINT ( 'NONE',  ( 27.16883889988623935, 46.57500000273119412, -19.73931689729374384 ) ) ;
#29618=CARTESIAN_POINT ( 'NONE',  ( 26.29305231718578995, 73.20000000000000284, -19.10302069950538240 ) ) ;
#29619=CARTESIAN_POINT ( 'NONE',  ( 33.58253175000000113, 12.12500000273118772, -4.112674001490185761E-15 ) ) ;
#29627=VERTEX_POINT ( 'NONE', #20376 ) ;
#29628=CARTESIAN_POINT ( 'NONE',  ( 10.37757302488624056, 56.52500000273118275, -31.93888565452638417 ) ) ;
#29654=CARTESIAN_POINT ( 'NONE',  ( 7.738208025867137962, 52.00000000000001421, 32.61747650539062704 ) ) ;
#29655=CARTESIAN_POINT ( 'NONE',  ( -2.162160676586881955E-15, 26.62500000273118417, -35.31076352940723240 ) ) ;
#29658=AXIS2_PLACEMENT_3D ( 'NONE', #3525, #18657, #21731 ) ;
#29659=CARTESIAN_POINT ( 'NONE',  ( -1.778240108872766143E-15, 62.00000000546238255, -32.49999999999999289 ) ) ;
#29662=CARTESIAN_POINT ( 'NONE',  ( -20.08610463437156923, 50.80000000546237970, 27.64615127144130113 ) ) ;
#29666=CARTESIAN_POINT ( 'NONE',  ( -33.58253175000000113, 75.02500000273117564, -10.91162601494193218 ) ) ;
#29669=EDGE_LOOP ( 'NONE', ( #17693, #19088, #1480, #20118 ) ) ;
#29671=CARTESIAN_POINT ( 'NONE',  ( 26.29305231718578995, 7.700000005462379171, -19.10302069950538240 ) ) ;
#29681=ADVANCED_FACE ( 'NONE', ( #30649 ), #33224, .F. ) ;
#29690=CARTESIAN_POINT ( 'NONE',  ( -10.37757302488624411, 66.97500000273119269, -31.93888565452638417 ) ) ;
#29694=LINE ( 'NONE', #16512, #31610 ) ;
#29696=CARTESIAN_POINT ( 'NONE',  ( 6.486482029760649416E-15, 45.62500000273118417, 35.31076352940723240 ) ) ;
#29697=CARTESIAN_POINT ( 'NONE',  ( 33.58253175000000823, 10.27500000273117564, 10.91162601494192863 ) ) ;
#29698=CARTESIAN_POINT ( 'NONE',  ( -33.58253175000000113, 63.37500000273120548, 0.000000000000000000 ) ) ;
#29700=( BOUNDED_CURVE ( )  B_SPLINE_CURVE ( 2, ( #406, #5570, #8300, #11063, #26506, #21699, #18792, #29404, #5906, #28734, #31480, #16383, #16052 ),
 .UNSPECIFIED., .F., .T. ) 
 B_SPLINE_CURVE_WITH_KNOTS ( ( 3, 2, 2, 2, 2, 2, 3 ),
 ( 0.1987179487179487336, 0.2000000000000000111, 0.2025641025641025661, 0.2051282051282051211, 0.2076923076923077038, 0.2102564102564102588, 0.2115384615384615363 ),
 .UNSPECIFIED. ) 
 CURVE ( )  GEOMETRIC_REPRESENTATION_ITEM ( )  RATIONAL_B_SPLINE_CURVE ( ( 0.9755282581475768211, 0.9755282581475770431, 1.000000000000000000, 0.9510565162951535312, 1.000000000000000000, 0.9510565162951535312, 1.000000000000000000, 0.9510565162951535312, 1.000000000000000000, 0.9510565162951535312, 1.000000000000000000, 0.9755282581475768211, 0.9755282581475768211 ) ) 
 REPRESENTATION_ITEM ( '' )  );
#29703=CARTESIAN_POINT ( 'NONE',  ( -10.04305231718579172, 68.10000000546239107, -30.90933677959248982 ) ) ;
#29710=CARTESIAN_POINT ( 'NONE',  ( -33.58253175000000113, 45.47500000273119980, 10.91162601494193929 ) ) ;
#29715=CARTESIAN_POINT ( 'NONE',  ( 6.486482029760649416E-15, 15.62500000273117884, 35.31076352940723240 ) ) ;
#29732=CARTESIAN_POINT ( 'NONE',  ( -32.50000000000000000, 10.10000000000000142, 10.55989012756946366 ) ) ;
#29739=CARTESIAN_POINT ( 'NONE',  ( 20.75514604977249178, 69.82500000273118701, 28.56700777964553950 ) ) ;
#29740=CARTESIAN_POINT ( 'NONE',  ( -27.16883889988624290, 31.17500000273119909, -19.73931689729374028 ) ) ;
#29741=CARTESIAN_POINT ( 'NONE',  ( 10.37757302488624056, 16.77500000273117564, -31.93888565452638417 ) ) ;
#29747=CARTESIAN_POINT ( 'NONE',  ( 20.08610463437158344, 50.69999999999999574, 27.64615127144129403 ) ) ;
#29748=DIRECTION ( 'NONE',  ( -0.8660254037844385966, 0.000000000000000000, 0.5000000000000000000 ) ) ;
#29753=CARTESIAN_POINT ( 'NONE',  ( -33.58253175000000113, 69.47500000273116427, 10.91162601494193929 ) ) ;
#29754=CARTESIAN_POINT ( 'NONE',  ( -1.053607264507113999E-13, 63.00000000546238255, 32.50000000000000711 ) ) ;
#29758=CARTESIAN_POINT ( 'NONE',  ( 33.58253175000000823, 34.02500000273118275, 10.91162601494192863 ) ) ;
#29776=CARTESIAN_POINT ( 'NONE',  ( -32.50000000000000000, 54.40000000546238823, -10.55989012756945300 ) ) ;
#29781=CARTESIAN_POINT ( 'NONE',  ( -27.16883889988623935, 49.57500000273120122, 19.73931689729374739 ) ) ;
#29788=CARTESIAN_POINT ( 'NONE',  ( -2.092463501923844636E-15, 65.49999999999998579, -34.17252228774368916 ) ) ;
#29789=CARTESIAN_POINT ( 'NONE',  ( -33.58253175000000113, 7.025000002731188964, -10.91162601494193218 ) ) ;
#29801=CARTESIAN_POINT ( 'NONE',  ( 6.486482029760649416E-15, 57.62500000273119127, 35.31076352940723240 ) ) ;
#29802=CARTESIAN_POINT ( 'NONE',  ( 33.58253175000000113, 28.37500000273117351, -4.112674001490185761E-15 ) ) ;
#29828=ADVANCED_FACE ( 'NONE', ( #28592 ), #26029, .F. ) ;
#29833=UNCERTAINTY_MEASURE_WITH_UNIT (LENGTH_MEASURE( 1.000000000000000082E-05 ), #30188, 'distance_accuracy_value', 'NONE');
#29834=CARTESIAN_POINT ( 'NONE',  ( -10.37757302488623701, 29.52500000273118630, 31.93888565452638417 ) ) ;
#29835=CARTESIAN_POINT ( 'NONE',  ( -5.147494310547423346, 56.94874572391555034, 32.50000000000000000 ) ) ;
#29838=CARTESIAN_POINT ( 'NONE',  ( -32.50000000000000000, 46.60000000546237686, 10.55989012756946366 ) ) ;
#29843=CARTESIAN_POINT ( 'NONE',  ( -27.16883889988623935, 77.32500000273120122, 19.73931689729374739 ) ) ;
#29846=( GEOMETRIC_REPRESENTATION_CONTEXT ( 3 ) GLOBAL_UNCERTAINTY_ASSIGNED_CONTEXT ( ( #3761 ) ) GLOBAL_UNIT_ASSIGNED_CONTEXT ( ( #29170, #26101, #2598 ) ) REPRESENTATION_CONTEXT ( 'NONE', 'WORKASPACE' ) );
#29850=CARTESIAN_POINT ( 'NONE',  ( -32.50000000000000000, 12.60000000546238219, 10.55989012756946366 ) ) ;
#29856=CARTESIAN_POINT ( 'NONE',  ( -20.08610463437156923, 62.80000000546237260, 27.64615127144130113 ) ) ;
#29859=CARTESIAN_POINT ( 'NONE',  ( 10.04305231718579705, 38.60000000000000853, 30.90933677959248982 ) ) ;
#29867=CARTESIAN_POINT ( 'NONE',  ( 10.37757302488624767, 67.97500000273119269, 31.93888565452638417 ) ) ;
#29873=CARTESIAN_POINT ( 'NONE',  ( 20.75514604977248467, 46.42500000273119554, -28.56700777964554305 ) ) ;
#29874=CARTESIAN_POINT ( 'NONE',  ( -10.37757302488623701, 9.775000002731168536, 31.93888565452638417 ) ) ;
#29875=CARTESIAN_POINT ( 'NONE',  ( 33.58253175000000823, 64.27500000273118985, 10.91162601494192685 ) ) ;
#29879=CARTESIAN_POINT ( 'NONE',  ( -26.29305231718578995, 66.70000000546237118, 19.10302069950538595 ) ) ;
#29885=CARTESIAN_POINT ( 'NONE',  ( -20.75514604977248823, 41.07500000273119412, -28.56700777964554305 ) ) ;
#29887=CARTESIAN_POINT ( 'NONE',  ( 10.04305231718579705, 27.10000000546238041, 30.90933677959248982 ) ) ;
#29905=CARTESIAN_POINT ( 'NONE',  ( -1.778240108872766143E-15, 63.50000000000000000, -32.49999999999999289 ) ) ;
#29907=CARTESIAN_POINT ( 'NONE',  ( -2.092463501923844636E-15, 11.50000000000000000, -34.17252228774368916 ) ) ;
#29914=CARTESIAN_POINT ( 'NONE',  ( -10.37757302488624411, 64.72500000273119269, -31.93888565452638417 ) ) ;
#29915=CARTESIAN_POINT ( 'NONE',  ( -20.75514604977248823, 33.07500000273117990, -28.56700777964554305 ) ) ;
#29916=CARTESIAN_POINT ( 'NONE',  ( -10.37757302488623701, 17.77500000273117564, 31.93888565452638417 ) ) ;
#29922=CARTESIAN_POINT ( 'NONE',  ( -32.50000000000000000, 47.89999999999999858, -10.55989012756945478 ) ) ;
#29927=CARTESIAN_POINT ( 'NONE',  ( -27.16883889988623935, 63.57500000273117990, 19.73931689729374739 ) ) ;
#29932=CARTESIAN_POINT ( 'NONE',  ( -33.58253175000000113, 37.02500000273117564, -10.91162601494193218 ) ) ;
#29937=CARTESIAN_POINT ( 'NONE',  ( 32.50000000000000000, 58.99999999999998579, -3.980102097228898626E-15 ) ) ;
#29947=CARTESIAN_POINT ( 'NONE',  ( 10.04305231718578817, 53.90000000546239534, -30.90933677959249337 ) ) ;
#29953=CARTESIAN_POINT ( 'NONE',  ( -10.37757302488623701, 49.77500000273120406, 31.93888565452638417 ) ) ;
#29959=CARTESIAN_POINT ( 'NONE',  ( 32.50000000000000000, 66.99999999999998579, -3.980102097228898626E-15 ) ) ;
#29964=CARTESIAN_POINT ( 'NONE',  ( -26.29305231718579350, 65.80000000000001137, -19.10302069950537884 ) ) ;
#29969=CARTESIAN_POINT ( 'NONE',  ( 10.37757302488624767, 55.72500000273118559, 31.93888565452638417 ) ) ;
#29970=CARTESIAN_POINT ( 'NONE',  ( 6.486482029760649416E-15, 25.87500000273117351, 35.31076352940723240 ) ) ;
#29985=CARTESIAN_POINT ( 'NONE',  ( 27.16883889988623935, 54.32500000273120122, -19.73931689729374384 ) ) ;
#29998=CARTESIAN_POINT ( 'NONE',  ( 31.78768264672016741, 66.99999999999997158, -7.374898305514718366 ) ) ;
#30000=CARTESIAN_POINT ( 'NONE',  ( -20.75514604977248823, 26.82500000273117280, -28.56700777964554305 ) ) ;
#30005=CARTESIAN_POINT ( 'NONE',  ( -32.50000000000000000, 50.40000000546237402, -10.55989012756945478 ) ) ;
#30007=CARTESIAN_POINT ( 'NONE',  ( -10.04305231718579172, 58.10000000546237686, -30.90933677959248982 ) ) ;
#30010=CARTESIAN_POINT ( 'NONE',  ( -33.58253175000000113, 75.12500000273118417, 0.000000000000000000 ) ) ;
#30014=CARTESIAN_POINT ( 'NONE',  ( 0.000000000000000000, 52.00000000000000711, 0.000000000000000000 ) ) ;
#30017=CARTESIAN_POINT ( 'NONE',  ( 32.50000000000000000, 11.50000000546237722, -3.980102097228898626E-15 ) ) ;
#30026=CARTESIAN_POINT ( 'NONE',  ( -26.29305231718579350, 35.79999999999998295, -19.10302069950537884 ) ) ;
#30034=VERTEX_POINT ( 'NONE', #29268 ) ;
#30038=CARTESIAN_POINT ( 'NONE',  ( 20.75514604977249178, 45.82500000273118701, 28.56700777964553950 ) ) ;
#30039=CARTESIAN_POINT ( 'NONE',  ( 27.16883889988624290, 2.175000002731186655, 19.73931689729373673 ) ) ;
#30040=CARTESIAN_POINT ( 'NONE',  ( -20.75514604977248823, 63.07500000273119412, -28.56700777964554305 ) ) ;
#30044=CARTESIAN_POINT ( 'NONE',  ( -20.08610463437156923, 64.80000000546237970, 27.64615127144130113 ) ) ;
#30050=CARTESIAN_POINT ( 'NONE',  ( 6.486482029760649416E-15, 39.87500000273119127, 35.31076352940723240 ) ) ;
#30052=CARTESIAN_POINT ( 'NONE',  ( 6.277390505771533514E-15, 29.00000000546237189, 34.17252228774368916 ) ) ;
#30060=CARTESIAN_POINT ( 'NONE',  ( 33.58253175000000113, 66.12500000273118417, -4.112674001490185761E-15 ) ) ;
#30069=CARTESIAN_POINT ( 'NONE',  ( -26.29305231718578995, 6.199999999999997513, 19.10302069950538595 ) ) ;
#30074=CARTESIAN_POINT ( 'NONE',  ( 27.16883889988624290, 63.92500000273120264, 19.73931689729373673 ) ) ;
#30075=CARTESIAN_POINT ( 'NONE',  ( 6.486482029760649416E-15, 27.87500000273120193, 35.31076352940723240 ) ) ;
#30076=CARTESIAN_POINT ( 'NONE',  ( 10.37757302488624767, 17.97500000273118204, 31.93888565452638417 ) ) ;
#30081=CARTESIAN_POINT ( 'NONE',  ( 20.08610463437158344, 48.70000000000000284, 27.64615127144129403 ) ) ;
#30082=CARTESIAN_POINT ( 'NONE',  ( 32.50000000000000000, 57.60000000546236976, -10.55989012756945833 ) ) ;
#30085=ORIENTED_EDGE ( 'NONE', *, *, #15671, .F. ) ;
#30086=CARTESIAN_POINT ( 'NONE',  ( -10.37757302488624411, 62.97500000273119269, -31.93888565452638417 ) ) ;
#30091=CARTESIAN_POINT ( 'NONE',  ( 27.16883889988624290, 27.92500000273119554, 19.73931689729373673 ) ) ;
#30107=EDGE_CURVE ( 'NONE', #1345, #19609, #13504, .T. ) ;
#30108=EDGE_CURVE ( 'NONE', #1221, #2261, #7577, .T. ) ;
#30115=CARTESIAN_POINT ( 'NONE',  ( -27.16883889988623935, 47.57500000273119412, 19.73931689729374739 ) ) ;
#30122=CARTESIAN_POINT ( 'NONE',  ( -32.50000000000000000, 69.99999999999998579, 0.000000000000000000 ) ) ;
#30127=CARTESIAN_POINT ( 'NONE',  ( -20.75514604977248112, 77.67500000273119554, 28.56700777964554661 ) ) ;
#30132=CARTESIAN_POINT ( 'NONE',  ( 33.58253175000000823, 52.02500000273118985, 10.91162601494192863 ) ) ;
#30133=CARTESIAN_POINT ( 'NONE',  ( 20.75514604977248467, 22.67500000273119198, -28.56700777964554305 ) ) ;
#30134=ORIENTED_EDGE ( 'NONE', *, *, #13556, .T. ) ;
#30144=CARTESIAN_POINT ( 'NONE',  ( -30.20345010595928059, 66.99999999999998579, -14.84467937978526564 ) ) ;
#30147=CARTESIAN_POINT ( 'NONE',  ( 33.58253175000000113, 54.22500000273117848, -10.91162601494193574 ) ) ;
#30161=CARTESIAN_POINT ( 'NONE',  ( 32.50000000000000000, 63.60000000546238397, -10.55989012756945833 ) ) ;
#30163=CARTESIAN_POINT ( 'NONE',  ( 20.75514604977248467, 20.42500000273120619, -28.56700777964554305 ) ) ;
#30165=CARTESIAN_POINT ( 'NONE',  ( 26.29305231718579350, 55.30000000546237970, 19.10302069950537529 ) ) ;
#30168=CARTESIAN_POINT ( 'NONE',  ( 10.04305231718579705, 45.10000000546236976, 30.90933677959248982 ) ) ;
#30174=CARTESIAN_POINT ( 'NONE',  ( -33.58253175000000113, 77.12500000273118417, 0.000000000000000000 ) ) ;
#30177=VERTEX_POINT ( 'NONE', #5500 ) ;
#30179=CARTESIAN_POINT ( 'NONE',  ( -32.50000000000000000, 10.60000000546237331, 10.55989012756946366 ) ) ;
#30188=( LENGTH_UNIT ( ) NAMED_UNIT ( * ) SI_UNIT ( .MILLI., .METRE. ) );
#30189=CARTESIAN_POINT ( 'NONE',  ( -10.04305231718579172, 37.60000000000000853, -30.90933677959248982 ) ) ;
#30202=( BOUNDED_CURVE ( )  B_SPLINE_CURVE ( 2, ( #22626, #19718, #12504, #9402, #15082, #14569, #30678, #4433, #30165, #25550, #14402, #17489, #6834 ),
 .UNSPECIFIED., .F., .T. ) 
 B_SPLINE_CURVE_WITH_KNOTS ( ( 3, 2, 2, 2, 2, 2, 3 ),
 ( 0.2884615384615384914, 0.2897435897435897689, 0.2923076923076923239, 0.2948717948717948789, 0.2974358974358974339, 0.2999999999999999889, 0.3012820512820512664 ),
 .UNSPECIFIED. ) 
 CURVE ( )  GEOMETRIC_REPRESENTATION_ITEM ( )  RATIONAL_B_SPLINE_CURVE ( ( 0.9755282581475768211, 0.9755282581475772652, 1.000000000000000000, 0.9510565162951535312, 1.000000000000000000, 0.9510565162951535312, 1.000000000000000000, 0.9510565162951535312, 1.000000000000000000, 0.9510565162951535312, 1.000000000000000000, 0.9755282581475768211, 0.9755282581475768211 ) ) 
 REPRESENTATION_ITEM ( '' )  );
#30204=CARTESIAN_POINT ( 'NONE',  ( -20.75514604977248823, 38.82500000273120122, -28.56700777964554305 ) ) ;
#30205=CARTESIAN_POINT ( 'NONE',  ( -20.75514604977248112, 5.675000002731189319, 28.56700777964554661 ) ) ;
#30206=CARTESIAN_POINT ( 'NONE',  ( 6.486482029760648627E-15, 57.87500000273117706, 35.31076352940722529 ) ) ;
#30211=CARTESIAN_POINT ( 'NONE',  ( -32.50000000000000000, 66.50000000546239676, 0.000000000000000000 ) ) ;
#30217=CARTESIAN_POINT ( 'NONE',  ( 27.16883889988623935, 42.57500000273119412, -19.73931689729374384 ) ) ;
#30220=CARTESIAN_POINT ( 'NONE',  ( -32.50000000000000000, 28.50000000546236478, 0.000000000000000000 ) ) ;
#30223=ORIENTED_EDGE ( 'NONE', *, *, #10518, .F. ) ;
#30230=CARTESIAN_POINT ( 'NONE',  ( 2.205017735002230837E-13, 56.00000000546238255, -32.50000000000000000 ) ) ;
#30235=CARTESIAN_POINT ( 'NONE',  ( 14.93337011119343671, 52.00000000000000711, 30.15969763299871786 ) ) ;
#30236=CARTESIAN_POINT ( 'NONE',  ( 20.75514604977248467, 78.67500000273116711, -28.56700777964554305 ) ) ;
#30241=CARTESIAN_POINT ( 'NONE',  ( 27.16883889988623935, 66.32500000273118701, -19.73931689729374384 ) ) ;
#30242=CARTESIAN_POINT ( 'NONE',  ( -27.16883889988624290, 23.17500000273119198, -19.73931689729374028 ) ) ;
#30243=CARTESIAN_POINT ( 'NONE',  ( -27.16883889988623935, 7.575000002731188786, 19.73931689729374739 ) ) ;
#30250=CARTESIAN_POINT ( 'NONE',  ( 26.29305231718578995, 47.20000000000000284, -19.10302069950538240 ) ) ;
#30251=CARTESIAN_POINT ( 'NONE',  ( 20.08610463437158344, 57.20000000546237828, 27.64615127144129403 ) ) ;
#30255=CARTESIAN_POINT ( 'NONE',  ( 33.58253175000000823, 62.27500000273118275, 10.91162601494192863 ) ) ;
#30262=CARTESIAN_POINT ( 'NONE',  ( 10.37757302488624767, 33.72500000273119269, 31.93888565452638417 ) ) ;
#30286=CARTESIAN_POINT ( 'NONE',  ( -10.37757302488624411, 40.97500000273117138, -31.93888565452638417 ) ) ;
#30291=CARTESIAN_POINT ( 'NONE',  ( 20.08610463437158344, 66.69999999999997442, 27.64615127144129403 ) ) ;
#30302=CARTESIAN_POINT ( 'NONE',  ( -20.75514604977248112, 49.42500000273118133, 28.56700777964554661 ) ) ;
#30304=CARTESIAN_POINT ( 'NONE',  ( -20.75514604977248823, 21.07500000273118346, -28.56700777964554305 ) ) ;
#30320=CARTESIAN_POINT ( 'NONE',  ( 10.37757302488624767, 57.72500000273118559, 31.93888565452638417 ) ) ;
#30335=CARTESIAN_POINT ( 'NONE',  ( 10.37757302488624056, 24.52500000273118275, -31.93888565452638417 ) ) ;
#30341=CARTESIAN_POINT ( 'NONE',  ( -26.29305231718578995, 40.70000000546237828, 19.10302069950538595 ) ) ;
#30345=CARTESIAN_POINT ( 'NONE',  ( -2.162160676586881955E-15, 66.62500000273118417, -35.31076352940723240 ) ) ;
#30351=CARTESIAN_POINT ( 'NONE',  ( 20.75514604977248467, 8.425000002731186655, -28.56700777964554305 ) ) ;
#30361=CARTESIAN_POINT ( 'NONE',  ( -2.092463501923844636E-15, 37.50000000000000711, -34.17252228774368916 ) ) ;
#30365=CARTESIAN_POINT ( 'NONE',  ( 26.29305231718578995, 63.20000000000001705, -19.10302069950538240 ) ) ;
#30373=CARTESIAN_POINT ( 'NONE',  ( -27.16883889988624290, 42.92500000273118133, -19.73931689729374028 ) ) ;
#30374=CARTESIAN_POINT ( 'NONE',  ( 27.16883889988623935, 2.575000002731184345, -19.73931689729374384 ) ) ;
#30375=CARTESIAN_POINT ( 'NONE',  ( -27.16883889988624290, 53.17500000273118843, -19.73931689729374028 ) ) ;
#30378=CARTESIAN_POINT ( 'NONE',  ( 32.50000000000000711, 61.40000000546237402, 10.55989012756945122 ) ) ;
#30385=CARTESIAN_POINT ( 'NONE',  ( -10.37757302488623701, 41.77500000273119696, 31.93888565452638417 ) ) ;
#30388=CARTESIAN_POINT ( 'NONE',  ( 20.08610463437157279, 29.80000000546237970, -27.64615127144129758 ) ) ;
#30400=CARTESIAN_POINT ( 'NONE',  ( 10.37757302488624056, 66.52500000273118985, -31.93888565452638417 ) ) ;
#30411=CARTESIAN_POINT ( 'NONE',  ( 33.58253175000000113, 78.47500000273116427, -10.91162601494193751 ) ) ;
#30416=CARTESIAN_POINT ( 'NONE',  ( -33.58253175000000113, 61.02500000273118985, -10.91162601494193218 ) ) ;
#30417=CARTESIAN_POINT ( 'NONE',  ( 20.75514604977248467, 26.67500000273118133, -28.56700777964554305 ) ) ;
#30418=CARTESIAN_POINT ( 'NONE',  ( 27.16883889988624290, 8.175000002731177773, 19.73931689729373673 ) ) ;
#30422=CARTESIAN_POINT ( 'NONE',  ( -27.16883889988623935, 1.325000002731183013, 19.73931689729374739 ) ) ;
#30424=CARTESIAN_POINT ( 'NONE',  ( 10.04305231718578817, 41.40000000000000568, -30.90933677959249337 ) ) ;
#30430=CARTESIAN_POINT ( 'NONE',  ( 10.37757302488624767, 59.97500000273119269, 31.93888565452638417 ) ) ;
#30435=CARTESIAN_POINT ( 'NONE',  ( -10.37757302488623701, 31.52500000273118630, 31.93888565452638417 ) ) ;
#30458=CARTESIAN_POINT ( 'NONE',  ( 33.58253175000000113, 44.37500000273119127, -4.112674001490185761E-15 ) ) ;
#30463=CARTESIAN_POINT ( 'NONE',  ( 26.29305231718579350, 66.80000000000001137, 19.10302069950537529 ) ) ;
#30468=CARTESIAN_POINT ( 'NONE',  ( 33.58253175000000823, 78.27500000273116143, 10.91162601494192863 ) ) ;
#30473=CARTESIAN_POINT ( 'NONE',  ( -10.37757302488624411, 46.72500000273120691, -31.93888565452638417 ) ) ;
#30474=CARTESIAN_POINT ( 'NONE',  ( 6.486482029760649416E-15, 23.87500000273117706, 35.31076352940723240 ) ) ;
#30496=CARTESIAN_POINT ( 'NONE',  ( -33.58253175000000113, 63.27500000273118985, -10.91162601494193218 ) ) ;
#30503=CARTESIAN_POINT ( 'NONE',  ( 32.50000000000000711, 63.40000000546236691, 10.55989012756945122 ) ) ;
#30505=CARTESIAN_POINT ( 'NONE',  ( 27.16883889988623935, 24.32500000273117635, -19.73931689729374384 ) ) ;
#30507=CARTESIAN_POINT ( 'NONE',  ( 5.147494310547426899, 53.44874571845314648, -32.50000000000000000 ) ) ;
#30510=CARTESIAN_POINT ( 'NONE',  ( 32.50000000000000000, 43.50000000546237544, -3.980102097228898626E-15 ) ) ;
#30515=ORIENTED_EDGE ( 'NONE', *, *, #13660, .F. ) ;
#30516=CARTESIAN_POINT ( 'NONE',  ( -33.58253175000000113, 69.02500000273118985, -10.91162601494193218 ) ) ;
#30522=CARTESIAN_POINT ( 'NONE',  ( -20.75514604977248112, 11.42500000273117955, 28.56700777964554661 ) ) ;
#30528=EDGE_CURVE ( 'NONE', #29627, #1345, #18113, .T. ) ;
#30534=CARTESIAN_POINT ( 'NONE',  ( -26.29305231718579350, 37.79999999999998295, -19.10302069950537884 ) ) ;
#30548=CARTESIAN_POINT ( 'NONE',  ( -2.162160676586881955E-15, 40.62500000273120548, -35.31076352940723240 ) ) ;
#30549=CARTESIAN_POINT ( 'NONE',  ( 27.16883889988624290, 4.175000002731188431, 19.73931689729373673 ) ) ;
#30550=CARTESIAN_POINT ( 'NONE',  ( -20.75514604977248823, 55.07500000273117990, -28.56700777964554305 ) ) ;
#30554=CARTESIAN_POINT ( 'NONE',  ( -32.50000000000000000, 60.50000000546238965, 0.000000000000000000 ) ) ;
#30560=CARTESIAN_POINT ( 'NONE',  ( 33.58253175000000823, 40.27500000273118985, 10.91162601494192863 ) ) ;
#30564=CARTESIAN_POINT ( 'NONE',  ( -32.50000000000000000, 26.60000000546239107, 10.55989012756946366 ) ) ;
#30582=CARTESIAN_POINT ( 'NONE',  ( -32.50000000000000000, 56.10000000000000142, 10.55989012756946366 ) ) ;
#30583=DIRECTION ( 'NONE',  ( -0.5000000000000001110, 0.000000000000000000, 0.8660254037844387076 ) ) ;
#30584=CARTESIAN_POINT ( 'NONE',  ( -26.29305231718578995, 4.199999999999995737, 19.10302069950538595 ) ) ;
#30589=CARTESIAN_POINT ( 'NONE',  ( 27.16883889988623935, 62.32500000273120833, -19.73931689729374384 ) ) ;
#30590=CARTESIAN_POINT ( 'NONE',  ( 33.58253175000000823, 22.27500000273116854, 10.91162601494192863 ) ) ;
#30591=CARTESIAN_POINT ( 'NONE',  ( 20.75514604977248467, 10.67500000273119021, -28.56700777964554305 ) ) ;
#30595=CARTESIAN_POINT ( 'NONE',  ( 20.08610463437158344, 77.20000000546238539, 27.64615127144129403 ) ) ;
#30598=CARTESIAN_POINT ( 'NONE',  ( -10.04305231718579172, 43.60000000000001563, -30.90933677959248982 ) ) ;
#30603=CARTESIAN_POINT ( 'NONE',  ( 33.58253175000000113, 60.37500000273120548, -4.112674001490185761E-15 ) ) ;
#30608=CARTESIAN_POINT ( 'NONE',  ( -27.16883889988623935, 31.32500000273118346, 19.73931689729374739 ) ) ;
#30628=CARTESIAN_POINT ( 'NONE',  ( 20.75514604977249178, 44.07500000273117990, 28.56700777964553950 ) ) ;
#30634=CARTESIAN_POINT ( 'NONE',  ( 10.04305231718578817, 57.39999999999999147, -30.90933677959249337 ) ) ;
#30644=CARTESIAN_POINT ( 'NONE',  ( 20.75514604977249178, 47.82500000273117990, 28.56700777964553950 ) ) ;
#30645=CARTESIAN_POINT ( 'NONE',  ( -2.162160676586881955E-15, 22.87500000273118062, -35.31076352940723240 ) ) ;
#30649=FACE_OUTER_BOUND ( 'NONE', #6519, .T. ) ;
#30668=CARTESIAN_POINT ( 'NONE',  ( 33.58253175000000113, 64.47500000273120691, -10.91162601494193751 ) ) ;
#30676=CARTESIAN_POINT ( 'NONE',  ( 33.58253175000000823, 24.02500000273117564, 10.91162601494192863 ) ) ;
#30678=CARTESIAN_POINT ( 'NONE',  ( 32.50000000000000000, 55.50000000546238965, -3.980102097228898626E-15 ) ) ;
#30681=CARTESIAN_POINT ( 'NONE',  ( -32.50000000000000000, 42.40000000546238823, -10.55989012756945478 ) ) ;
#30688=CARTESIAN_POINT ( 'NONE',  ( 20.75514604977248467, 70.42500000273119554, -28.56700777964554305 ) ) ;
#30694=CARTESIAN_POINT ( 'NONE',  ( 33.58253175000000113, 14.12500000273118950, -4.112674001490185761E-15 ) ) ;
#30706=CARTESIAN_POINT ( 'NONE',  ( 20.08610463437158344, 26.70000000000000284, 27.64615127144129403 ) ) ;
#30720=CARTESIAN_POINT ( 'NONE',  ( -27.16883889988624290, 40.92500000273118133, -19.73931689729374028 ) ) ;
#30721=CARTESIAN_POINT ( 'NONE',  ( 27.16883889988624290, 6.175000002731190207, 19.73931689729373673 ) ) ;
#30722=CARTESIAN_POINT ( 'NONE',  ( 20.75514604977248467, 58.67500000273118843, -28.56700777964554305 ) ) ;
#30726=CARTESIAN_POINT ( 'NONE',  ( -26.29305231718579350, 60.30000000546238681, -19.10302069950537884 ) ) ;
#30733=CARTESIAN_POINT ( 'NONE',  ( -27.16883889988624290, 35.17500000273120264, -19.73931689729374028 ) ) ;
#30737=CARTESIAN_POINT ( 'NONE',  ( -32.50000000000000000, 20.40000000546238113, -10.55989012756945478 ) ) ;
#30747=EDGE_CURVE ( 'NONE', #30034, #24911, #29117, .T. ) ;
#30758=CARTESIAN_POINT ( 'NONE',  ( 32.50000000000000000, 5.000000000000004441, -3.980102097228898626E-15 ) ) ;
#30763=CARTESIAN_POINT ( 'NONE',  ( 6.486482029760649416E-15, 59.62500000273118417, 35.31076352940723240 ) ) ;
#30764=CARTESIAN_POINT ( 'NONE',  ( 10.37757302488624767, 23.97500000273118559, 31.93888565452638417 ) ) ;
#30765=CARTESIAN_POINT ( 'NONE',  ( 6.486482029760649416E-15, 9.875000002731187720, 35.31076352940723240 ) ) ;
#30770=CARTESIAN_POINT ( 'NONE',  ( 10.04305231718578817, 77.90000000546235981, -30.90933677959249337 ) ) ;
#30772=CARTESIAN_POINT ( 'NONE',  ( -10.04305231718579172, 39.60000000000000853, -30.90933677959248982 ) ) ;
#30778=CARTESIAN_POINT ( 'NONE',  ( 33.58253175000000113, 54.47500000273117138, -10.91162601494193751 ) ) ;
#30782=ORIENTED_EDGE ( 'NONE', *, *, #23495, .F. ) ;
#30783=CARTESIAN_POINT ( 'NONE',  ( -33.58253175000000113, 29.12500000273120193, 0.000000000000000000 ) ) ;
#30803=CARTESIAN_POINT ( 'NONE',  ( -33.58253175000000113, 45.27500000273116854, -10.91162601494193218 ) ) ;
#30807=CARTESIAN_POINT ( 'NONE',  ( -32.50000000000000000, 61.89999999999999147, -10.55989012756945478 ) ) ;
#30814=CARTESIAN_POINT ( 'NONE',  ( -27.16883889988623935, 77.57500000273120122, 19.73931689729374739 ) ) ;
#30819=ORIENTED_EDGE ( 'NONE', *, *, #33551, .F. ) ;
#30820=CARTESIAN_POINT ( 'NONE',  ( -10.37757302488624411, 52.72500000273121401, -31.93888565452638417 ) ) ;
#30825=CARTESIAN_POINT ( 'NONE',  ( -20.08610463437157989, 8.200000005462374730, -27.64615127144129758 ) ) ;
#30847=CARTESIAN_POINT ( 'NONE',  ( 27.16883889988623935, 62.57500000273117990, -19.73931689729374384 ) ) ;
#30853=CARTESIAN_POINT ( 'NONE',  ( -26.29305231718579350, 79.79999999999999716, -19.10302069950537884 ) ) ;
#30854=CARTESIAN_POINT ( 'NONE',  ( 10.37757302488624767, 23.72500000273118559, 31.93888565452638417 ) ) ;
#30858=CARTESIAN_POINT ( 'NONE',  ( -32.50000000000000000, 44.60000000546237686, 10.55989012756946366 ) ) ;
#30864=CARTESIAN_POINT ( 'NONE',  ( -27.16883889988624290, 66.92500000273119554, -19.73931689729374028 ) ) ;
#30870=CARTESIAN_POINT ( 'NONE',  ( 6.486482029760649416E-15, 13.62500000273118417, 35.31076352940723240 ) ) ;
#30880=CARTESIAN_POINT ( 'NONE',  ( 10.04305231718578817, 31.39999999999999858, -30.90933677959249337 ) ) ;
#30881=EDGE_CURVE ( 'NONE', #22505, #52, #30202, .T. ) ;
#30889=AXIS2_PLACEMENT_3D ( 'NONE', #9883, #8321, #11080 ) ;
#30895=CARTESIAN_POINT ( 'NONE',  ( 27.16883889988624290, 43.92500000273118133, 19.73931689729373673 ) ) ;
#30896=DIRECTION ( 'NONE',  ( 0.000000000000000000, 1.000000000000000000, 0.000000000000000000 ) ) ;
#30897=CARTESIAN_POINT ( 'NONE',  ( -33.58253175000000113, 55.37500000273119838, 0.000000000000000000 ) ) ;
#30902=CARTESIAN_POINT ( 'NONE',  ( -32.50000000000000000, 60.60000000546239107, 10.55989012756946366 ) ) ;
#30904=CARTESIAN_POINT ( 'NONE',  ( 5.147494310547426899, 57.94874572391552903, -32.50000000000000000 ) ) ;
#30909=CARTESIAN_POINT ( 'NONE',  ( -10.37757302488623701, 33.77500000273118985, 31.93888565452638417 ) ) ;
#30913=CARTESIAN_POINT ( 'NONE',  ( 32.50000000000000000, 21.50000000546238610, -3.980102097228898626E-15 ) ) ;
#30919=CYLINDRICAL_SURFACE ( 'NONE', #25924, 32.50000000000000000 ) ;
#30924=CARTESIAN_POINT ( 'NONE',  ( -10.37757302488624411, 58.72500000273119269, -31.93888565452638417 ) ) ;
#30934=CARTESIAN_POINT ( 'NONE',  ( -2.162160676586881955E-15, 72.87500000273115575, -35.31076352940723240 ) ) ;
#30939=CARTESIAN_POINT ( 'NONE',  ( 20.75514604977249178, 57.82500000273118701, 28.56700777964553950 ) ) ;
#30940=CARTESIAN_POINT ( 'NONE',  ( 27.16883889988623935, 20.57500000273120122, -19.73931689729374384 ) ) ;
#30941=CARTESIAN_POINT ( 'NONE',  ( -20.75514604977248112, 11.67500000273118843, 28.56700777964554661 ) ) ;
#30945=CARTESIAN_POINT ( 'NONE',  ( 33.58253175000000823, 2.025000002731187632, 10.91162601494192863 ) ) ;
#30947=CARTESIAN_POINT ( 'NONE',  ( -2.092463501923844636E-15, 41.49999999999999289, -34.17252228774368916 ) ) ;
#30952=CARTESIAN_POINT ( 'NONE',  ( 20.75514604977248467, 56.67500000273119554, -28.56700777964554305 ) ) ;
#30957=CARTESIAN_POINT ( 'NONE',  ( 10.37757302488624767, 23.72500000273118559, 31.93888565452638417 ) ) ;
#30972=CARTESIAN_POINT ( 'NONE',  ( 32.50000000000000000, 17.10000000000001208, -10.55989012756945833 ) ) ;
#30978=CARTESIAN_POINT ( 'NONE',  ( -33.58253175000000113, 77.02500000273118985, -10.91162601494193218 ) ) ;
#30979=CARTESIAN_POINT ( 'NONE',  ( -33.58253175000000113, 41.37500000273118417, 0.000000000000000000 ) ) ;
#30985=CARTESIAN_POINT ( 'NONE',  ( 20.08610463437158344, 62.69999999999999574, 27.64615127144129403 ) ) ;
#30989=CARTESIAN_POINT ( 'NONE',  ( -27.16883889988624290, 75.17500000273118133, -19.73931689729374028 ) ) ;
#30995=ORIENTED_EDGE ( 'NONE', *, *, #18697, .F. ) ;
#30996=CARTESIAN_POINT ( 'NONE',  ( -10.37757302488623701, 45.52500000273117564, 31.93888565452638417 ) ) ;
#31000=CARTESIAN_POINT ( 'NONE',  ( -32.50000000000000000, 2.500000005462382546, 0.000000000000000000 ) ) ;
#31019=CARTESIAN_POINT ( 'NONE',  ( -33.58253175000000113, 61.37500000273120548, 0.000000000000000000 ) ) ;
#31026=CARTESIAN_POINT ( 'NONE',  ( 26.29305231718579350, 76.80000000000002558, 19.10302069950537529 ) ) ;
#31027=CARTESIAN_POINT ( 'NONE',  ( -20.75514604977248112, 13.42500000273119198, 28.56700777964554661 ) ) ;
#31032=CARTESIAN_POINT ( 'NONE',  ( 10.04305231718578817, 33.90000000546238113, -30.90933677959249337 ) ) ;
#31033=EDGE_CURVE ( 'NONE', #17050, #25078, #27951, .T. ) ;
#31034=CARTESIAN_POINT ( 'NONE',  ( -5.147494310547423346, 66.44874571845315359, 32.50000000000000000 ) ) ;
#31039=CARTESIAN_POINT ( 'NONE',  ( 10.37757302488624056, 68.52500000273118985, -31.93888565452638417 ) ) ;
#31042=ORIENTED_EDGE ( 'NONE', *, *, #26141, .T. ) ;
#31046=CARTESIAN_POINT ( 'NONE',  ( -10.37757302488624411, 12.72500000273117671, -31.93888565452638417 ) ) ;
#31057=CARTESIAN_POINT ( 'NONE',  ( -26.29305231718578995, 32.19999999999999574, 19.10302069950538595 ) ) ;
#31066=CARTESIAN_POINT ( 'NONE',  ( -7.738208025866914141, 66.99999999999998579, -32.61747650539069099 ) ) ;
#31067=CARTESIAN_POINT ( 'NONE',  ( -33.58253175000000113, 37.02500000273117564, -10.91162601494193218 ) ) ;
#31068=CARTESIAN_POINT ( 'NONE',  ( 20.08610463437157279, 57.29999999999999005, -27.64615127144129758 ) ) ;
#31073=CARTESIAN_POINT ( 'NONE',  ( -26.29305231718578995, 58.70000000546237118, 19.10302069950538595 ) ) ;
#31081=CARTESIAN_POINT ( 'NONE',  ( 27.16883889988623935, 32.57500000273117990, -19.73931689729374384 ) ) ;
#31085=CARTESIAN_POINT ( 'NONE',  ( 26.29305231718578995, 21.70000000546239249, -19.10302069950538240 ) ) ;
#31095=CARTESIAN_POINT ( 'NONE',  ( 33.58253175000000823, 64.02500000273118985, 10.91162601494192685 ) ) ;
#31106=CARTESIAN_POINT ( 'NONE',  ( 33.58253175000000113, 74.47500000273116427, -10.91162601494193751 ) ) ;
#31111=CARTESIAN_POINT ( 'NONE',  ( -10.37757302488623701, 61.52500000273118985, 31.93888565452638417 ) ) ;
#31112=CARTESIAN_POINT ( 'NONE',  ( -27.16883889988624290, 15.17500000273118488, -19.73931689729374028 ) ) ;
#31113=CARTESIAN_POINT ( 'NONE',  ( -10.37757302488623701, 1.775000002731188964, 31.93888565452638417 ) ) ;
#31118=CARTESIAN_POINT ( 'NONE',  ( 27.16883889988624290, 1.925000002731186433, 19.73931689729373673 ) ) ;
#31120=CARTESIAN_POINT ( 'NONE',  ( 20.08610463437158344, 40.69999999999999574, 27.64615127144129403 ) ) ;
#31125=CARTESIAN_POINT ( 'NONE',  ( 20.75514604977249178, 56.07500000273117990, 28.56700777964553950 ) ) ;
#31126=( BOUNDED_CURVE ( )  B_SPLINE_CURVE ( 2, ( #13684, #24802, #29947, #24314, #788, #29608, #22240, #27047, #3540, #19004, #5951, #16925, #3872 ),
 .UNSPECIFIED., .F., .T. ) 
 B_SPLINE_CURVE_WITH_KNOTS ( ( 3, 2, 2, 2, 2, 2, 3 ),
 ( 0.3141025641025640969, 0.3153846153846153744, 0.3179487179487179294, 0.3205128205128205399, 0.3230769230769230949, 0.3256410256410256499, 0.3269230769230769273 ),
 .UNSPECIFIED. ) 
 CURVE ( )  GEOMETRIC_REPRESENTATION_ITEM ( )  RATIONAL_B_SPLINE_CURVE ( ( 0.9755282581475768211, 0.9755282581475768211, 1.000000000000000000, 0.9510565162951535312, 1.000000000000000000, 0.9510565162951535312, 1.000000000000000000, 0.9510565162951535312, 1.000000000000000000, 0.9510565162951535312, 1.000000000000000000, 0.9755282581475768211, 0.9755282581475768211 ) ) 
 REPRESENTATION_ITEM ( '' )  );
#31131=CARTESIAN_POINT ( 'NONE',  ( 33.58253175000000113, 26.22500000273119625, -10.91162601494193751 ) ) ;
#31146=CARTESIAN_POINT ( 'NONE',  ( -2.092463501923844636E-15, 19.49999999999998934, -34.17252228774368916 ) ) ;
#31153=CARTESIAN_POINT ( 'NONE',  ( -33.58253175000000113, 37.27500000273119696, -10.91162601494193218 ) ) ;
#31158=CARTESIAN_POINT ( 'NONE',  ( -32.50000000000000000, 58.10000000000000142, 10.55989012756946366 ) ) ;
#31162=CARTESIAN_POINT ( 'NONE',  ( 10.37757302488624767, 73.97500000273120691, 31.93888565452638417 ) ) ;
#31168=CARTESIAN_POINT ( 'NONE',  ( -27.16883889988624290, 44.92500000273118133, -19.73931689729374028 ) ) ;
#31171=CARTESIAN_POINT ( 'NONE',  ( 20.08610463437158344, 1.200000005462378283, 27.64615127144129403 ) ) ;
#31181=CYLINDRICAL_SURFACE ( 'NONE', #17064, 32.50000000000000000 ) ;
#31185=PRODUCT_CONTEXT ( 'NONE', #27191, 'mechanical' ) ;
#31193=CARTESIAN_POINT ( 'NONE',  ( -27.16883889988624290, 55.17500000273119554, -19.73931689729374028 ) ) ;
#31199=CARTESIAN_POINT ( 'NONE',  ( -10.04305231718579172, 77.59999999999999432, -30.90933677959248982 ) ) ;
#31200=CARTESIAN_POINT ( 'NONE',  ( 33.58253175000000113, 14.12500000273118950, -4.112674001490185761E-15 ) ) ;
#31201=CARTESIAN_POINT ( 'NONE',  ( 3.980102097228898626E-15, 52.00000000000000711, -32.50000000000000000 ) ) ;
#31205=CARTESIAN_POINT ( 'NONE',  ( -10.04305231718578462, 36.90000000546238113, 30.90933677959249337 ) ) ;
#31210=CARTESIAN_POINT ( 'NONE',  ( 27.16883889988624290, 61.92500000273119554, 19.73931689729373673 ) ) ;
#31215=CARTESIAN_POINT ( 'NONE',  ( 33.58253175000000823, 6.025000002731191628, 10.91162601494192863 ) ) ;
#31222=LINE ( 'NONE', #7715, #22512 ) ;
#31225=CARTESIAN_POINT ( 'NONE',  ( -20.08610463437157989, 29.69999999999999574, -27.64615127144129758 ) ) ;
#31230=CARTESIAN_POINT ( 'NONE',  ( -33.35123603814785298, 67.00000000000000000, -2.296425957314693012 ) ) ;
#31237=CARTESIAN_POINT ( 'NONE',  ( 20.75514604977248467, 34.42500000273117422, -28.56700777964554305 ) ) ;
#31242=CARTESIAN_POINT ( 'NONE',  ( -2.092463501923844636E-15, 52.00000000546236834, -34.17252228774368916 ) ) ;
#31249=CARTESIAN_POINT ( 'NONE',  ( -33.58253175000000113, 37.27500000273119696, -10.91162601494193218 ) ) ;
#31253=CARTESIAN_POINT ( 'NONE',  ( 32.50000000000000000, 23.60000000546236976, -10.55989012756945833 ) ) ;
#31263=CARTESIAN_POINT ( 'NONE',  ( 6.486482029760648627E-15, 63.62500000273117706, 35.31076352940722529 ) ) ;
#31275=CARTESIAN_POINT ( 'NONE',  ( 33.58253175000000113, 74.37500000273118417, -4.112674001490185761E-15 ) ) ;
#31279=CARTESIAN_POINT ( 'NONE',  ( -20.75514604977248112, 53.42500000273117422, 28.56700777964554661 ) ) ;
#31280=CARTESIAN_POINT ( 'NONE',  ( -10.37757302488623701, 17.77500000273117564, 31.93888565452638417 ) ) ;
#31281=CARTESIAN_POINT ( 'NONE',  ( 33.58253175000000823, 2.275000002731194293, 10.91162601494192863 ) ) ;
#31285=CARTESIAN_POINT ( 'NONE',  ( 6.277390505771533514E-15, 75.00000000546238255, 34.17252228774368916 ) ) ;
#31286=CARTESIAN_POINT ( 'NONE',  ( 33.35123603814782456, 52.00000000000003553, 2.296425957315384458 ) ) ;
#31291=CARTESIAN_POINT ( 'NONE',  ( -10.37757302488624411, 56.97500000273118559, -31.93888565452638417 ) ) ;
#31297=CARTESIAN_POINT ( 'NONE',  ( 33.58253175000000113, 22.12500000273119483, -4.112674001490185761E-15 ) ) ;
#31310=CARTESIAN_POINT ( 'NONE',  ( -1.778240108872766143E-15, 59.50000000000000711, -32.49999999999999289 ) ) ;
#31311=CARTESIAN_POINT ( 'NONE',  ( 20.08610463437157279, 15.29999999999998472, -27.64615127144129758 ) ) ;
#31319=CARTESIAN_POINT ( 'NONE',  ( 27.16883889988624290, 75.92500000273120975, 19.73931689729373673 ) ) ;
#31320=VECTOR ( 'NONE', #19199, 1000.000000000000000 ) ;
#31321=CARTESIAN_POINT ( 'NONE',  ( -2.162160676586881955E-15, 36.87500000273116996, -35.31076352940723240 ) ) ;
#31328=CARTESIAN_POINT ( 'NONE',  ( -32.50000000000000000, 57.99999999999997868, 0.000000000000000000 ) ) ;
#31332=CARTESIAN_POINT ( 'NONE',  ( -27.16883889988623935, 73.57500000273118701, 19.73931689729374739 ) ) ;
#31337=CARTESIAN_POINT ( 'NONE',  ( 33.58253175000000113, 44.22500000273117138, -10.91162601494193751 ) ) ;
#31341=CARTESIAN_POINT ( 'NONE',  ( 10.04305231718578817, 3.900000005462381125, -30.90933677959249337 ) ) ;
#31360=CARTESIAN_POINT ( 'NONE',  ( -10.37757302488624411, 56.97500000273118559, -31.93888565452638417 ) ) ;
#31365=CARTESIAN_POINT ( 'NONE',  ( -40.00000000000000711, 66.99999999999998579, 23.09401076758504345 ) ) ;
#31366=CARTESIAN_POINT ( 'NONE',  ( -20.08610463437156923, 78.29999999999999716, 27.64615127144130113 ) ) ;
#31367=CARTESIAN_POINT ( 'NONE',  ( -20.75514604977248823, 16.82500000273120122, -28.56700777964554305 ) ) ;
#31372=CARTESIAN_POINT ( 'NONE',  ( -32.50000000000000000, 34.60000000546236976, 10.55989012756946366 ) ) ;
#31378=CARTESIAN_POINT ( 'NONE',  ( -33.58253175000000113, 63.22500000273119269, 10.91162601494193929 ) ) ;
#31384=CARTESIAN_POINT ( 'NONE',  ( 33.58253175000000113, 4.125000002731193938, -4.112674001490185761E-15 ) ) ;
#31395=CARTESIAN_POINT ( 'NONE',  ( 26.29305231718578995, 27.19999999999998863, -19.10302069950538240 ) ) ;
#31405=CARTESIAN_POINT ( 'NONE',  ( -0.3462681986482577523, 67.00000000000001421, -33.37691080753737083 ) ) ;
#31407=CARTESIAN_POINT ( 'NONE',  ( 20.75514604977248467, 36.42500000273118843, -28.56700777964554305 ) ) ;
#31408=CARTESIAN_POINT ( 'NONE',  ( -26.29305231718578995, 64.70000000546237118, 19.10302069950538595 ) ) ;
#31409=CARTESIAN_POINT ( 'NONE',  ( 33.58253175000000113, 52.47500000273117848, -10.91162601494193574 ) ) ;
#31413=CARTESIAN_POINT ( 'NONE',  ( -20.08610463437156923, 56.80000000546240102, 27.64615127144130113 ) ) ;
#31420=CARTESIAN_POINT ( 'NONE',  ( 6.486482029760649416E-15, 31.87500000273119127, 35.31076352940723240 ) ) ;
#31424=CARTESIAN_POINT ( 'NONE',  ( 32.50000000000000000, 19.50000000546238255, -3.980102097228898626E-15 ) ) ;
#31429=CARTESIAN_POINT ( 'NONE',  ( 0.000000000000000000, 52.00000000000000711, 0.000000000000000000 ) ) ;
#31435=CARTESIAN_POINT ( 'NONE',  ( -20.75514604977248112, 61.42500000273118133, 28.56700777964554661 ) ) ;
#31440=DIRECTION ( 'NONE',  ( 0.000000000000000000, 1.000000000000000000, 0.000000000000000000 ) ) ;
#31445=CARTESIAN_POINT ( 'NONE',  ( -33.58253175000000113, 75.47500000273116427, 10.91162601494193929 ) ) ;
#31449=CARTESIAN_POINT ( 'NONE',  ( 10.37757302488624767, 53.72500000273118559, 31.93888565452638417 ) ) ;
#31450=CARTESIAN_POINT ( 'NONE',  ( -33.58253175000000113, 17.27500000273118630, -10.91162601494193218 ) ) ;
#31451=CARTESIAN_POINT ( 'NONE',  ( -33.58253175000000113, 5.475000002731181148, 10.91162601494193929 ) ) ;
#31455=CARTESIAN_POINT ( 'NONE',  ( -32.50000000000000000, 72.60000000546236265, 10.55989012756946366 ) ) ;
#31456=CARTESIAN_POINT ( 'NONE',  ( 17.97732221215932569, 52.00000000000000711, -27.49025280458518239 ) ) ;
#31464=CARTESIAN_POINT ( 'NONE',  ( 10.37757302488624767, 55.97500000273118559, 31.93888565452638417 ) ) ;
#31470=CARTESIAN_POINT ( 'NONE',  ( 10.37757302488624767, 21.72500000273118559, 31.93888565452638417 ) ) ;
#31473=CARTESIAN_POINT ( 'NONE',  ( -32.50000000000000000, 57.89999999999999858, -10.55989012756945300 ) ) ;
#31480=CARTESIAN_POINT ( 'NONE',  ( -10.04305231718579172, 63.60000000000000142, -30.90933677959248982 ) ) ;
#31483=CARTESIAN_POINT ( 'NONE',  ( 10.04305231718578817, 65.90000000546237402, -30.90933677959249337 ) ) ;
#31485=CARTESIAN_POINT ( 'NONE',  ( -32.50000000000000000, 13.99999999999999822, 0.000000000000000000 ) ) ;
#31491=CARTESIAN_POINT ( 'NONE',  ( 33.58253175000000823, 70.02500000273121827, 10.91162601494192863 ) ) ;
#31492=CARTESIAN_POINT ( 'NONE',  ( -33.58253175000000113, 39.27500000273118275, -10.91162601494193218 ) ) ;
#31498=CARTESIAN_POINT ( 'NONE',  ( 10.04305231718579705, 54.59999999999999432, 30.90933677959248982 ) ) ;
#31504=CARTESIAN_POINT ( 'NONE',  ( 6.486482029760649416E-15, 71.87500000273116996, 35.31076352940723240 ) ) ;
#31509=CARTESIAN_POINT ( 'NONE',  ( 6.486482029760649416E-15, 41.62500000273116996, 35.31076352940723240 ) ) ;
#31513=CARTESIAN_POINT ( 'NONE',  ( -32.50000000000000000, 6.500000005462372776, 0.000000000000000000 ) ) ;
#31514=CARTESIAN_POINT ( 'NONE',  ( 3.980102097228898626E-15, 52.00000000000000711, -32.50000000000000000 ) ) ;
#31529=SHAPE_REPRESENTATION ( 'lock nut', ( #1376 ), #10174 ) ;
#31532=CARTESIAN_POINT ( 'NONE',  ( -20.75514604977248823, 57.07500000273117280, -28.56700777964554305 ) ) ;
#31537=CARTESIAN_POINT ( 'NONE',  ( 32.50000000000000711, 74.90000000000000568, 10.55989012756945122 ) ) ;
#31538=CARTESIAN_POINT ( 'NONE',  ( -27.16883889988623935, 15.32500000273116747, 19.73931689729374739 ) ) ;
#31541=CARTESIAN_POINT ( 'NONE',  ( 32.50000000000000711, 35.40000000546237402, 10.55989012756945122 ) ) ;
#31544=ORIENTED_EDGE ( 'NONE', *, *, #14595, .T. ) ;
#31545=CARTESIAN_POINT ( 'NONE',  ( -33.58253175000000113, 61.22500000273118559, 10.91162601494193929 ) ) ;
#31549=CARTESIAN_POINT ( 'NONE',  ( -33.58253175000000113, 3.025000002731184967, -10.91162601494193218 ) ) ;
#31558=CARTESIAN_POINT ( 'NONE',  ( 10.04305231718578817, 23.39999999999999147, -30.90933677959249337 ) ) ;
#31570=CARTESIAN_POINT ( 'NONE',  ( 20.75514604977248467, 32.42500000273116711, -28.56700777964554305 ) ) ;
#31571=FACE_OUTER_BOUND ( 'NONE', #25775, .T. ) ;
#31575=CARTESIAN_POINT ( 'NONE',  ( 26.29305231718579350, 57.30000000546238681, 19.10302069950537529 ) ) ;
#31582=CARTESIAN_POINT ( 'NONE',  ( -33.58253175000000113, 31.27500000273118275, -10.91162601494193218 ) ) ;
#31586=CARTESIAN_POINT ( 'NONE',  ( 10.04305231718579705, 17.10000000546236976, 30.90933677959248982 ) ) ;
#31587=ADVANCED_FACE ( 'NONE', ( #7820, #18309 ), #5251, .F. ) ;
#31597=CARTESIAN_POINT ( 'NONE',  ( 33.58253175000000113, 60.22500000273119980, -10.91162601494193574 ) ) ;
#31608=CARTESIAN_POINT ( 'NONE',  ( -33.58253175000000113, 77.47500000273120691, 10.91162601494193929 ) ) ;
#31610=VECTOR ( 'NONE', #6200, 1000.000000000000000 ) ;
#31613=CARTESIAN_POINT ( 'NONE',  ( -10.37757302488624411, 56.72500000273118559, -31.93888565452638417 ) ) ;
#31614=CARTESIAN_POINT ( 'NONE',  ( 33.58253175000000113, 18.37500000273119127, -4.112674001490185761E-15 ) ) ;
#31615=CARTESIAN_POINT ( 'NONE',  ( -20.75514604977248112, 1.675000002731184434, 28.56700777964554661 ) ) ;
#31619=CARTESIAN_POINT ( 'NONE',  ( -26.29305231718578995, 70.70000000546238539, 19.10302069950538595 ) ) ;
#31625=ORIENTED_EDGE ( 'NONE', *, *, #5711, .F. ) ;
#31626=CARTESIAN_POINT ( 'NONE',  ( 33.58253175000000823, 46.27500000273120406, 10.91162601494192863 ) ) ;
#31631=CARTESIAN_POINT ( 'NONE',  ( -10.37757302488623701, 25.52500000273118275, 31.93888565452638417 ) ) ;
#31633=VERTEX_POINT ( 'NONE', #6082 ) ;
#31645=CARTESIAN_POINT ( 'NONE',  ( 32.50000000000000000, 65.60000000546239107, -10.55989012756945833 ) ) ;
#31647=CARTESIAN_POINT ( 'NONE',  ( -26.29305231718579350, 17.79999999999999716, -19.10302069950537884 ) ) ;
#31654=CARTESIAN_POINT ( 'NONE',  ( 33.58253175000000113, 72.22500000273119269, -10.91162601494193751 ) ) ;
#31655=CARTESIAN_POINT ( 'NONE',  ( -33.58253175000000113, 35.37500000273117706, 0.000000000000000000 ) ) ;
#31661=CARTESIAN_POINT ( 'NONE',  ( -20.08610463437156923, 54.30000000000000426, 27.64615127144130113 ) ) ;
#31667=CARTESIAN_POINT ( 'NONE',  ( -20.75514604977248823, 73.07500000273115859, -28.56700777964554305 ) ) ;
#31668=CARTESIAN_POINT ( 'NONE',  ( 1.093617666956751375E-13, 61.50000000000000711, -32.50000000000000711 ) ) ;
#31671=ORIENTED_EDGE ( 'NONE', *, *, #6933, .T. ) ;
#31672=CARTESIAN_POINT ( 'NONE',  ( 27.16883889988623935, 42.32500000273119412, -19.73931689729374384 ) ) ;
#31676=CARTESIAN_POINT ( 'NONE',  ( -2.162160676586882350E-15, 66.87500000273119838, -35.31076352940722529 ) ) ;
#31677=CARTESIAN_POINT ( 'NONE',  ( 20.08610463437157279, 5.800000005462378816, -27.64615127144129758 ) ) ;
#31684=CARTESIAN_POINT ( 'NONE',  ( 0.000000000000000000, 52.00000000000000711, 0.000000000000000000 ) ) ;
#31692=FACE_OUTER_BOUND ( 'NONE', #29669, .T. ) ;
#31697=CARTESIAN_POINT ( 'NONE',  ( 20.75514604977248467, 54.67500000273119554, -28.56700777964554305 ) ) ;
#31699=LINE ( 'NONE', #8192, #23485 ) ;
#31700=EDGE_CURVE ( 'NONE', #6717, #13108, #13490, .T. ) ;
#31704=CARTESIAN_POINT ( 'NONE',  ( 32.50000000000000000, 73.00000000000000000, -3.980102097228898626E-15 ) ) ;
#31705=CARTESIAN_POINT ( 'NONE',  ( 6.486482029760649416E-15, 13.62500000273118417, 35.31076352940723240 ) ) ;
#31709=CARTESIAN_POINT ( 'NONE',  ( -26.29305231718578995, 34.70000000546237828, 19.10302069950538595 ) ) ;
#31710=CARTESIAN_POINT ( 'NONE',  ( 1.093617666956751375E-13, 61.50000000000000711, -32.50000000000000711 ) ) ;
#31714=CARTESIAN_POINT ( 'NONE',  ( 6.486482029760649416E-15, 65.62500000273116996, 35.31076352940723240 ) ) ;
#31718=CARTESIAN_POINT ( 'NONE',  ( -20.75514604977248112, 5.425000002731182214, 28.56700777964554661 ) ) ;
#31723=( BOUNDED_CURVE ( )  B_SPLINE_CURVE ( 2, ( #9977, #30904, #27189, #15133, #24611, #30082, #24775, #8993, #7398, #30251, #6754, #3681, #17234 ),
 .UNSPECIFIED., .F., .T. ) 
 B_SPLINE_CURVE_WITH_KNOTS ( ( 3, 2, 2, 2, 2, 2, 3 ),
 ( 0.2628205128205128305, 0.2641025641025641080, 0.2666666666666666630, 0.2692307692307692180, 0.2717948717948717730, 0.2743589743589743835, 0.2756410256410256610 ),
 .UNSPECIFIED. ) 
 CURVE ( )  GEOMETRIC_REPRESENTATION_ITEM ( )  RATIONAL_B_SPLINE_CURVE ( ( 0.9755282581475768211, 0.9755282581475768211, 1.000000000000000000, 0.9510565162951535312, 1.000000000000000000, 0.9510565162951535312, 1.000000000000000000, 0.9510565162951535312, 1.000000000000000000, 0.9510565162951535312, 1.000000000000000000, 0.9755282581475768211, 0.9755282581475768211 ) ) 
 REPRESENTATION_ITEM ( '' )  );
#31727=CARTESIAN_POINT ( 'NONE',  ( 10.04305231718579705, 24.59999999999999787, 30.90933677959248982 ) ) ;
#31731=CARTESIAN_POINT ( 'NONE',  ( -26.85105675556549087, 66.99999999999997158, 19.27006841923039104 ) ) ;
#31738=CARTESIAN_POINT ( 'NONE',  ( 9.638965394428042899, 66.99999999999995737, -31.78062433674936571 ) ) ;
#31739=CARTESIAN_POINT ( 'NONE',  ( -13.42768774669675125, 52.00000000000000000, 30.32522641246977457 ) ) ;
#31740=CARTESIAN_POINT ( 'NONE',  ( 27.16883889988624290, 35.92500000273117422, 19.73931689729373673 ) ) ;
#31745=CARTESIAN_POINT ( 'NONE',  ( 32.50000000000000711, 51.40000000546238823, 10.55989012756945122 ) ) ;
#31751=CARTESIAN_POINT ( 'NONE',  ( 20.75514604977249178, 30.07500000273118701, 28.56700777964553950 ) ) ;
#31753=ORIENTED_EDGE ( 'NONE', *, *, #14029, .T. ) ;
#31755=CARTESIAN_POINT ( 'NONE',  ( -10.04305231718579172, 14.10000000546239640, -30.90933677959248982 ) ) ;
#31764=CARTESIAN_POINT ( 'NONE',  ( 27.16883889988623935, 52.32500000273120122, -19.73931689729374384 ) ) ;
#31774=CARTESIAN_POINT ( 'NONE',  ( 33.58253175000000113, 66.37500000273121259, -4.112674001490185761E-15 ) ) ;
#31778=CARTESIAN_POINT ( 'NONE',  ( -27.16883889988624290, 56.92500000273119554, -19.73931689729374028 ) ) ;
#31779=CARTESIAN_POINT ( 'NONE',  ( -10.37757302488623701, 7.775000002731194293, 31.93888565452638417 ) ) ;
#31780=CARTESIAN_POINT ( 'NONE',  ( -33.58253175000000113, 1.475000002731190474, 10.91162601494193929 ) ) ;
#31785=CARTESIAN_POINT ( 'NONE',  ( -32.50000000000000000, 76.40000000546235981, -10.55989012756945478 ) ) ;
#31793=CARTESIAN_POINT ( 'NONE',  ( 20.75514604977248467, 46.67500000273118133, -28.56700777964554305 ) ) ;
#31798=CARTESIAN_POINT ( 'NONE',  ( 27.16883889988623935, 20.32500000273117280, -19.73931689729374384 ) ) ;
#31812=CARTESIAN_POINT ( 'NONE',  ( 32.50000000000000711, 65.40000000546237402, 10.55989012756945122 ) ) ;
#31814=CARTESIAN_POINT ( 'NONE',  ( -32.50000000000000000, 12.09999999999999787, 10.55989012756946366 ) ) ;
#31821=CARTESIAN_POINT ( 'NONE',  ( -27.16883889988624290, 72.92500000273120975, -19.73931689729374028 ) ) ;
#31822=CARTESIAN_POINT ( 'NONE',  ( -27.16883889988623935, 35.57500000273118701, 19.73931689729374739 ) ) ;
#31827=CARTESIAN_POINT ( 'NONE',  ( 32.50000000000000000, 51.09999999999998721, -10.55989012756945833 ) ) ;
#31832=CARTESIAN_POINT ( 'NONE',  ( -20.75514604977248112, 69.67500000273119554, 28.56700777964554661 ) ) ;
#31837=CARTESIAN_POINT ( 'NONE',  ( -20.75514604977248823, 36.82500000273117990, -28.56700777964554305 ) ) ;
#31842=CARTESIAN_POINT ( 'NONE',  ( -32.50000000000000000, 60.40000000546236691, -10.55989012756945300 ) ) ;
#31843=CARTESIAN_POINT ( 'NONE',  ( -32.50000000000000000, 0.5000000054623809920, 0.000000000000000000 ) ) ;
#31860=CARTESIAN_POINT ( 'NONE',  ( 10.37757302488624056, 54.77500000273121117, -31.93888565452638417 ) ) ;
#31862=DIRECTION ( 'NONE',  ( 0.000000000000000000, 1.000000000000000000, 0.000000000000000000 ) ) ;
#31866=CARTESIAN_POINT ( 'NONE',  ( -20.08610463437156923, 72.30000000000002558, 27.64615127144130113 ) ) ;
#31867=CARTESIAN_POINT ( 'NONE',  ( 33.58253175000000823, 8.025000002731188076, 10.91162601494192863 ) ) ;
#31875=CARTESIAN_POINT ( 'NONE',  ( 33.58253175000000823, 64.02500000273118985, 10.91162601494192863 ) ) ;
#31880=CARTESIAN_POINT ( 'NONE',  ( -20.75514604977248112, 7.425000002731191984, 28.56700777964554661 ) ) ;
#31890=CARTESIAN_POINT ( 'NONE',  ( -10.04305231718579172, 23.59999999999999432, -30.90933677959248982 ) ) ;
#31902=CARTESIAN_POINT ( 'NONE',  ( -28.18730216971796310, 52.00000000000000711, 16.82255561449002457 ) ) ;
#31904=CARTESIAN_POINT ( 'NONE',  ( -27.16883889988623935, 31.32500000273118346, 19.73931689729374739 ) ) ;
#31905=CARTESIAN_POINT ( 'NONE',  ( 32.50000000000000000, 64.99999999999998579, -3.980102097228898626E-15 ) ) ;
#31909=CARTESIAN_POINT ( 'NONE',  ( 26.29305231718579350, 53.30000000546237970, 19.10302069950537529 ) ) ;
#31922=CARTESIAN_POINT ( 'NONE',  ( 32.50000000000000000, 17.60000000546238397, -10.55989012756945833 ) ) ;
#31932=CARTESIAN_POINT ( 'NONE',  ( 33.58253175000000113, 56.22500000273117138, -10.91162601494193574 ) ) ;
#31942=CARTESIAN_POINT ( 'NONE',  ( -33.58253175000000113, 65.47500000273117848, 10.91162601494193929 ) ) ;
#31946=CARTESIAN_POINT ( 'NONE',  ( 27.16883889988623935, 56.32500000273120122, -19.73931689729374384 ) ) ;
#31947=CARTESIAN_POINT ( 'NONE',  ( 27.16883889988624290, 12.17500000273118133, 19.73931689729373673 ) ) ;
#31948=CARTESIAN_POINT ( 'NONE',  ( 20.75514604977249178, 62.07500000273119412, 28.56700777964553950 ) ) ;
#31953=CARTESIAN_POINT ( 'NONE',  ( 32.50000000000000000, 75.60000000546236265, -10.55989012756945833 ) ) ;
#31960=CARTESIAN_POINT ( 'NONE',  ( -2.162160676586881955E-15, 50.87500000273119838, -35.31076352940723240 ) ) ;
#31966=CARTESIAN_POINT ( 'NONE',  ( -10.37757302488623701, 15.52500000273120051, 31.93888565452638417 ) ) ;
#31980=CARTESIAN_POINT ( 'NONE',  ( 10.04305231718578817, 13.40000000000000924, -30.90933677959249337 ) ) ;
#31986=CARTESIAN_POINT ( 'NONE',  ( 6.486482029760649416E-15, 75.62500000273121259, 35.31076352940723240 ) ) ;
#31987=CARTESIAN_POINT ( 'NONE',  ( 27.16883889988624290, 30.17500000273119909, 19.73931689729373673 ) ) ;
#31994=CARTESIAN_POINT ( 'NONE',  ( -32.50000000000000000, 55.90000000000000568, -10.55989012756945478 ) ) ;
#31999=CARTESIAN_POINT ( 'NONE',  ( 10.37757302488624056, 64.77500000273118985, -31.93888565452638417 ) ) ;
#32000=CARTESIAN_POINT ( 'NONE',  ( -32.50000000000000000, 61.89999999999999147, -10.55989012756945300 ) ) ;
#32004=CARTESIAN_POINT ( 'NONE',  ( -10.37757302488624411, 38.72500000273119980, -31.93888565452638417 ) ) ;
#32009=CARTESIAN_POINT ( 'NONE',  ( -5.147494310547377161, 60.05125428700922896, -32.50000000000002132 ) ) ;
#32022=EDGE_CURVE ( 'NONE', #9005, #20850, #31723, .T. ) ;
#32028=CARTESIAN_POINT ( 'NONE',  ( -33.58253175000000113, 47.47500000273119269, 10.91162601494193929 ) ) ;
#32034=CARTESIAN_POINT ( 'NONE',  ( 20.08610463437158344, 70.70000000000000284, 27.64615127144129403 ) ) ;
#32035=CARTESIAN_POINT ( 'NONE',  ( 10.37757302488624767, 9.725000002731173154, 31.93888565452638417 ) ) ;
#32043=CARTESIAN_POINT ( 'NONE',  ( -33.58253175000000113, 55.22500000273117848, 10.91162601494193929 ) ) ;
#32059=CARTESIAN_POINT ( 'NONE',  ( -26.29305231718578995, 22.19999999999998508, 19.10302069950538595 ) ) ;
#32069=CARTESIAN_POINT ( 'NONE',  ( 30.22248186753583710, 66.99999999999998579, -12.55019540181426052 ) ) ;
#32072=CARTESIAN_POINT ( 'NONE',  ( -33.58253175000000113, 31.12500000273120548, 0.000000000000000000 ) ) ;
#32073=CARTESIAN_POINT ( 'NONE',  ( -1.053607264507113999E-13, 64.50000000000000000, 32.50000000000000711 ) ) ;
#32074=CARTESIAN_POINT ( 'NONE',  ( 32.50000000000000000, 61.60000000546236265, -10.55989012756945833 ) ) ;
#32078=CARTESIAN_POINT ( 'NONE',  ( -32.50000000000000000, 48.40000000546237402, -10.55989012756945478 ) ) ;
#32084=CARTESIAN_POINT ( 'NONE',  ( -33.58253175000000113, 73.12500000273118417, 0.000000000000000000 ) ) ;
#32089=CARTESIAN_POINT ( 'NONE',  ( -10.04305231718579172, 20.10000000546237331, -30.90933677959248982 ) ) ;
#32104=DIRECTION ( 'NONE',  ( 0.000000000000000000, 0.000000000000000000, 1.000000000000000000 ) ) ;
#32105=CARTESIAN_POINT ( 'NONE',  ( -2.162160676586881955E-15, 70.87500000273118417, -35.31076352940723240 ) ) ;
#32106=ORIENTED_EDGE ( 'NONE', *, *, #25184, .T. ) ;
#32112=CARTESIAN_POINT ( 'NONE',  ( -10.37757302488623701, 45.52500000273117564, 31.93888565452638417 ) ) ;
#32113=CARTESIAN_POINT ( 'NONE',  ( -10.37757302488624411, 10.97500000273120335, -31.93888565452638417 ) ) ;
#32114=CARTESIAN_POINT ( 'NONE',  ( -33.58253175000000113, 63.27500000273118985, -10.91162601494193041 ) ) ;
#32120=CARTESIAN_POINT ( 'NONE',  ( -32.50000000000000000, 68.60000000546237686, 10.55989012756946366 ) ) ;
#32127=CARTESIAN_POINT ( 'NONE',  ( -2.162160676586881955E-15, 48.87500000273117706, -35.31076352940723240 ) ) ;
#32129=MANIFOLD_SOLID_BREP ( 'Cavity1', #10105 ) ;
#32133=CARTESIAN_POINT ( 'NONE',  ( 20.75514604977248467, 20.42500000273120619, -28.56700777964554305 ) ) ;
#32146=CARTESIAN_POINT ( 'NONE',  ( 10.04305231718579705, 65.10000000546239107, 30.90933677959248982 ) ) ;
#32149=CARTESIAN_POINT ( 'NONE',  ( 26.29305231718578995, 13.20000000000000284, -19.10302069950538240 ) ) ;
#32155=CARTESIAN_POINT ( 'NONE',  ( -10.37757302488624411, 66.72500000273116427, -31.93888565452638417 ) ) ;
#32156=CARTESIAN_POINT ( 'NONE',  ( 20.75514604977248467, 32.67500000273118843, -28.56700777964554305 ) ) ;
#32157=CARTESIAN_POINT ( 'NONE',  ( -33.58253175000000113, 15.47500000273118381, 10.91162601494193929 ) ) ;
#32164=CARTESIAN_POINT ( 'NONE',  ( 10.04305231718578817, 53.39999999999999147, -30.90933677959249337 ) ) ;
#32170=CARTESIAN_POINT ( 'NONE',  ( -27.16883889988623935, 65.57500000273118701, 19.73931689729374739 ) ) ;
#32175=CARTESIAN_POINT ( 'NONE',  ( -20.75514604977248112, 35.42500000273119554, 28.56700777964554661 ) ) ;
#32179=CARTESIAN_POINT ( 'NONE',  ( 33.58253175000000823, 66.27500000273117564, 10.91162601494192685 ) ) ;
#32180=CARTESIAN_POINT ( 'NONE',  ( 26.29305231718578995, 59.20000000000001705, -19.10302069950538240 ) ) ;
#32197=CARTESIAN_POINT ( 'NONE',  ( -2.162160676586881955E-15, 46.87500000273118417, -35.31076352940723240 ) ) ;
#32200=VECTOR ( 'NONE', #15875, 1000.000000000000000 ) ;
#32203=CARTESIAN_POINT ( 'NONE',  ( 32.50000000000000711, 70.90000000000000568, 10.55989012756945122 ) ) ;
#32204=CARTESIAN_POINT ( 'NONE',  ( -10.37757302488624411, 10.72500000273117493, -31.93888565452638417 ) ) ;
#32206=EDGE_CURVE ( 'NONE', #9681, #9005, #2153, .T. ) ;
#32213=EDGE_CURVE ( 'NONE', #11742, #10580, #8743, .T. ) ;
#32215=CARTESIAN_POINT ( 'NONE',  ( -20.75514604977248112, 55.42500000273119554, 28.56700777964554661 ) ) ;
#32221=CARTESIAN_POINT ( 'NONE',  ( -33.58253175000000113, 1.225000002731198467, 10.91162601494193929 ) ) ;
#32243=CARTESIAN_POINT ( 'NONE',  ( 10.37757302488624056, 30.52500000273118630, -31.93888565452638417 ) ) ;
#32249=CARTESIAN_POINT ( 'NONE',  ( 26.29305231718578995, 49.70000000546236407, -19.10302069950538240 ) ) ;
#32252=CARTESIAN_POINT ( 'NONE',  ( -20.75514604977248823, 72.82500000273118701, -28.56700777964554305 ) ) ;
#32257=CARTESIAN_POINT ( 'NONE',  ( 32.50000000000000711, 9.400000005462366914, 10.55989012756945122 ) ) ;
#32274=CARTESIAN_POINT ( 'NONE',  ( 10.37757302488624056, 70.77500000273118985, -31.93888565452638417 ) ) ;
#32279=CARTESIAN_POINT ( 'NONE',  ( -10.37757302488624411, 48.72500000273120691, -31.93888565452638417 ) ) ;
#32280=CARTESIAN_POINT ( 'NONE',  ( 10.37757302488624056, 10.77500000273116854, -31.93888565452638417 ) ) ;
#32281=CARTESIAN_POINT ( 'NONE',  ( 6.486482029760648627E-15, 61.87500000273117706, 35.31076352940722529 ) ) ;
#32285=CARTESIAN_POINT ( 'NONE',  ( -26.29305231718579350, 68.30000000546236549, -19.10302069950537884 ) ) ;
#32291=CARTESIAN_POINT ( 'NONE',  ( 10.37757302488624767, 47.97500000273117848, 31.93888565452638417 ) ) ;
#32296=CARTESIAN_POINT ( 'NONE',  ( 27.16883889988624290, 17.92500000273118843, 19.73931689729373673 ) ) ;
#32315=CARTESIAN_POINT ( 'NONE',  ( 10.04305231718579705, 10.59999999999998366, 30.90933677959248982 ) ) ;
#32321=CARTESIAN_POINT ( 'NONE',  ( 20.75514604977248467, 68.42500000273120975, -28.56700777964554305 ) ) ;
#32322=CARTESIAN_POINT ( 'NONE',  ( 27.16883889988623935, 32.57500000273117990, -19.73931689729374384 ) ) ;
#32323=CARTESIAN_POINT ( 'NONE',  ( 20.75514604977248467, 18.67500000273120264, -28.56700777964554305 ) ) ;
#32329=CARTESIAN_POINT ( 'NONE',  ( -20.08610463437156923, 48.30000000000001847, 27.64615127144130113 ) ) ;
#32334=CARTESIAN_POINT ( 'NONE',  ( -33.58253175000000113, 67.47500000273117848, 10.91162601494193929 ) ) ;
#32335=CARTESIAN_POINT ( 'NONE',  ( 5.779280353836490358E-15, 62.50000000000000000, 32.49999999999999289 ) ) ;
#32339=CARTESIAN_POINT ( 'NONE',  ( -10.37757302488623701, 35.52500000273118985, 31.93888565452638417 ) ) ;
#32361=CARTESIAN_POINT ( 'NONE',  ( 27.16883889988623935, 48.57500000273119412, -19.73931689729374384 ) ) ;
#32367=CARTESIAN_POINT ( 'NONE',  ( -26.29305231718579350, 69.80000000000001137, -19.10302069950537884 ) ) ;
#32368=CARTESIAN_POINT ( 'NONE',  ( -27.16883889988624290, 10.92500000273120797, -19.73931689729374028 ) ) ;
#32377=CARTESIAN_POINT ( 'NONE',  ( -33.58253175000000113, 59.22500000273119269, 10.91162601494193929 ) ) ;
#32378=CARTESIAN_POINT ( 'NONE',  ( -20.75514604977248112, 29.67500000273119909, 28.56700777964554661 ) ) ;
#32405=CARTESIAN_POINT ( 'NONE',  ( 33.58253175000000823, 26.02500000273120406, 10.91162601494192863 ) ) ;
#32411=CARTESIAN_POINT ( 'NONE',  ( 26.29305231718579350, 47.30000000546237260, 19.10302069950537529 ) ) ;
#32416=CARTESIAN_POINT ( 'NONE',  ( 10.37757302488624056, 72.52500000273118985, -31.93888565452638417 ) ) ;
#32421=CARTESIAN_POINT ( 'NONE',  ( -26.29305231718578995, 10.70000000546238184, 19.10302069950538595 ) ) ;
#32431=CARTESIAN_POINT ( 'NONE',  ( -20.08610463437156923, 36.29999999999997584, 27.64615127144130113 ) ) ;
#32439=CARTESIAN_POINT ( 'NONE',  ( -10.37757302488623701, 69.77500000273118985, 31.93888565452638417 ) ) ;
#32443=VECTOR ( 'NONE', #12716, 1000.000000000000114 ) ;
#32444=CARTESIAN_POINT ( 'NONE',  ( -33.58253175000000113, 47.02500000273116854, -10.91162601494193218 ) ) ;
#32445=CARTESIAN_POINT ( 'NONE',  ( 33.58253175000000113, 10.47500000273118204, -10.91162601494193751 ) ) ;
#32446=CARTESIAN_POINT ( 'NONE',  ( 27.16883889988624290, 60.17500000273119554, 19.73931689729373673 ) ) ;
#32450=CARTESIAN_POINT ( 'NONE',  ( -32.50000000000000000, 66.40000000546238823, -10.55989012756945478 ) ) ;
#32456=CARTESIAN_POINT ( 'NONE',  ( 20.75514604977249178, 44.07500000273117990, 28.56700777964553950 ) ) ;
#32458=CARTESIAN_POINT ( 'NONE',  ( 10.04305231718578817, 27.90000000546237402, -30.90933677959249337 ) ) ;
#32460=CARTESIAN_POINT ( 'NONE',  ( 33.58253175000000823, 16.02500000273119340, 10.91162601494192863 ) ) ;
#32476=CARTESIAN_POINT ( 'NONE',  ( -32.50000000000000000, 9.999999999999994671, 0.000000000000000000 ) ) ;
#32482=CARTESIAN_POINT ( 'NONE',  ( -2.162160676586881955E-15, 64.62500000273121259, -35.31076352940723240 ) ) ;
#32483=CARTESIAN_POINT ( 'NONE',  ( -20.75514604977248112, 29.67500000273119909, 28.56700777964554661 ) ) ;
#32484=CARTESIAN_POINT ( 'NONE',  ( -10.37757302488624411, 16.97500000273118204, -31.93888565452638417 ) ) ;
#32492=CARTESIAN_POINT ( 'NONE',  ( -26.29305231718578995, 50.20000000000000995, 19.10302069950538595 ) ) ;
#32498=CARTESIAN_POINT ( 'NONE',  ( -2.162160676586881955E-15, 62.87500000273120548, -35.31076352940723240 ) ) ;
#32502=CARTESIAN_POINT ( 'NONE',  ( 27.16883889988624290, 37.92500000273117422, 19.73931689729373673 ) ) ;
#32507=CARTESIAN_POINT ( 'NONE',  ( -10.04305231718578462, 0.9000000054623785717, 30.90933677959249337 ) ) ;
#32524=CARTESIAN_POINT ( 'NONE',  ( -10.37757302488623701, 51.77500000273120406, 31.93888565452638417 ) ) ;
#32531=CARTESIAN_POINT ( 'NONE',  ( -20.08610463437157989, 67.70000000000000284, -27.64615127144129758 ) ) ;
#32532=CARTESIAN_POINT ( 'NONE',  ( 27.16883889988623935, 10.32500000273119056, -19.73931689729374384 ) ) ;
#32537=CARTESIAN_POINT ( 'NONE',  ( -5.147494310547430452, 65.55125428154684641, -32.49999999999999289 ) ) ;
#32543=CARTESIAN_POINT ( 'NONE',  ( -27.16883889988624290, 54.92500000273118843, -19.73931689729374028 ) ) ;
#32544=CARTESIAN_POINT ( 'NONE',  ( -2.162160676586881955E-15, 26.87500000273116996, -35.31076352940723240 ) ) ;
#32558=CARTESIAN_POINT ( 'NONE',  ( 6.486482029760648627E-15, 53.62500000273120548, 35.31076352940722529 ) ) ;
#32571=CARTESIAN_POINT ( 'NONE',  ( -32.46022989551241977, 52.00000000000002842, 2.703243202363978526 ) ) ;
#32573=CARTESIAN_POINT ( 'NONE',  ( -20.75514604977248112, 25.42500000273119198, 28.56700777964554661 ) ) ;
#32578=CARTESIAN_POINT ( 'NONE',  ( 32.50000000000000711, 47.40000000546237402, 10.55989012756945122 ) ) ;
#32581=ORIENTED_EDGE ( 'NONE', *, *, #16639, .F. ) ;
#32582=CARTESIAN_POINT ( 'NONE',  ( 20.75514604977249178, 77.82500000273120122, 28.56700777964553950 ) ) ;
#32588=CARTESIAN_POINT ( 'NONE',  ( -2.092463501923844636E-15, 12.00000000546237189, -34.17252228774368916 ) ) ;
#32597=CARTESIAN_POINT ( 'NONE',  ( 32.50000000000000711, 36.89999999999999858, 10.55989012756945122 ) ) ;
#32608=VECTOR ( 'NONE', #16087, 1000.000000000000000 ) ;
#32612=CARTESIAN_POINT ( 'NONE',  ( 10.37757302488624056, 46.52500000273117564, -31.93888565452638417 ) ) ;
#32613=CARTESIAN_POINT ( 'NONE',  ( 10.37757302488624767, 3.975000002731182924, 31.93888565452638417 ) ) ;
#32614=CARTESIAN_POINT ( 'NONE',  ( 33.58253175000000113, 64.47500000273120691, -10.91162601494193574 ) ) ;
#32618=CARTESIAN_POINT ( 'NONE',  ( 32.50000000000000000, 67.50000000546239676, -3.980102097228898626E-15 ) ) ;
#32625=CARTESIAN_POINT ( 'NONE',  ( -27.16883889988624290, 41.17500000273118133, -19.73931689729374028 ) ) ;
#32626=CARTESIAN_POINT ( 'NONE',  ( 1.076200423132605543E-16, 66.99999999999998579, -46.18802153517007980 ) ) ;
#32627=CARTESIAN_POINT ( 'NONE',  ( 32.50000000000000000, 29.60000000546238041, -10.55989012756945833 ) ) ;
#32647=CARTESIAN_POINT ( 'NONE',  ( 32.50000000000000000, 3.000000000000002665, -3.980102097228898626E-15 ) ) ;
#32652=CARTESIAN_POINT ( 'NONE',  ( -10.37757302488623701, 63.52500000273118985, 31.93888565452638417 ) ) ;
#32653=CARTESIAN_POINT ( 'NONE',  ( 10.37757302488624767, 27.97500000273118914, 31.93888565452638417 ) ) ;
#32654=CARTESIAN_POINT ( 'NONE',  ( 27.16883889988624290, 16.17500000273118488, 19.73931689729373673 ) ) ;
#32660=CARTESIAN_POINT ( 'NONE',  ( 32.50000000000000000, 49.00000000000000000, -3.980102097228898626E-15 ) ) ;
#32665=CARTESIAN_POINT ( 'NONE',  ( 33.58253175000000113, 58.47500000273118559, -10.91162601494193751 ) ) ;
#32670=CARTESIAN_POINT ( 'NONE',  ( -2.162160676586881955E-15, 28.62500000273118062, -35.31076352940723240 ) ) ;
#32671=VERTEX_POINT ( 'NONE', #31710 ) ;
#32691=CARTESIAN_POINT ( 'NONE',  ( -10.37757302488623701, 47.77500000273120406, 31.93888565452638417 ) ) ;
#32697=CARTESIAN_POINT ( 'NONE',  ( -32.50000000000000000, 64.10000000000000853, 10.55989012756946366 ) ) ;
#32706=CARTESIAN_POINT ( 'NONE',  ( 6.486482029760649416E-15, 53.62500000273119838, 35.31076352940723240 ) ) ;
#32707=CARTESIAN_POINT ( 'NONE',  ( -27.16883889988624290, 29.17500000273119554, -19.73931689729374028 ) ) ;
#32722=CARTESIAN_POINT ( 'NONE',  ( 6.486482029760648627E-15, 57.62500000273119127, 35.31076352940722529 ) ) ;
#32739=CARTESIAN_POINT ( 'NONE',  ( -33.58253175000000113, 19.12500000273119483, 0.000000000000000000 ) ) ;
#32744=CARTESIAN_POINT ( 'NONE',  ( -10.04305231718578462, 48.90000000546239534, 30.90933677959249337 ) ) ;
#32749=CARTESIAN_POINT ( 'NONE',  ( 20.75514604977248467, 76.42500000273118133, -28.56700777964554305 ) ) ;
#32752=DIRECTION ( 'NONE',  ( 0.000000000000000000, 1.000000000000000000, 0.000000000000000000 ) ) ;
#32755=CARTESIAN_POINT ( 'NONE',  ( -26.29305231718579350, 12.30000000546237260, -19.10302069950537884 ) ) ;
#32765=CARTESIAN_POINT ( 'NONE',  ( 26.29305231718578995, 35.19999999999999574, -19.10302069950538240 ) ) ;
#32777=CARTESIAN_POINT ( 'NONE',  ( -20.75514604977248112, 45.42500000273119554, 28.56700777964554661 ) ) ;
#32778=CARTESIAN_POINT ( 'NONE',  ( 33.58253175000000113, 6.375000002731182391, -4.112674001490185761E-15 ) ) ;
#32779=CARTESIAN_POINT ( 'NONE',  ( -27.16883889988623935, 53.57500000273117280, 19.73931689729374739 ) ) ;
#32783=CARTESIAN_POINT ( 'NONE',  ( -32.50000000000000000, 64.60000000546237686, 10.55989012756946366 ) ) ;
#32784=EDGE_CURVE ( 'NONE', #2770, #18447, #29314, .T. ) ;
#32787=LINE ( 'NONE', #9118, #7242 ) ;
#32790=CARTESIAN_POINT ( 'NONE',  ( -2.162160676586881955E-15, 38.87500000273120548, -35.31076352940723240 ) ) ;
#32792=CARTESIAN_POINT ( 'NONE',  ( -26.29305231718579350, 30.30000000546238681, -19.10302069950537884 ) ) ;
#32793=VERTEX_POINT ( 'NONE', #8868 ) ;
#32800=CARTESIAN_POINT ( 'NONE',  ( -2.162160676586882350E-15, 66.62500000273119838, -35.31076352940722529 ) ) ;
#32809=DIRECTION ( 'NONE',  ( 0.000000000000000000, 0.000000000000000000, 1.000000000000000000 ) ) ;
#32810=CARTESIAN_POINT ( 'NONE',  ( -32.50000000000000000, 5.900000000000002132, -10.55989012756945478 ) ) ;
#32815=CARTESIAN_POINT ( 'NONE',  ( -2.162160676586881955E-15, 68.62500000273119838, -35.31076352940723240 ) ) ;
#32817=CARTESIAN_POINT ( 'NONE',  ( -2.162160676586881955E-15, 26.87500000273116996, -35.31076352940723240 ) ) ;
#32818=CARTESIAN_POINT ( 'NONE',  ( 20.75514604977248467, 14.67500000273117955, -28.56700777964554305 ) ) ;
#32824=CARTESIAN_POINT ( 'NONE',  ( -32.50000000000000000, 49.89999999999999147, -10.55989012756945478 ) ) ;
#32829=ORIENTED_EDGE ( 'NONE', *, *, #5711, .T. ) ;
#32830=CARTESIAN_POINT ( 'NONE',  ( 20.75514604977248467, 62.67500000273117422, -28.56700777964554305 ) ) ;
#32835=CARTESIAN_POINT ( 'NONE',  ( -10.37757302488624411, 30.72500000273119269, -31.93888565452638417 ) ) ;
#32855=CARTESIAN_POINT ( 'NONE',  ( -27.16883889988623935, 45.57500000273119412, 19.73931689729374739 ) ) ;
#32860=CARTESIAN_POINT ( 'NONE',  ( 26.29305231718578995, 67.20000000000000284, -19.10302069950538240 ) ) ;
#32870=CARTESIAN_POINT ( 'NONE',  ( -27.16883889988624290, 52.92500000273118843, -19.73931689729374028 ) ) ;
#32871=CARTESIAN_POINT ( 'NONE',  ( -33.58253175000000113, 23.37500000273119838, 0.000000000000000000 ) ) ;
#32885=CARTESIAN_POINT ( 'NONE',  ( -33.58253175000000113, 53.12500000273119838, 0.000000000000000000 ) ) ;
#32895=DIRECTION ( 'NONE',  ( 0.4999999999999998335, 0.000000000000000000, -0.8660254037844387076 ) ) ;
#32900=CARTESIAN_POINT ( 'NONE',  ( 33.58253175000000113, 24.12500000273119838, -4.112674001490185761E-15 ) ) ;
#32902=CARTESIAN_POINT ( 'NONE',  ( 26.29305231718578995, 53.20000000000000995, -19.10302069950538240 ) ) ;
#32905=CARTESIAN_POINT ( 'NONE',  ( 10.04305231718578817, 43.90000000546238823, -30.90933677959249337 ) ) ;
#32912=CARTESIAN_POINT ( 'NONE',  ( -20.75514604977248823, 68.82500000273118701, -28.56700777964554305 ) ) ;
#32918=CARTESIAN_POINT ( 'NONE',  ( -10.04305231718578462, 8.900000005462358033, 30.90933677959249337 ) ) ;
#32928=CARTESIAN_POINT ( 'NONE',  ( 32.50000000000000000, 33.00000000000001421, -3.980102097228898626E-15 ) ) ;
#32942=CARTESIAN_POINT ( 'NONE',  ( -33.58253175000000113, 41.22500000273118559, 10.91162601494193929 ) ) ;
#32943=CARTESIAN_POINT ( 'NONE',  ( -33.58253175000000113, 3.375000002731193049, 0.000000000000000000 ) ) ;
#32944=CARTESIAN_POINT ( 'NONE',  ( 10.37757302488624767, 53.97500000273118559, 31.93888565452638417 ) ) ;
#32947=CARTESIAN_POINT ( 'NONE',  ( 26.29305231718579350, 63.30000000546235839, 19.10302069950537529 ) ) ;
#32950=CARTESIAN_POINT ( 'NONE',  ( -10.04305231718578462, 54.39999999999999147, 30.90933677959249337 ) ) ;
#32951=B_SPLINE_CURVE_WITH_KNOTS ( 'NONE', 3,
 ( #33288, #20435, #15284, #17345, #14767, #25744, #12185, #2226, #7034, #4125, #14600, #17517, #27978, #4463, #324, #10811, #21291, #8060, #28823, #18209, #31731, #18545, #23352, #8222, #4980, #26087, #8390, #28991, #18716, #2745, #13562, #29152, #33814, #28652, #24025, #31230, #5658, #5321, #2407, #15635, #21119, #12875, #494, #10977 ),
 .UNSPECIFIED., .F., .F.,
 ( 4, 2, 2, 2, 2, 2, 2, 2, 2, 2, 2, 2, 2, 2, 2, 2, 2, 2, 2, 2, 2, 4 ),
 ( 0.000000000000000000, 0.004057857163981326565, 0.008115714327962653130, 0.01217357149194398663, 0.01420250007393465339, 0.01623142865592532014, 0.02028928581990665364, 0.02231821440189732039, 0.02434714298388798714, 0.02840500014786932065, 0.03246285731185065415, 0.03652071447583198766, 0.03854964305782265094, 0.04057857163981331422, 0.04463642880379464078, 0.04869428596777596735, 0.05072321454976663063, 0.05275214313175728698, 0.05681000029573861354, 0.05883892887772927682, 0.06086785745971993317, 0.06492571462370128055 ),
 .UNSPECIFIED. ) ;
#32954=CARTESIAN_POINT ( 'NONE',  ( -10.37757302488624411, 40.97500000273117138, -31.93888565452638417 ) ) ;
#32958=CARTESIAN_POINT ( 'NONE',  ( -2.092463501923844636E-15, 28.00000000546237544, -34.17252228774368916 ) ) ;
#32976=CARTESIAN_POINT ( 'NONE',  ( -5.147494310547430452, 55.55125428154683220, -32.49999999999999289 ) ) ;
#32978=CARTESIAN_POINT ( 'NONE',  ( -32.50000000000000000, 2.000000000000001776, 0.000000000000000000 ) ) ;
#32983=CARTESIAN_POINT ( 'NONE',  ( 6.486482029760649416E-15, 61.62500000273118417, 35.31076352940723240 ) ) ;
#32984=CARTESIAN_POINT ( 'NONE',  ( 20.75514604977249178, 26.07500000273119767, 28.56700777964553950 ) ) ;
#32985=CARTESIAN_POINT ( 'NONE',  ( -33.58253175000000113, 11.37500000273118594, 0.000000000000000000 ) ) ;
#32989=CARTESIAN_POINT ( 'NONE',  ( 26.29305231718579350, 44.79999999999999005, 19.10302069950537529 ) ) ;
#32994=CARTESIAN_POINT ( 'NONE',  ( -20.75514604977248112, 61.67500000273117422, 28.56700777964554661 ) ) ;
#33000=CARTESIAN_POINT ( 'NONE',  ( -10.37757302488623701, 33.52500000273118985, 31.93888565452638417 ) ) ;
#33025=CARTESIAN_POINT ( 'NONE',  ( -33.58253175000000113, 43.37500000273118417, 0.000000000000000000 ) ) ;
#33031=CARTESIAN_POINT ( 'NONE',  ( -20.08610463437156923, 66.30000000000001137, 27.64615127144130113 ) ) ;
#33043=CARTESIAN_POINT ( 'NONE',  ( 27.16883889988623935, 48.32500000273119412, -19.73931689729374384 ) ) ;
#33044=CARTESIAN_POINT ( 'NONE',  ( 10.37757302488624056, 24.77500000273118275, -31.93888565452638417 ) ) ;
#33051=EDGE_CURVE ( 'NONE', #4618, #22505, #1636, .T. ) ;
#33068=CARTESIAN_POINT ( 'NONE',  ( -33.58253175000000113, 59.47500000273118559, 10.91162601494193929 ) ) ;
#33076=CARTESIAN_POINT ( 'NONE',  ( -10.37757302488623701, 23.52500000273117919, 31.93888565452638417 ) ) ;
#33083=CARTESIAN_POINT ( 'NONE',  ( -2.092463501923844636E-15, 42.00000000546236834, -34.17252228774368916 ) ) ;
#33086=CARTESIAN_POINT ( 'NONE',  ( -20.75514604977248112, 65.67500000273116711, 28.56700777964554661 ) ) ;
#33089=CARTESIAN_POINT ( 'NONE',  ( -33.58253175000000113, 71.22500000273117848, 10.91162601494193929 ) ) ;
#33095=CARTESIAN_POINT ( 'NONE',  ( 33.58253175000000113, 10.22500000273118914, -10.91162601494193751 ) ) ;
#33103=CARTESIAN_POINT ( 'NONE',  ( 6.277390505771533514E-15, 36.49999999999997868, 34.17252228774368916 ) ) ;
#33109=CARTESIAN_POINT ( 'NONE',  ( 32.50000000000000000, 62.99999999999998579, -3.980102097228898626E-15 ) ) ;
#33118=CARTESIAN_POINT ( 'NONE',  ( 27.16883889988624290, 39.92500000273118133, 19.73931689729373673 ) ) ;
#33119=CARTESIAN_POINT ( 'NONE',  ( -20.75514604977248112, 1.675000002731184434, 28.56700777964554661 ) ) ;
#33120=CARTESIAN_POINT ( 'NONE',  ( 33.58253175000000823, 58.27500000273116854, 10.91162601494192685 ) ) ;
#33123=CARTESIAN_POINT ( 'NONE',  ( -20.08610463437157989, 58.20000000546238539, -27.64615127144129758 ) ) ;
#33129=CARTESIAN_POINT ( 'NONE',  ( -27.16883889988623935, 41.57500000273119412, 19.73931689729374739 ) ) ;
#33134=CARTESIAN_POINT ( 'NONE',  ( 26.29305231718578995, 27.70000000546236762, -19.10302069950538240 ) ) ;
#33143=CARTESIAN_POINT ( 'NONE',  ( -20.75514604977248823, 66.82500000273118701, -28.56700777964554305 ) ) ;
#33153=CYLINDRICAL_SURFACE ( 'NONE', #24984, 32.50000000000000000 ) ;
#33154=CARTESIAN_POINT ( 'NONE',  ( 12.90513655866702081, 52.00000000000000711, 31.00393344628893288 ) ) ;
#33155=ADVANCED_FACE ( 'NONE', ( #9196 ), #10689, .T. ) ;
#33156=CARTESIAN_POINT ( 'NONE',  ( 20.08610463437158344, 6.699999999999991296, 27.64615127144129403 ) ) ;
#33161=CARTESIAN_POINT ( 'NONE',  ( 10.37757302488624767, 61.72500000273119269, 31.93888565452638417 ) ) ;
#33162=CARTESIAN_POINT ( 'NONE',  ( 20.75514604977248467, 24.67500000273118843, -28.56700777964554305 ) ) ;
#33163=CARTESIAN_POINT ( 'NONE',  ( -27.16883889988624290, 9.175000002731179549, -19.73931689729374028 ) ) ;
#33167=CARTESIAN_POINT ( 'NONE',  ( 26.29305231718578995, 77.70000000546238539, -19.10302069950538240 ) ) ;
#33169=CARTESIAN_POINT ( 'NONE',  ( -32.50000000000000000, 39.99999999999999289, 0.000000000000000000 ) ) ;
#33175=CARTESIAN_POINT ( 'NONE',  ( -20.75514604977248823, 63.07500000273119412, -28.56700777964554305 ) ) ;
#33180=CARTESIAN_POINT ( 'NONE',  ( -27.16883889988624290, 30.92500000273119909, -19.73931689729374028 ) ) ;
#33200=CARTESIAN_POINT ( 'NONE',  ( -27.16883889988623935, 77.32500000273120122, 19.73931689729374739 ) ) ;
#33201=CARTESIAN_POINT ( 'NONE',  ( -27.16883889988623935, 43.57500000273119412, 19.73931689729374739 ) ) ;
#33206=CARTESIAN_POINT ( 'NONE',  ( 6.277390505771533514E-15, 60.49999999999997868, 34.17252228774368916 ) ) ;
#33219=CARTESIAN_POINT ( 'NONE',  ( 10.37757302488624056, 48.52500000273117564, -31.93888565452638417 ) ) ;
#33220=CARTESIAN_POINT ( 'NONE',  ( 27.16883889988623935, 24.57500000273120477, -19.73931689729374384 ) ) ;
#33224=CYLINDRICAL_SURFACE ( 'NONE', #7299, 32.50000000000000000 ) ;
#33244=CARTESIAN_POINT ( 'NONE',  ( -10.37757302488624411, 58.97500000273119269, -31.93888565452638417 ) ) ;
#33254=CARTESIAN_POINT ( 'NONE',  ( -2.162160676586881955E-15, 24.62500000273118772, -35.31076352940723240 ) ) ;
#33257=EDGE_CURVE ( 'NONE', #927, #25651, #33738, .T. ) ;
#33261=CARTESIAN_POINT ( 'NONE',  ( -26.29305231718579350, 42.30000000546237260, -19.10302069950537884 ) ) ;
#33268=CARTESIAN_POINT ( 'NONE',  ( -33.58253175000000113, 69.12500000273118417, 0.000000000000000000 ) ) ;
#33274=CARTESIAN_POINT ( 'NONE',  ( -33.58253175000000113, 13.02500000273118985, -10.91162601494193218 ) ) ;
#33284=CARTESIAN_POINT ( 'NONE',  ( -32.50000000000000000, 32.10000000000000142, 10.55989012756946366 ) ) ;
#33288=CARTESIAN_POINT ( 'NONE',  ( -5.485892052525789174E-07, 66.99999999999998579, 32.49999999999999289 ) ) ;
#33297=CARTESIAN_POINT ( 'NONE',  ( 10.37757302488624767, 41.72500000273119980, 31.93888565452638417 ) ) ;
#33298=CARTESIAN_POINT ( 'NONE',  ( 20.75514604977248467, 6.675000002731186655, -28.56700777964554305 ) ) ;
#33299=CARTESIAN_POINT ( 'NONE',  ( 33.58253175000000113, 58.37500000273119838, -4.112674001490185761E-15 ) ) ;
#33303=CARTESIAN_POINT ( 'NONE',  ( -26.29305231718579350, 62.30000000546238681, -19.10302069950537884 ) ) ;
#33310=CARTESIAN_POINT ( 'NONE',  ( -20.75514604977248112, 35.67500000273118843, 28.56700777964554661 ) ) ;
#33314=CARTESIAN_POINT ( 'NONE',  ( 10.04305231718578817, 23.90000000546237047, -30.90933677959249337 ) ) ;
#33332=CARTESIAN_POINT ( 'NONE',  ( -10.04305231718579172, 55.59999999999999432, -30.90933677959248982 ) ) ;
#33334=CARTESIAN_POINT ( 'NONE',  ( -10.04305231718578462, 2.399999999999999467, 30.90933677959249337 ) ) ;
#33335=ORIENTED_EDGE ( 'NONE', *, *, #25184, .F. ) ;
#33339=CARTESIAN_POINT ( 'NONE',  ( 33.58253175000000113, 62.12500000273117706, -4.112674001490185761E-15 ) ) ;
#33340=CARTESIAN_POINT ( 'NONE',  ( -10.37757302488623701, 21.77500000273117919, 31.93888565452638417 ) ) ;
#33341=CARTESIAN_POINT ( 'NONE',  ( -10.37757302488624411, 10.97500000273120335, -31.93888565452638417 ) ) ;
#33346=CARTESIAN_POINT ( 'NONE',  ( 10.37757302488624767, 3.725000002731182480, 31.93888565452638417 ) ) ;
#33348=CARTESIAN_POINT ( 'NONE',  ( -20.08610463437156923, 40.30000000000001137, 27.64615127144130113 ) ) ;
#33354=CARTESIAN_POINT ( 'NONE',  ( 20.75514604977248467, 52.67500000273116711, -28.56700777964554305 ) ) ;
#33355=CARTESIAN_POINT ( 'NONE',  ( 20.08610463437157279, 59.80000000546235839, -27.64615127144129758 ) ) ;
#33360=CARTESIAN_POINT ( 'NONE',  ( 33.58253175000000823, 30.02500000273118985, 10.91162601494192863 ) ) ;
#33362=VERTEX_POINT ( 'NONE', #4237 ) ;
#33373=CARTESIAN_POINT ( 'NONE',  ( 26.29305231718578995, 55.20000000000000995, -19.10302069950538240 ) ) ;
#33380=CARTESIAN_POINT ( 'NONE',  ( 20.75514604977249178, 42.07500000273117990, 28.56700777964553950 ) ) ;
#33385=CARTESIAN_POINT ( 'NONE',  ( 20.08610463437157279, 57.29999999999999005, -27.64615127144129758 ) ) ;
#33394=EDGE_LOOP ( 'NONE', ( #15269, #17035, #20124, #25080 ) ) ;
#33395=CARTESIAN_POINT ( 'NONE',  ( -33.58253175000000113, 51.12500000273119127, 0.000000000000000000 ) ) ;
#33396=CARTESIAN_POINT ( 'NONE',  ( -10.37757302488623701, 23.77500000273117919, 31.93888565452638417 ) ) ;
#33421=CARTESIAN_POINT ( 'NONE',  ( -20.75514604977248823, 63.07500000273119412, -28.56700777964554305 ) ) ;
#33428=CARTESIAN_POINT ( 'NONE',  ( 20.08610463437157279, 77.30000000000001137, -27.64615127144129758 ) ) ;
#33429=CARTESIAN_POINT ( 'NONE',  ( -27.16883889988624290, 24.92500000273119198, -19.73931689729374028 ) ) ;
#33434=CARTESIAN_POINT ( 'NONE',  ( 10.04305231718579705, 41.10000000546236265, 30.90933677959248982 ) ) ;
#33440=CARTESIAN_POINT ( 'NONE',  ( 6.486482029760649416E-15, 71.62500000273119838, 35.31076352940723240 ) ) ;
#33446=CARTESIAN_POINT ( 'NONE',  ( 27.16883889988624290, 13.92500000273118310, 19.73931689729373673 ) ) ;
#33456=CARTESIAN_POINT ( 'NONE',  ( -20.08610463437156923, 30.30000000000000426, 27.64615127144130113 ) ) ;
#33460=CARTESIAN_POINT ( 'NONE',  ( 20.08610463437158344, 62.69999999999998863, 27.64615127144129403 ) ) ;
#33469=CARTESIAN_POINT ( 'NONE',  ( 10.37757302488624056, 42.52500000273119696, -31.93888565452638417 ) ) ;
#33470=DIRECTION ( 'NONE',  ( 0.000000000000000000, 0.000000000000000000, -1.000000000000000000 ) ) ;
#33471=CARTESIAN_POINT ( 'NONE',  ( -10.37757302488624411, 58.97500000273119269, -31.93888565452638417 ) ) ;
#33475=CARTESIAN_POINT ( 'NONE',  ( 20.08610463437157279, 61.80000000546237970, -27.64615127144129758 ) ) ;
#33484=CARTESIAN_POINT ( 'NONE',  ( 10.37757302488624767, 33.97500000273119269, 31.93888565452638417 ) ) ;
#33488=CARTESIAN_POINT ( 'NONE',  ( 6.277390505771533514E-15, 23.00000000546238610, 34.17252228774368916 ) ) ;
#33497=CARTESIAN_POINT ( 'NONE',  ( -10.37757302488624411, 66.72500000273116427, -31.93888565452638417 ) ) ;
#33507=CARTESIAN_POINT ( 'NONE',  ( -33.58253175000000113, 73.47500000273117848, 10.91162601494193929 ) ) ;
#33512=CARTESIAN_POINT ( 'NONE',  ( 33.58253175000000113, 60.22500000273119980, -10.91162601494193751 ) ) ;
#33513=CARTESIAN_POINT ( 'NONE',  ( -10.37757302488624411, 20.97500000273118559, -31.93888565452638417 ) ) ;
#33514=CARTESIAN_POINT ( 'NONE',  ( 27.16883889988623935, 12.57500000273119234, -19.73931689729374384 ) ) ;
#33519=CARTESIAN_POINT ( 'NONE',  ( 10.37757302488624056, 2.525000002731189852, -31.93888565452638417 ) ) ;
#33521=CARTESIAN_POINT ( 'NONE',  ( -2.092463501923844636E-15, 43.49999999999999289, -34.17252228774368916 ) ) ;
#33527=CARTESIAN_POINT ( 'NONE',  ( 20.75514604977248467, 54.67500000273119554, -28.56700777964554305 ) ) ;
#33533=CARTESIAN_POINT ( 'NONE',  ( -2.162160676586881955E-15, 24.62500000273118772, -35.31076352940723240 ) ) ;
#33551=EDGE_CURVE ( 'NONE', #2770, #19648, #12124, .T. ) ;
#33553=CARTESIAN_POINT ( 'NONE',  ( -10.37757302488623701, 77.52500000273120406, 31.93888565452638417 ) ) ;
#33554=CARTESIAN_POINT ( 'NONE',  ( 6.486482029760649416E-15, 45.87500000273117706, 35.31076352940723240 ) ) ;
#33560=CARTESIAN_POINT ( 'NONE',  ( -20.08610463437156923, 60.29999999999998295, 27.64615127144130113 ) ) ;
#33566=CARTESIAN_POINT ( 'NONE',  ( 27.16883889988624290, 70.17500000273118133, 19.73931689729373673 ) ) ;
#33571=CARTESIAN_POINT ( 'NONE',  ( -20.75514604977248823, 44.82500000273117990, -28.56700777964554305 ) ) ;
#33575=CARTESIAN_POINT ( 'NONE',  ( -20.08610463437157989, 6.200000005462380948, -27.64615127144129758 ) ) ;
#33596=CARTESIAN_POINT ( 'NONE',  ( 10.37757302488624056, 64.77500000273118985, -31.93888565452638417 ) ) ;
#33603=CARTESIAN_POINT ( 'NONE',  ( 32.50000000000000000, 77.09999999999998010, -10.55989012756945833 ) ) ;
#33604=CARTESIAN_POINT ( 'NONE',  ( -33.58253175000000113, 13.12500000273118772, 0.000000000000000000 ) ) ;
#33608=CARTESIAN_POINT ( 'NONE',  ( 26.29305231718578995, 41.70000000546237828, -19.10302069950538240 ) ) ;
#33612=VECTOR ( 'NONE', #16181, 1000.000000000000000 ) ;
#33614=CARTESIAN_POINT ( 'NONE',  ( 33.58253175000000823, 68.02500000273117564, 10.91162601494192863 ) ) ;
#33621=CARTESIAN_POINT ( 'NONE',  ( -27.16883889988624290, 8.925000002731206195, -19.73931689729374028 ) ) ;
#33629=CARTESIAN_POINT ( 'NONE',  ( -5.147494043133895580, 52.05125428434654822, -32.50000008688792263 ) ) ;
#33632=CARTESIAN_POINT ( 'NONE',  ( -26.29305231718578995, 30.19999999999999218, 19.10302069950538595 ) ) ;
#33636=CARTESIAN_POINT ( 'NONE',  ( 10.04305231718578817, 63.39999999999999858, -30.90933677959249337 ) ) ;
#33645=CARTESIAN_POINT ( 'NONE',  ( 23.31009017153205320, 66.99999999999998579, -23.30172593756741506 ) ) ;
#33646=CARTESIAN_POINT ( 'NONE',  ( -20.75514604977248112, 39.42500000273118843, 28.56700777964554661 ) ) ;
#33647=CARTESIAN_POINT ( 'NONE',  ( -1.137977401836464321E-14, 52.00000000000000711, 46.18802153517007270 ) ) ;
#33651=CARTESIAN_POINT ( 'NONE',  ( -2.092463501923844636E-15, 62.00000000546238255, -34.17252228774368916 ) ) ;
#33658=CARTESIAN_POINT ( 'NONE',  ( 20.75514604977248467, 32.67500000273118843, -28.56700777964554305 ) ) ;
#33663=CARTESIAN_POINT ( 'NONE',  ( -32.50000000000000000, 22.60000000546236976, 10.55989012756946366 ) ) ;
#33668=ORIENTED_EDGE ( 'NONE', *, *, #18935, .F. ) ;
#33674=CARTESIAN_POINT ( 'NONE',  ( 10.37757302488624767, 59.72500000273119269, 31.93888565452638417 ) ) ;
#33677=CARTESIAN_POINT ( 'NONE',  ( 40.00000000000000000, 52.00000000000000711, -23.09401076758505766 ) ) ;
#33684=CARTESIAN_POINT ( 'NONE',  ( 6.486482029760649416E-15, 71.87500000273116996, 35.31076352940723240 ) ) ;
#33690=CARTESIAN_POINT ( 'NONE',  ( -27.16883889988623935, 57.32500000273120833, 19.73931689729374739 ) ) ;
#33691=CARTESIAN_POINT ( 'NONE',  ( 20.75514604977248467, 16.67500000273117777, -28.56700777964554305 ) ) ;
#33692=CARTESIAN_POINT ( 'NONE',  ( -2.162160676586881955E-15, 8.875000002731189497, -35.31076352940723240 ) ) ;
#33697=CARTESIAN_POINT ( 'NONE',  ( -10.37757302488623701, 1.525000002731188964, 31.93888565452638417 ) ) ;
#33698=CARTESIAN_POINT ( 'NONE',  ( 30.82792611048020603, 52.00000000000000711, -12.22707559850320891 ) ) ;
#33699=CARTESIAN_POINT ( 'NONE',  ( 32.50000000000000000, 43.10000000000000853, -10.55989012756945833 ) ) ;
#33706=CARTESIAN_POINT ( 'NONE',  ( -33.58253175000000113, 51.37500000273119127, 0.000000000000000000 ) ) ;
#33707=CARTESIAN_POINT ( 'NONE',  ( 10.04305231718578817, 59.90000000546237402, -30.90933677959249337 ) ) ;
#33711=CARTESIAN_POINT ( 'NONE',  ( -33.58253175000000113, 27.02500000273119696, -10.91162601494193218 ) ) ;
#33716=CARTESIAN_POINT ( 'NONE',  ( -20.08610463437157989, 57.70000000000000995, -27.64615127144129758 ) ) ;
#33727=CARTESIAN_POINT ( 'NONE',  ( -10.04305231718578462, 14.40000000000000924, 30.90933677959249337 ) ) ;
#33734=CARTESIAN_POINT ( 'NONE',  ( 33.58253175000000113, 34.47500000273119980, -10.91162601494193751 ) ) ;
#33738=CIRCLE ( 'NONE', #11794, 32.50000000000000000 ) ;
#33741=CARTESIAN_POINT ( 'NONE',  ( -2.092463501923844636E-15, 61.50000000000000000, -34.17252228774368916 ) ) ;
#33745=CARTESIAN_POINT ( 'NONE',  ( -27.16883889988623935, 71.57500000273118701, 19.73931689729374739 ) ) ;
#33747=VECTOR ( 'NONE', #19782, 1000.000000000000000 ) ;
#33752=CARTESIAN_POINT ( 'NONE',  ( -33.58253175000000113, 41.22500000273118559, 10.91162601494193929 ) ) ;
#33754=EDGE_CURVE ( 'NONE', #18447, #1729, #13156, .T. ) ;
#33758=CARTESIAN_POINT ( 'NONE',  ( 32.50000000000000711, 1.400000005462371799, 10.55989012756945122 ) ) ;
#33777=CARTESIAN_POINT ( 'NONE',  ( -33.58253175000000113, 65.27500000273117564, -10.91162601494193218 ) ) ;
#33781=DIRECTION ( 'NONE',  ( 0.000000000000000000, 1.000000000000000000, 0.000000000000000000 ) ) ;
#33783=CARTESIAN_POINT ( 'NONE',  ( -32.50000000000000000, 77.90000000000001990, -10.55989012756945478 ) ) ;
#33784=CARTESIAN_POINT ( 'NONE',  ( -2.162160676586881955E-15, 16.62500000273120548, -35.31076352940723240 ) ) ;
#33789=CARTESIAN_POINT ( 'NONE',  ( -32.50000000000000000, 34.50000000546236834, 0.000000000000000000 ) ) ;
#33794=CARTESIAN_POINT ( 'NONE',  ( 10.37757302488624767, 61.72500000273119269, 31.93888565452638417 ) ) ;
#33799=CARTESIAN_POINT ( 'NONE',  ( -2.162160676586881955E-15, 8.625000002731180615, -35.31076352940723240 ) ) ;
#33802=AXIS2_PLACEMENT_3D ( 'NONE', #6502, #833, #8899 ) ;
#33807=CARTESIAN_POINT ( 'NONE',  ( -10.04305231718579172, 52.10000000546237686, -30.90933677959248982 ) ) ;
#33810=CARTESIAN_POINT ( 'NONE',  ( -20.08610463437157989, 31.69999999999998508, -27.64615127144129758 ) ) ;
#33814=CARTESIAN_POINT ( 'NONE',  ( -33.29860495311159951, 66.99999999999998579, 1.751800823569703791 ) ) ;
#33819=CARTESIAN_POINT ( 'NONE',  ( 29.96643421716999356, 66.99999999999997158, -13.17858490638464986 ) ) ;
#33820=CARTESIAN_POINT ( 'NONE',  ( -10.37757302488623701, 33.52500000273118985, 31.93888565452638417 ) ) ;
#33821=CARTESIAN_POINT ( 'NONE',  ( 2.205017735002230837E-13, 57.49999999999998579, -32.50000000000000000 ) ) ;
#33825=CARTESIAN_POINT ( 'NONE',  ( 26.29305231718578995, 53.70000000546236407, -19.10302069950538240 ) ) ;
#33832=CARTESIAN_POINT ( 'NONE',  ( -10.37757302488624411, 36.97500000273119980, -31.93888565452638417 ) ) ;
#33836=CARTESIAN_POINT ( 'NONE',  ( 10.04305231718578817, 25.90000000546237402, -30.90933677959249337 ) ) ;
#33848=CARTESIAN_POINT ( 'NONE',  ( 33.58253175000000113, 64.22500000273117848, -10.91162601494193574 ) ) ;
#33857=VECTOR ( 'NONE', #25765, 1000.000000000000114 ) ;
#33858=CARTESIAN_POINT ( 'NONE',  ( 6.486482029760649416E-15, 77.87500000273118417, 35.31076352940723240 ) ) ;
#33863=CARTESIAN_POINT ( 'NONE',  ( -20.75514604977248112, 51.42500000273118133, 28.56700777964554661 ) ) ;
#33864=CARTESIAN_POINT ( 'NONE',  ( 10.37757302488624767, 19.97500000273118204, 31.93888565452638417 ) ) ;
#33865=CARTESIAN_POINT ( 'NONE',  ( -20.75514604977248112, 3.675000002731193316, 28.56700777964554661 ) ) ;
#33869=CARTESIAN_POINT ( 'NONE',  ( 20.75514604977249178, 5.825000002731183457, 28.56700777964553950 ) ) ;
#33875=CARTESIAN_POINT ( 'NONE',  ( -2.162160676586881955E-15, 52.87500000273119838, -35.31076352940723240 ) ) ;
#33880=CARTESIAN_POINT ( 'NONE',  ( -2.162160676586881955E-15, 22.62500000273119127, -35.31076352940723240 ) ) ;
#33896=CARTESIAN_POINT ( 'NONE',  ( 10.04305231718578817, 17.40000000000001279, -30.90933677959249337 ) ) ;
#33902=CARTESIAN_POINT ( 'NONE',  ( 6.486482029760649416E-15, 73.62500000273118417, 35.31076352940723240 ) ) ;
#33903=CARTESIAN_POINT ( 'NONE',  ( 6.486482029760649416E-15, 33.87500000273118417, 35.31076352940723240 ) ) ;
#33905=CARTESIAN_POINT ( 'NONE',  ( -2.165007332552593587E-13, 52.50000000000000711, 32.50000000000000000 ) ) ;
#33910=CARTESIAN_POINT ( 'NONE',  ( -10.04305231718578462, 58.39999999999999147, 30.90933677959249337 ) ) ;
#33915=CARTESIAN_POINT ( 'NONE',  ( -27.16883889988624290, 73.17500000273118133, -19.73931689729374028 ) ) ;
#33920=CARTESIAN_POINT ( 'NONE',  ( -2.162160676586881955E-15, 44.62500000273119838, -35.31076352940723240 ) ) ;
#33924=CARTESIAN_POINT ( 'NONE',  ( -20.08610463437157989, 2.200000005462375618, -27.64615127144129758 ) ) ;
#33943=CARTESIAN_POINT ( 'NONE',  ( -27.16883889988624290, 53.17500000273118843, -19.73931689729374028 ) ) ;
#33948=CARTESIAN_POINT ( 'NONE',  ( 20.08610463437157279, 79.30000000000001137, -27.64615127144129758 ) ) ;
#33949=CARTESIAN_POINT ( 'NONE',  ( 33.58253175000000823, 16.02500000273119340, 10.91162601494192863 ) ) ;
#33953=CARTESIAN_POINT ( 'NONE',  ( 26.29305231718579350, 35.30000000546239391, 19.10302069950537529 ) ) ;
#33958=CARTESIAN_POINT ( 'NONE',  ( 10.37757302488624056, 62.52500000273118985, -31.93888565452638417 ) ) ;
#33963=VERTEX_POINT ( 'NONE', #18411 ) ;
#33964=CARTESIAN_POINT ( 'NONE',  ( 33.58253175000000113, 2.225000002731181592, -10.91162601494193751 ) ) ;
#33974=CARTESIAN_POINT ( 'NONE',  ( -32.50000000000000000, 28.10000000000001208, 10.55989012756946366 ) ) ;
#33987=CARTESIAN_POINT ( 'NONE',  ( 6.486482029760649416E-15, 35.62500000273119127, 35.31076352940723240 ) ) ;
#33988=CARTESIAN_POINT ( 'NONE',  ( -32.50000000000000000, 64.40000000546238823, -10.55989012756945300 ) ) ;
ENDSEC;
END-ISO-10303-21;
